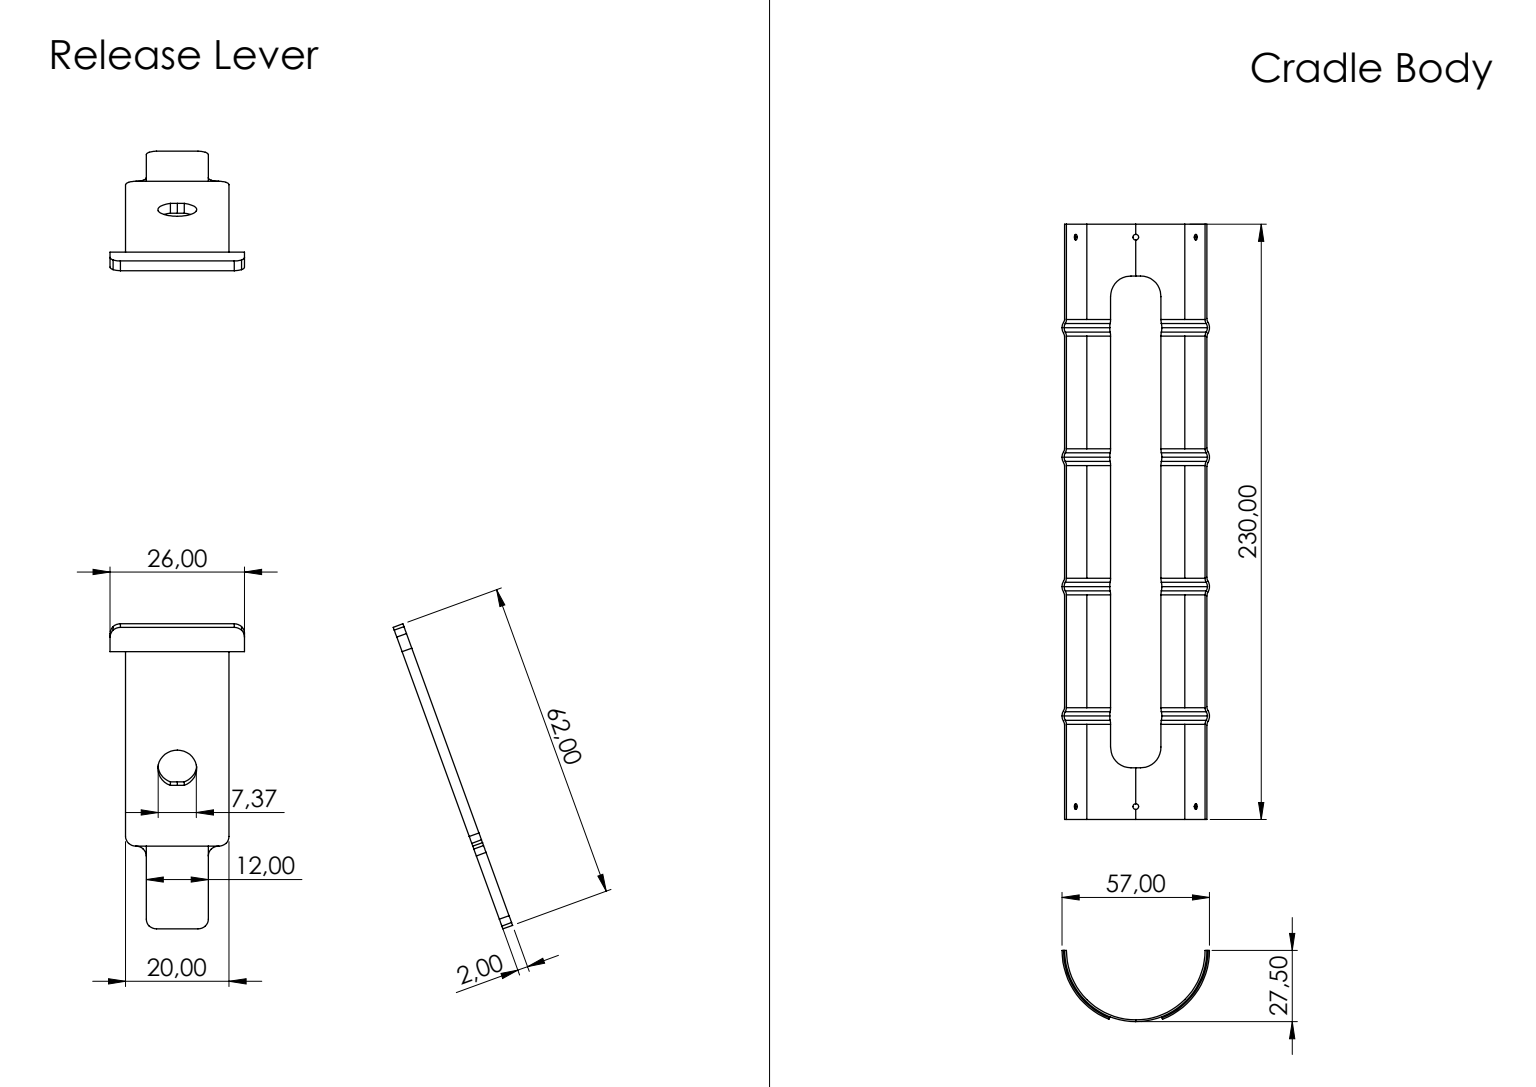
ISO-10303-21;
HEADER;
FILE_DESCRIPTION (('STEP AP214'),
    '1' );
FILE_NAME ('Cradle Body.step',
    '2026-10-06T09:00:30',
    ( '' ),
    ( '' ),
    'SwSTEP 2.0',
    'SolidWorks 2020',
    '' );
FILE_SCHEMA (( 'AUTOMOTIVE_DESIGN' ));
ENDSEC;

DATA;
#3=CARTESIAN_POINT ( 'NONE',  ( 27.50000000000000000, -6.735334946019999940E-15, 115.0000000000000000 ) ) ;
#7=B_SPLINE_CURVE_WITH_KNOTS ( 'NONE', 5,
 ( #8666, #18262, #27873, #6319, #23164, #13557 ),
 .UNSPECIFIED., .F., .F.,
 ( 6, 6 ),
 ( -2.319814965009999952, 0.000000000000000000 ),
 .UNSPECIFIED. ) ;
#21=ORIENTED_EDGE ( 'NONE', *, *, #30426, .T. ) ;
#35=AXIS2_PLACEMENT_3D ( 'NONE', #27512, #5959, #1254 ) ;
#45=ORIENTED_EDGE ( 'NONE', *, *, #3237, .T. ) ;
#75=CARTESIAN_POINT ( 'NONE',  ( 0.09701118263791908003, -27.50000000070000894, 6.100000000000011191 ) ) ;
#76=ORIENTED_EDGE ( 'NONE', *, *, #19659, .F. ) ;
#80=EDGE_CURVE ( 'NONE', #20682, #22430, #3324, .T. ) ;
#82=CARTESIAN_POINT ( 'NONE',  ( 7.105427357599999217E-15, 3.552713678799999608E-15, 43.21714158840000408 ) ) ;
#85=EDGE_LOOP ( 'NONE', ( #21526, #26943, #30310, #22481 ) ) ;
#87=CARTESIAN_POINT ( 'NONE',  ( 27.69999999930000101, -3.392159599989999961E-15, 90.00000000000000000 ) ) ;
#106=EDGE_CURVE ( 'NONE', #11838, #4649, #28678, .T. ) ;
#109=ORIENTED_EDGE ( 'NONE', *, *, #22749, .F. ) ;
#114=AXIS2_PLACEMENT_3D ( 'NONE', #11940, #28625, #12094 ) ;
#115=CARTESIAN_POINT ( 'NONE',  ( -3.552713678799999608E-15, 0.000000000000000000, 193.2171415880000040 ) ) ;
#128=DIRECTION ( 'NONE',  ( -0.000000000000000000, -0.000000000000000000, -1.000000000000000000 ) ) ;
#137=ORIENTED_EDGE ( 'NONE', *, *, #11511, .F. ) ;
#149=CARTESIAN_POINT ( 'NONE',  ( 0.4908581387334869928, -27.49541710664063032, 225.9948832293035537 ) ) ;
#160=ORIENTED_EDGE ( 'NONE', *, *, #26147, .F. ) ;
#162=FACE_BOUND ( 'NONE', #6310, .T. ) ;
#166=ORIENTED_EDGE ( 'NONE', *, *, #29617, .T. ) ;
#182=ORIENTED_EDGE ( 'NONE', *, *, #19559, .F. ) ;
#186=EDGE_CURVE ( 'NONE', #24695, #19740, #19204, .T. ) ;
#189=LINE ( 'NONE', #19380, #24692 ) ;
#190=CARTESIAN_POINT ( 'NONE',  ( 8.566424601805415762, -26.13212873426111216, 23.30748548239859019 ) ) ;
#192=AXIS2_PLACEMENT_3D ( 'NONE', #23801, #30571, #26003 ) ;
#202=EDGE_LOOP ( 'NONE', ( #3283, #15747, #28522, #14669, #12113 ) ) ;
#208=VECTOR ( 'NONE', #27934, 1000.000000000000114 ) ;
#210=CIRCLE ( 'NONE', #706, 27.69999999999999929 ) ;
#213=ORIENTED_EDGE ( 'NONE', *, *, #13656, .T. ) ;
#220=ADVANCED_FACE ( 'NONE', ( #19519 ), #21819, .T. ) ;
#224=EDGE_CURVE ( 'NONE', #17932, #4565, #12425, .T. ) ;
#228=CARTESIAN_POINT ( 'NONE',  ( 26.93395403039999891, -3.298349123909999533E-15, 87.75675929330000713 ) ) ;
#231=CARTESIAN_POINT ( 'NONE',  ( 22.70032920257776254, -14.24644155109503885, 5.491373161944450132 ) ) ;
#237=AXIS2_PLACEMENT_3D ( 'NONE', #28809, #7419, #7570 ) ;
#240=AXIS2_PLACEMENT_3D ( 'NONE', #28736, #7186, #4980 ) ;
#241=AXIS2_PLACEMENT_3D ( 'NONE', #12449, #26774, #973 ) ;
#243=AXIS2_PLACEMENT_3D ( 'NONE', #30286, #20689, #17993 ) ;
#255=EDGE_CURVE ( 'NONE', #7386, #15620, #13185, .T. ) ;
#264=DIRECTION ( 'NONE',  ( 0.000000000000000000, 0.000000000000000000, -1.000000000000000000 ) ) ;
#271=DIRECTION ( 'NONE',  ( 0.000000000000000000, 0.000000000000000000, 1.000000000000000000 ) ) ;
#276=CARTESIAN_POINT ( 'NONE',  ( 0.9565336475350260104, -27.48338672371320612, 4.451904520592202097 ) ) ;
#281=CARTESIAN_POINT ( 'NONE',  ( 8.903108651239925564, -22.82508830966962421, 140.0000000000000000 ) ) ;
#290=ORIENTED_EDGE ( 'NONE', *, *, #7961, .T. ) ;
#300=DIRECTION ( 'NONE',  ( -1.224606353819999829E-16, -1.000000000000000000, 0.000000000000000000 ) ) ;
#304=DIRECTION ( 'NONE',  ( 0.000000000000000000, 0.000000000000000000, 1.000000000000000000 ) ) ;
#312=CARTESIAN_POINT ( 'NONE',  ( 1.087768546295719840, -27.47890868157812605, 225.2179249496743978 ) ) ;
#314=CARTESIAN_POINT ( 'NONE',  ( 8.903108651239925564, -22.82508830966962421, 40.00000000000000000 ) ) ;
#317=DIRECTION ( 'NONE',  ( 0.9316362575375356503, 0.3633921898465274913, 0.000000000000000000 ) ) ;
#324=FACE_OUTER_BOUND ( 'NONE', #14055, .T. ) ;
#332=ORIENTED_EDGE ( 'NONE', *, *, #29953, .F. ) ;
#342=CARTESIAN_POINT ( 'NONE',  ( -23.20948082139999968, -13.40000000000000036, 6.099999999630000502 ) ) ;
#351=CARTESIAN_POINT ( 'NONE',  ( 8.414407093329970166, -26.18160851622837981, 23.09437632025412412 ) ) ;
#369=ORIENTED_EDGE ( 'NONE', *, *, #12352, .F. ) ;
#380=EDGE_CURVE ( 'NONE', #18294, #17040, #28347, .T. ) ;
#381=AXIS2_PLACEMENT_3D ( 'NONE', #29649, #27284, #22722 ) ;
#385=DIRECTION ( 'NONE',  ( 0.000000000000000000, 0.000000000000000000, 1.000000000000000000 ) ) ;
#387=CARTESIAN_POINT ( 'NONE',  ( 7.105427357599999217E-15, 3.552713678799999608E-15, 143.6055512749999821 ) ) ;
#390=CARTESIAN_POINT ( 'NONE',  ( 10.35667741062603397, -26.55163333981976592, 190.0000000000000000 ) ) ;
#399=DIRECTION ( 'NONE',  ( 0.000000000000000000, 0.000000000000000000, 1.000000000000000000 ) ) ;
#400=ORIENTED_EDGE ( 'NONE', *, *, #20390, .F. ) ;
#405=CIRCLE ( 'NONE', #17950, 27.23548387080000310 ) ;
#407=FACE_OUTER_BOUND ( 'NONE', #9123, .T. ) ;
#420=AXIS2_PLACEMENT_3D ( 'NONE', #11851, #7126, #19088 ) ;
#422=CARTESIAN_POINT ( 'NONE',  ( -27.92857142909999979, 3.420150602519999655E-15, 92.06031501479999690 ) ) ;
#427=CIRCLE ( 'NONE', #27022, 27.23548387080000310 ) ;
#428=DIRECTION ( 'NONE',  ( 0.3633921898465272138, -0.9316362575375356503, 0.000000000000000000 ) ) ;
#432=AXIS2_PLACEMENT_3D ( 'NONE', #11352, #25679, #6931 ) ;
#439=CARTESIAN_POINT ( 'NONE',  ( -24.33346004068414459, -12.81155130651161045, 5.286751411345756324 ) ) ;
#449=ORIENTED_EDGE ( 'NONE', *, *, #3492, .F. ) ;
#462=ORIENTED_EDGE ( 'NONE', *, *, #21169, .F. ) ;
#470=CARTESIAN_POINT ( 'NONE',  ( -3.907985046680000082E-14, -26.80000000000000071, 6.099999999630000502 ) ) ;
#471=DIRECTION ( 'NONE',  ( 1.000000000000000000, 0.000000000000000000, 0.000000000000000000 ) ) ;
#473=CARTESIAN_POINT ( 'NONE',  ( -27.50000000000000000, 3.367667473009999970E-15, 36.39444872359999295 ) ) ;
#474=CARTESIAN_POINT ( 'NONE',  ( 0.6479069288420113981, -26.79235980062891542, 224.0901877813894032 ) ) ;
#485=ORIENTED_EDGE ( 'NONE', *, *, #26372, .T. ) ;
#486=AXIS2_PLACEMENT_3D ( 'NONE', #21935, #385, #9970 ) ;
#489=ORIENTED_EDGE ( 'NONE', *, *, #26242, .T. ) ;
#498=DIRECTION ( 'NONE',  ( -0.7071067811865475727, -0.7071067811865475727, 0.000000000000000000 ) ) ;
#504=ADVANCED_FACE ( 'NONE', ( #24355, #2797 ), #16952, .T. ) ;
#505=CARTESIAN_POINT ( 'NONE',  ( 10.14902473058287491, -26.01926976374856082, 187.9396849849999853 ) ) ;
#513=ORIENTED_EDGE ( 'NONE', *, *, #26739, .T. ) ;
#515=CARTESIAN_POINT ( 'NONE',  ( -10.35667741062608371, -26.55163333981974816, 190.0000000000000000 ) ) ;
#521=DIRECTION ( 'NONE',  ( 1.000000000000000000, 0.000000000000000000, 0.000000000000000000 ) ) ;
#524=ORIENTED_EDGE ( 'NONE', *, *, #26123, .T. ) ;
#530=FACE_OUTER_BOUND ( 'NONE', #26990, .T. ) ;
#538=ORIENTED_EDGE ( 'NONE', *, *, #20624, .T. ) ;
#546=LINE ( 'NONE', #17194, #5634 ) ;
#547=DIRECTION ( 'NONE',  ( 0.000000000000000000, 0.000000000000000000, -1.000000000000000000 ) ) ;
#559=ORIENTED_EDGE ( 'NONE', *, *, #5058, .T. ) ;
#564=DIRECTION ( 'NONE',  ( 1.000000000000000000, 0.000000000000000000, 0.000000000000000000 ) ) ;
#568=DIRECTION ( 'NONE',  ( 1.000000000000000000, -1.224606353819999582E-16, 0.000000000000000000 ) ) ;
#569=AXIS2_PLACEMENT_3D ( 'NONE', #17547, #27158, #15193 ) ;
#570=CARTESIAN_POINT ( 'NONE',  ( -3.552713678799999608E-15, -26.80000000000000071, 0.000000000000000000 ) ) ;
#571=CARTESIAN_POINT ( 'NONE',  ( -23.92402432625451070, -13.56054118811422882, 3.912293197164086855 ) ) ;
#577=ORIENTED_EDGE ( 'NONE', *, *, #30008, .F. ) ;
#580=CARTESIAN_POINT ( 'NONE',  ( 24.49999999589999788, -3.000285566359999846E-15, 90.00000000000000000 ) ) ;
#583=CARTESIAN_POINT ( 'NONE',  ( 26.93395386830000149, -3.298349104060000254E-15, 142.2432411360000231 ) ) ;
#589=FACE_OUTER_BOUND ( 'NONE', #26163, .T. ) ;
#591=CARTESIAN_POINT ( 'NONE',  ( -22.29514036694591184, -14.89751301532327155, 93.21714158846667431 ) ) ;
#607=DIRECTION ( 'NONE',  ( 1.224606353819999829E-16, 1.000000000000000000, 0.000000000000000000 ) ) ;
#619=EDGE_CURVE ( 'NONE', #11656, #7142, #9529, .T. ) ;
#625=CARTESIAN_POINT ( 'NONE',  ( -26.84464183999999776, 3.287411896330000120E-15, 142.5624961750000068 ) ) ;
#637=ORIENTED_EDGE ( 'NONE', *, *, #4986, .T. ) ;
#640=ORIENTED_EDGE ( 'NONE', *, *, #8309, .F. ) ;
#660=CARTESIAN_POINT ( 'NONE',  ( 24.34663841809999951, -12.78636765230000094, 5.000000000000000000 ) ) ;
#667=DIRECTION ( 'NONE',  ( 0.3090169943750400994, -0.9510565162951234441, 0.000000000000000000 ) ) ;
#668=EDGE_CURVE ( 'NONE', #10071, #13694, #28108, .T. ) ;
#675=CARTESIAN_POINT ( 'NONE',  ( 27.50000000000000000, -1.044349611129999949E-13, 0.000000000000000000 ) ) ;
#677=EDGE_CURVE ( 'NONE', #10071, #14251, #16593, .T. ) ;
#679=DIRECTION ( 'NONE',  ( 0.9316362575375356503, 0.3633921898465274913, 0.000000000000000000 ) ) ;
#680=ORIENTED_EDGE ( 'NONE', *, *, #23014, .F. ) ;
#682=DIRECTION ( 'NONE',  ( 0.9316362575375356503, 0.3633921898465274913, 0.000000000000000000 ) ) ;
#684=CARTESIAN_POINT ( 'NONE',  ( 0.000000000000000000, 0.000000000000000000, 92.06031501460000754 ) ) ;
#685=CIRCLE ( 'NONE', #15728, 3.200000000000000178 ) ;
#688=MANIFOLD_SOLID_BREP ( 'Stock-MAS-156-1', #17562 ) ;
#691=TOROIDAL_SURFACE ( 'NONE', #8176, 29.80000000000000071, 3.000000000000000000 ) ;
#694=CARTESIAN_POINT ( 'NONE',  ( -0.2897532859572976571, -27.49881094958763939, 6.071390044457605661 ) ) ;
#695=CARTESIAN_POINT ( 'NONE',  ( 23.26185891380331583, -14.66761890373620503, 225.2867514118632357 ) ) ;
#706=AXIS2_PLACEMENT_3D ( 'NONE', #14476, #7537, #17129 ) ;
#708=CIRCLE ( 'NONE', #23295, 3.000000000000001332 ) ;
#709=CARTESIAN_POINT ( 'NONE',  ( 23.81569860410000317, -13.75000000000000000, 6.099999999630000502 ) ) ;
#717=LINE ( 'NONE', #17373, #10923 ) ;
#722=ORIENTED_EDGE ( 'NONE', *, *, #2189, .T. ) ;
#729=CIRCLE ( 'NONE', #20825, 27.50000000000000000 ) ;
#731=VECTOR ( 'NONE', #13088, 1000.000000000000114 ) ;
#733=CARTESIAN_POINT ( 'NONE',  ( 26.80000000069999899, -3.281945028320000125E-15, 142.8898184869999852 ) ) ;
#734=CARTESIAN_POINT ( 'NONE',  ( -5.851800771450323957, -26.15706768910720825, 208.9785434308453489 ) ) ;
#741=CARTESIAN_POINT ( 'NONE',  ( -7.833397470852288436, -25.63019328476619307, 22.68384840406914549 ) ) ;
#752=EDGE_CURVE ( 'NONE', #26248, #11846, #25282, .T. ) ;
#758=DIRECTION ( 'NONE',  ( 1.224606353819999829E-16, 1.000000000000000000, 0.000000000000000000 ) ) ;
#768=CARTESIAN_POINT ( 'NONE',  ( 20.19076655603537418, -17.71015691556361205, 86.78285841154168168 ) ) ;
#770=DIRECTION ( 'NONE',  ( 0.000000000000000000, 0.000000000000000000, 1.000000000000000000 ) ) ;
#774=CARTESIAN_POINT ( 'NONE',  ( 9.339631244007776445, -25.12005762863061165, 204.5931320852415354 ) ) ;
#783=DIRECTION ( 'NONE',  ( 0.7071067811865475727, 0.7071067811865475727, 0.000000000000000000 ) ) ;
#798=CYLINDRICAL_SURFACE ( 'NONE', #20779, 26.80000000000002203 ) ;
#799=CARTESIAN_POINT ( 'NONE',  ( -27.50000000000000000, 1.776356839399999804E-15, 43.60555127550000520 ) ) ;
#800=DIRECTION ( 'NONE',  ( 0.000000000000000000, 0.000000000000000000, 1.000000000000000000 ) ) ;
#807=CARTESIAN_POINT ( 'NONE',  ( 11.08346179031908640, -28.41490585489484033, 193.6055512750000105 ) ) ;
#813=CARTESIAN_POINT ( 'NONE',  ( -27.54391552379999908, 3.373045395949999841E-15, 92.95625301640001226 ) ) ;
#819=CARTESIAN_POINT ( 'NONE',  ( 0.000000000000000000, 0.000000000000000000, 90.00000000000000000 ) ) ;
#821=ORIENTED_EDGE ( 'NONE', *, *, #27749, .F. ) ;
#822=CARTESIAN_POINT ( 'NONE',  ( -0.8355101799141004815, -26.78702284090145014, 4.280685865825344827 ) ) ;
#839=CARTESIAN_POINT ( 'NONE',  ( 0.000000000000000000, -17.25771824150000100, 5.000000000000000000 ) ) ;
#840=EDGE_CURVE ( 'NONE', #23934, #21744, #20728, .T. ) ;
#842=CARTESIAN_POINT ( 'NONE',  ( 23.74292845531203966, -13.87604159492686939, 226.1000000000000512 ) ) ;
#846=EDGE_CURVE ( 'NONE', #15698, #27653, #3362, .T. ) ;
#859=SHAPE_REPRESENTATION_RELATIONSHIP ( 'NONE' , 'NONE' ,  #19621, #20057 ) ;
#863=ORIENTED_EDGE ( 'NONE', *, *, #7156, .T. ) ;
#871=ORIENTED_EDGE ( 'NONE', *, *, #27753, .F. ) ;
#873=CARTESIAN_POINT ( 'NONE',  ( 1.100000000000000089, -26.77741585740000119, 5.000000000000000000 ) ) ;
#875=ORIENTED_EDGE ( 'NONE', *, *, #15893, .F. ) ;
#876=CARTESIAN_POINT ( 'NONE',  ( 11.45957740435851235, -24.29669185712473478, 36.78285841129288514 ) ) ;
#885=CARTESIAN_POINT ( 'NONE',  ( 27.76135144349999706, -3.399672736829999707E-15, 142.3385858900000187 ) ) ;
#886=EDGE_CURVE ( 'NONE', #22309, #15300, #28972, .T. ) ;
#891=AXIS2_PLACEMENT_3D ( 'NONE', #15373, #6397, #3885 ) ;
#892=CARTESIAN_POINT ( 'NONE',  ( -19.36389667587701524, -18.53702679572193546, 93.21714158842225117 ) ) ;
#902=VERTEX_POINT ( 'NONE', #27140 ) ;
#903=CIRCLE ( 'NONE', #21011, 2.999999999999999556 ) ;
#906=ORIENTED_EDGE ( 'NONE', *, *, #846, .F. ) ;
#911=CIRCLE ( 'NONE', #3909, 4.000000000000001776 ) ;
#922=CARTESIAN_POINT ( 'NONE',  ( -27.92857142820000149, 1.776356839399999804E-15, 187.9396849849999853 ) ) ;
#927=CARTESIAN_POINT ( 'NONE',  ( 8.158046243928268382, -25.52871334855630536, 206.9076631228209635 ) ) ;
#930=CARTESIAN_POINT ( 'NONE',  ( 24.05715877135684622, -13.32261293554750914, 225.9948832293248415 ) ) ;
#942=ORIENTED_EDGE ( 'NONE', *, *, #4712, .F. ) ;
#947=EDGE_CURVE ( 'NONE', #18243, #19781, #29652, .T. ) ;
#958=VECTOR ( 'NONE', #5157, 1000.000000000000114 ) ;
#959=CARTESIAN_POINT ( 'NONE',  ( 0.000000000000000000, 0.000000000000000000, 115.0000000000000000 ) ) ;
#969=DIRECTION ( 'NONE',  ( 1.000000000000000000, 0.000000000000000000, 0.000000000000000000 ) ) ;
#970=LINE ( 'NONE', #17624, #2207 ) ;
#971=ORIENTED_EDGE ( 'NONE', *, *, #25154, .T. ) ;
#973=DIRECTION ( 'NONE',  ( -0.5000000000001898481, -0.8660254037843291286, 0.000000000000000000 ) ) ;
#975=CARTESIAN_POINT ( 'NONE',  ( -4.182178350032519809, -27.18131967880235322, 20.25455995680620447 ) ) ;
#976=ORIENTED_EDGE ( 'NONE', *, *, #14186, .T. ) ;
#981=EDGE_CURVE ( 'NONE', #18243, #12035, #20262, .T. ) ;
#988=CARTESIAN_POINT ( 'NONE',  ( -27.50000000000000000, 3.367667473009999970E-15, 186.3944487260000074 ) ) ;
#998=VECTOR ( 'NONE', #23561, 1000.000000000000000 ) ;
#999=AXIS2_PLACEMENT_3D ( 'NONE', #22838, #679, #10268 ) ;
#1000=CARTESIAN_POINT ( 'NONE',  ( 24.34660549313293032, -12.78643034496977116, 224.8543268302984188 ) ) ;
#1003=CARTESIAN_POINT ( 'NONE',  ( 23.76736455380283530, -13.83371703085023086, 223.8999999999988688 ) ) ;
#1004=ORIENTED_EDGE ( 'NONE', *, *, #677, .F. ) ;
#1025=CARTESIAN_POINT ( 'NONE',  ( 14.94562240850000023, -8.628859120750000500, 225.0000000000000000 ) ) ;
#1029=ORIENTED_EDGE ( 'NONE', *, *, #5957, .T. ) ;
#1031=CARTESIAN_POINT ( 'NONE',  ( -22.77466902118896996, -14.12660345815406338, 4.296357262948782285 ) ) ;
#1038=EDGE_LOOP ( 'NONE', ( #25052, #15396, #23007, #6576 ) ) ;
#1042=FACE_OUTER_BOUND ( 'NONE', #3125, .T. ) ;
#1048=ORIENTED_EDGE ( 'NONE', *, *, #17146, .F. ) ;
#1057=CARTESIAN_POINT ( 'NONE',  ( -23.73992238019999945, -12.43607998449999918, 225.0000000000000000 ) ) ;
#1067=CARTESIAN_POINT ( 'NONE',  ( 23.62133197435833409, -12.66014020633680914, 4.296357262547505940 ) ) ;
#1069=B_SPLINE_CURVE_WITH_KNOTS ( 'NONE', 3,
 ( #24794, #9698, #21667, #19302, #28895, #7344, #26539, #4979, #14590, #24178, #2618, #19455, #12210, #21822 ),
 .UNSPECIFIED., .F., .F.,
 ( 4, 2, 2, 2, 2, 2, 4 ),
 ( 0.000000000000000000, 0.2500000000000449640, 0.3750000000000674460, 0.4375000000000606182, 0.5000000000000538458, 0.7500000000000269784, 1.000000000000000000 ),
 .UNSPECIFIED. ) ;
#1070=CARTESIAN_POINT ( 'NONE',  ( -1.100000000000000089, -27.47799119300000115, 225.0000000000000000 ) ) ;
#1074=CARTESIAN_POINT ( 'NONE',  ( 7.662090775718879421, -25.68204763724676454, 207.5103208889252357 ) ) ;
#1077=CARTESIAN_POINT ( 'NONE',  ( 6.496986506900683800, -26.00150201275823392, 21.45239876629313258 ) ) ;
#1083=ORIENTED_EDGE ( 'NONE', *, *, #8304, .F. ) ;
#1088=EDGE_LOOP ( 'NONE', ( #13311, #8137, #3315, #26948, #18723, #26281, #19667, #6923, #6456, #7311, #3860, #7841, #18721, #26251, #1988, #26660, #13386, #29370, #11303, #12417, #30625, #13343, #13248, #22269, #29067, #21456, #29439, #26048, #28817, #4264, #9391, #19279, #17779, #17940, #28601, #166, #332, #23931, #19123, #1813, #6184, #27951, #18968, #5521 ) ) ;
#1092=CARTESIAN_POINT ( 'NONE',  ( -7.453090060300354480, -2.907137518772246576, 27.99999999999999645 ) ) ;
#1096=CARTESIAN_POINT ( 'NONE',  ( -7.453090060300356257, -2.907137518772246576, 20.00000000000000000 ) ) ;
#1110=CARTESIAN_POINT ( 'NONE',  ( 0.000000000000000000, 0.000000000000000000, 36.39444872359999295 ) ) ;
#1115=DIRECTION ( 'NONE',  ( 0.000000000000000000, 0.000000000000000000, 1.000000000000000000 ) ) ;
#1117=CARTESIAN_POINT ( 'NONE',  ( -22.63992238021892334, -14.34133587286723888, 224.9035646515725659 ) ) ;
#1119=ORIENTED_EDGE ( 'NONE', *, *, #21500, .T. ) ;
#1120=CARTESIAN_POINT ( 'NONE',  ( -0.1474957663552681764, -26.80000000000001492, 3.899999999999999911 ) ) ;
#1121=ORIENTED_EDGE ( 'NONE', *, *, #17384, .F. ) ;
#1131=CARTESIAN_POINT ( 'NONE',  ( 9.797681423453981964, -25.69548940455785413, 203.8387348960827694 ) ) ;
#1149=ORIENTED_EDGE ( 'NONE', *, *, #12119, .F. ) ;
#1158=CARTESIAN_POINT ( 'NONE',  ( 24.29812717139177636, -12.87956648213236832, 5.490554142100076085 ) ) ;
#1161=CARTESIAN_POINT ( 'NONE',  ( -8.903108651239966420, -22.82508830966961000, 140.0000000000000000 ) ) ;
#1163=EDGE_CURVE ( 'NONE', #16579, #13261, #16538, .T. ) ;
#1167=EDGE_CURVE ( 'NONE', #15899, #25472, #18720, .T. ) ;
#1168=B_SPLINE_CURVE_WITH_KNOTS ( 'NONE', 3,
 ( #26996, #12366, #24485, #2922, #12515, #29350, #5435, #3071, #734, #10325, #29505, #7942, #17542, #4831, #22437, #15497, #3534, #22594, #3375, #12981, #25101, #3227, #13445, #8397 ),
 .UNSPECIFIED., .F., .F.,
 ( 4, 2, 2, 2, 2, 2, 2, 2, 2, 2, 2, 4 ),
 ( 0.000000000000000000, 0.001577043753785914524, 0.002365565630678863329, 0.003154087507571812134, 0.004731131261357737934, 0.005519653138250699316, 0.006308175015143660698, 0.007885218768929582595, 0.009462262522715505358, 0.01025078439960847021, 0.01103930627650143333, 0.01261635003028735783 ),
 .UNSPECIFIED. ) ;
#1180=ORIENTED_EDGE ( 'NONE', *, *, #1838, .T. ) ;
#1182=CARTESIAN_POINT ( 'NONE',  ( -22.87891075612136760, -13.95728375031006685, 4.090187774257245223 ) ) ;
#1189=CARTESIAN_POINT ( 'NONE',  ( 22.63996212555145249, -14.34127312894895923, 224.8540320937674437 ) ) ;
#1206=EDGE_LOOP ( 'NONE', ( #7039, #213, #29911, #1121, #16764, #16573 ) ) ;
#1226=CARTESIAN_POINT ( 'NONE',  ( -9.993285220779425160, -25.61999708228226069, 136.3944487260000074 ) ) ;
#1231=CARTESIAN_POINT ( 'NONE',  ( 9.484767271962898150, -25.06561782275612771, 204.0863404859320553 ) ) ;
#1233=CARTESIAN_POINT ( 'NONE',  ( -24.90462872294775920, -9.900530325344874427, 43.21714158839293418 ) ) ;
#1234=AXIS2_PLACEMENT_3D ( 'NONE', #16237, #4129, #16086 ) ;
#1254=DIRECTION ( 'NONE',  ( 1.000000000000000000, -1.224606353819999829E-16, 0.000000000000000000 ) ) ;
#1264=DIRECTION ( 'NONE',  ( 0.3633921898465272138, -0.9316362575375356503, 1.850371707708593498E-14 ) ) ;
#1265=CARTESIAN_POINT ( 'NONE',  ( 3.552713678799999608E-15, -3.552713678799999608E-15, 136.7828584120000244 ) ) ;
#1276=CARTESIAN_POINT ( 'NONE',  ( -2.168672284410000206E-10, -27.14999999990000035, 0.000000000000000000 ) ) ;
#1278=DIRECTION ( 'NONE',  ( 1.000000000000000000, 0.000000000000000000, 0.000000000000000000 ) ) ;
#1279=CARTESIAN_POINT ( 'NONE',  ( -18.95046173579999760, -18.95046173579999760, -2.842170943039999687E-14 ) ) ;
#1282=ORIENTED_EDGE ( 'NONE', *, *, #21795, .F. ) ;
#1290=VERTEX_POINT ( 'NONE', #7385 ) ;
#1294=CARTESIAN_POINT ( 'NONE',  ( -23.26091398107482888, -13.42624119016083384, 0.000000000000000000 ) ) ;
#1296=DIRECTION ( 'NONE',  ( -1.000000000000000000, 1.224606353819999829E-16, 0.000000000000000000 ) ) ;
#1315=CARTESIAN_POINT ( 'NONE',  ( 26.80000000069999899, -3.281945028320000125E-15, 137.1101814800000227 ) ) ;
#1316=FACE_OUTER_BOUND ( 'NONE', #18611, .T. ) ;
#1318=DIRECTION ( 'NONE',  ( 0.000000000000000000, 0.000000000000000000, 1.000000000000000000 ) ) ;
#1324=CARTESIAN_POINT ( 'NONE',  ( 23.48807013373048491, -14.30280389787537842, 4.086914724217819206 ) ) ;
#1326=ADVANCED_FACE ( 'NONE', ( #162, #324 ), #9277, .F. ) ;
#1332=ADVANCED_FACE ( 'NONE', ( #18883 ), #6663, .T. ) ;
#1333=CYLINDRICAL_SURFACE ( 'NONE', #5437, 1.099999999999999867 ) ;
#1338=EDGE_LOOP ( 'NONE', ( #8212, #25635, #5309, #8348 ) ) ;
#1340=CARTESIAN_POINT ( 'NONE',  ( 18.95046173579999760, -18.95046173579999760, 115.0000000000000000 ) ) ;
#1343=CARTESIAN_POINT ( 'NONE',  ( 24.34663841809999951, -12.78636765230000094, 225.0000000000000000 ) ) ;
#1359=CARTESIAN_POINT ( 'NONE',  ( -18.95046173579999760, -18.95046173579999760, 115.0000000000000000 ) ) ;
#1374=EDGE_LOOP ( 'NONE', ( #18092, #3792, #29449, #21165 ) ) ;
#1375=CARTESIAN_POINT ( 'NONE',  ( 10.14902473071748368, -26.01926976409366077, 87.93968498540000667 ) ) ;
#1383=CIRCLE ( 'NONE', #7898, 27.50000000000000000 ) ;
#1389=CARTESIAN_POINT ( 'NONE',  ( 9.689803781819819051, -24.98716455116954549, 203.0573596598972017 ) ) ;
#1395=B_SPLINE_CURVE_WITH_KNOTS ( 'NONE', 5,
 ( #25094, #24937, #3063, #15177, #6041, #22267 ),
 .UNSPECIFIED., .F., .F.,
 ( 6, 6 ),
 ( -2.319814960280000005, 0.000000000000000000 ),
 .UNSPECIFIED. ) ;
#1402=AXIS2_PLACEMENT_3D ( 'NONE', #24745, #14997, #2153 ) ;
#1403=AXIS2_PLACEMENT_3D ( 'NONE', #15802, #3679, #8082 ) ;
#1405=ORIENTED_EDGE ( 'NONE', *, *, #3637, .F. ) ;
#1408=CARTESIAN_POINT ( 'NONE',  ( 7.105427357599999217E-15, 3.552713678799999608E-15, 93.60555127549999099 ) ) ;
#1411=CARTESIAN_POINT ( 'NONE',  ( -1.033595436889999888E-13, -27.50000000069999828, 3.899999999999999911 ) ) ;
#1416=EDGE_CURVE ( 'NONE', #27427, #6530, #20546, .T. ) ;
#1431=DIRECTION ( 'NONE',  ( 1.000000000000000000, -1.224606353820000075E-16, 0.000000000000000000 ) ) ;
#1433=CARTESIAN_POINT ( 'NONE',  ( -22.70120178296838986, -14.24511786445138206, 224.5052107108826647 ) ) ;
#1435=CARTESIAN_POINT ( 'NONE',  ( 0.8466631608419120658, -26.78674355063222734, 4.296357544259503669 ) ) ;
#1436=EDGE_LOOP ( 'NONE', ( #19200, #25509, #1669, #15010, #4840, #15096, #3053, #26439, #4768, #7960 ) ) ;
#1437=CARTESIAN_POINT ( 'NONE',  ( -9.738910687886987105, -24.96785170200594095, 143.2171415880000040 ) ) ;
#1441=ORIENTED_EDGE ( 'NONE', *, *, #10698, .F. ) ;
#1442=CARTESIAN_POINT ( 'NONE',  ( -3.552713678799999608E-15, -3.552713678799999608E-15, 141.6604601749999972 ) ) ;
#1452=ADVANCED_FACE ( 'NONE', ( #5755 ), #12994, .F. ) ;
#1453=CARTESIAN_POINT ( 'NONE',  ( 9.944225187684267553, -25.63929276476995156, 203.0591393848753512 ) ) ;
#1454=CARTESIAN_POINT ( 'NONE',  ( -21.30588112097817088, -16.35227051405537679, -0.000000000000000000 ) ) ;
#1459=CARTESIAN_POINT ( 'NONE',  ( -5.420768140797359358, -26.96154273974103077, 209.3135392056180706 ) ) ;
#1484=CARTESIAN_POINT ( 'NONE',  ( -23.25788685383076881, -13.43083806724688500, 186.7828584123333826 ) ) ;
#1486=ORIENTED_EDGE ( 'NONE', *, *, #27163, .T. ) ;
#1493=VERTEX_POINT ( 'NONE', #13937 ) ;
#1498=CARTESIAN_POINT ( 'NONE',  ( 25.43121960300669215, -8.635379644106567554, 136.7828584120000244 ) ) ;
#1502=CYLINDRICAL_SURFACE ( 'NONE', #243, 26.80000000000002203 ) ;
#1505=DIRECTION ( 'NONE',  ( 1.000000000000000000, 0.000000000000000000, 0.000000000000000000 ) ) ;
#1511=EDGE_CURVE ( 'NONE', #24890, #28814, #18024, .T. ) ;
#1520=DIRECTION ( 'NONE',  ( -0.000000000000000000, -0.000000000000000000, -1.000000000000000000 ) ) ;
#1526=VERTEX_POINT ( 'NONE', #5375 ) ;
#1529=CARTESIAN_POINT ( 'NONE',  ( -26.93395402219999824, 3.298349122909999612E-15, 187.7567592740000180 ) ) ;
#1540=DIRECTION ( 'NONE',  ( 0.000000000000000000, 0.000000000000000000, 1.000000000000000000 ) ) ;
#1544=CARTESIAN_POINT ( 'NONE',  ( -0.5569265645694643219, -27.49469370722579242, 225.9595466040883878 ) ) ;
#1548=CARTESIAN_POINT ( 'NONE',  ( -23.56630063302987921, -14.17280417044578655, 5.994883229690994852 ) ) ;
#1553=CARTESIAN_POINT ( 'NONE',  ( -1.100000000000000311, -27.47799119299999759, 224.9035402883650647 ) ) ;
#1563=EDGE_CURVE ( 'NONE', #7142, #20367, #26643, .T. ) ;
#1568=CIRCLE ( 'NONE', #4075, 27.49999999619999969 ) ;
#1569=DIRECTION ( 'NONE',  ( -0.3633921898465274913, 0.9316362575375356503, 0.000000000000000000 ) ) ;
#1571=DIRECTION ( 'NONE',  ( 0.000000000000000000, 0.000000000000000000, -1.000000000000000000 ) ) ;
#1579=CARTESIAN_POINT ( 'NONE',  ( -3.907985046680000082E-14, -26.80000000000000071, 6.099999999630000502 ) ) ;
#1586=EDGE_CURVE ( 'NONE', #22430, #26248, #13128, .T. ) ;
#1587=CARTESIAN_POINT ( 'NONE',  ( -27.92857142909999979, 3.420150602519999655E-15, 42.06031501480000401 ) ) ;
#1588=CIRCLE ( 'NONE', #28218, 27.50000000000000000 ) ;
#1596=EDGE_CURVE ( 'NONE', #6530, #7809, #10987, .T. ) ;
#1598=VERTEX_POINT ( 'NONE', #1437 ) ;
#1613=DIRECTION ( 'NONE',  ( 1.000000000000000000, 0.000000000000000000, 0.000000000000000000 ) ) ;
#1620=EDGE_CURVE ( 'NONE', #6179, #13261, #23694, .T. ) ;
#1633=EDGE_LOOP ( 'NONE', ( #13346, #45, #30897, #13735, #27902 ) ) ;
#1634=VERTEX_POINT ( 'NONE', #27695 ) ;
#1639=DIRECTION ( 'NONE',  ( 0.3633921898465273803, -0.9316362575375355393, -1.387778780781445044E-14 ) ) ;
#1643=CARTESIAN_POINT ( 'NONE',  ( -0.9560301558052189952, -26.78297054395609322, 224.4510318449164004 ) ) ;
#1648=FACE_OUTER_BOUND ( 'NONE', #26090, .T. ) ;
#1663=CARTESIAN_POINT ( 'NONE',  ( 9.993285220779439371, -25.61999708228226069, 27.99999999999999645 ) ) ;
#1669=ORIENTED_EDGE ( 'NONE', *, *, #31035, .T. ) ;
#1673=EDGE_LOOP ( 'NONE', ( #15667, #2741, #7837, #6105 ) ) ;
#1680=( LENGTH_UNIT ( ) NAMED_UNIT ( * ) SI_UNIT ( .MILLI., .METRE. ) );
#1706=ADVANCED_FACE ( 'NONE', ( #20781 ), #26066, .F. ) ;
#1708=AXIS2_PLACEMENT_3D ( 'NONE', #30537, #18565, #30994 ) ;
#1716=ORIENTED_EDGE ( 'NONE', *, *, #13633, .F. ) ;
#1718=DIRECTION ( 'NONE',  ( 0.000000000000000000, 0.000000000000000000, 1.000000000000000000 ) ) ;
#1721=DIRECTION ( 'NONE',  ( 0.000000000000000000, 0.000000000000000000, 1.000000000000000000 ) ) ;
#1730=CIRCLE ( 'NONE', #7253, 26.80000000000000071 ) ;
#1739=CARTESIAN_POINT ( 'NONE',  ( -2.947640775130000104E-14, -27.50000000000000000, 226.0999999999999943 ) ) ;
#1741=EDGE_CURVE ( 'NONE', #17533, #18378, #27065, .T. ) ;
#1742=EDGE_CURVE ( 'NONE', #10713, #24430, #2938, .T. ) ;
#1751=ORIENTED_EDGE ( 'NONE', *, *, #13656, .F. ) ;
#1756=CIRCLE ( 'NONE', #8768, 4.000000004070001225 ) ;
#1767=CARTESIAN_POINT ( 'NONE',  ( -26.80000000069999899, 3.281945028329999726E-15, 43.21714158909999526 ) ) ;
#1771=CARTESIAN_POINT ( 'NONE',  ( -8.566424601805399774, -26.13212873426111926, 206.6925145176014098 ) ) ;
#1780=CARTESIAN_POINT ( 'NONE',  ( -10.82908725742657019, -27.76276047461853835, 193.2171415880000040 ) ) ;
#1785=AXIS2_PLACEMENT_3D ( 'NONE', #27160, #27614, #10632 ) ;
#1793=ORIENTED_EDGE ( 'NONE', *, *, #25948, .F. ) ;
#1794=ORIENTED_EDGE ( 'NONE', *, *, #22467, .T. ) ;
#1802=B_SPLINE_CURVE_WITH_KNOTS ( 'NONE', 5,
 ( #3037, #26961, #3189, #22093, #5248, #3338 ),
 .UNSPECIFIED., .F., .F.,
 ( 6, 6 ),
 ( 0.000000000000000000, 2.319815199919999849 ),
 .UNSPECIFIED. ) ;
#1806=CARTESIAN_POINT ( 'NONE',  ( -23.73992238019999945, -12.43607998449999918, 5.000000000000000000 ) ) ;
#1808=CARTESIAN_POINT ( 'NONE',  ( -22.75759213010913484, -14.15424219528663130, 225.6766013745738348 ) ) ;
#1813=ORIENTED_EDGE ( 'NONE', *, *, #30225, .F. ) ;
#1814=CARTESIAN_POINT ( 'NONE',  ( -9.738910687886855655, -24.96785170200598714, 27.99999999999999645 ) ) ;
#1816=FACE_OUTER_BOUND ( 'NONE', #5552, .T. ) ;
#1824=DIRECTION ( 'NONE',  ( 0.9316362575375356503, 0.3633921898465274913, 0.000000000000000000 ) ) ;
#1827=CARTESIAN_POINT ( 'NONE',  ( -23.95771898018137236, -13.50170546705606789, 226.0719093208724075 ) ) ;
#1831=ORIENTED_EDGE ( 'NONE', *, *, #8892, .T. ) ;
#1832=DIRECTION ( 'NONE',  ( 0.9316362575375356503, 0.3633921898465274913, 0.000000000000000000 ) ) ;
#1838=EDGE_CURVE ( 'NONE', #4180, #4540, #6968, .T. ) ;
#1850=CARTESIAN_POINT ( 'NONE',  ( -0.2860395613546503069, -27.49884598709234496, 226.0719093208176673 ) ) ;
#1856=CARTESIAN_POINT ( 'NONE',  ( -24.34131725940281044, -12.79741914667978619, 224.7820750478432217 ) ) ;
#1857=ORIENTED_EDGE ( 'NONE', *, *, #6043, .F. ) ;
#1868=ORIENTED_EDGE ( 'NONE', *, *, #9506, .T. ) ;
#1870=CARTESIAN_POINT ( 'NONE',  ( -27.23548387100000312, 1.421085471519999843E-14, 91.66046017469999185 ) ) ;
#1883=CARTESIAN_POINT ( 'NONE',  ( -0.2196051096525505342, -26.79904497467719438, 6.087620938723986797 ) ) ;
#1902=ORIENTED_EDGE ( 'NONE', *, *, #16079, .T. ) ;
#1919=EDGE_CURVE ( 'NONE', #23553, #25078, #23536, .T. ) ;
#1924=LINE ( 'NONE', #30714, #27909 ) ;
#1929=DIRECTION ( 'NONE',  ( -0.9316362575375349842, 0.3633921898465292122, -0.000000000000000000 ) ) ;
#1945=EDGE_CURVE ( 'NONE', #24116, #11717, #903, .T. ) ;
#1947=ORIENTED_EDGE ( 'NONE', *, *, #186, .T. ) ;
#1950=CARTESIAN_POINT ( 'NONE',  ( 23.56630063294606714, -14.17280417058648467, 4.005116770382093350 ) ) ;
#1964=CARTESIAN_POINT ( 'NONE',  ( -9.738910687886981776, -24.96785170200593384, 193.2171415880000040 ) ) ;
#1974=CARTESIAN_POINT ( 'NONE',  ( 9.738910687886868089, -24.96785170200598358, 115.0000000000000000 ) ) ;
#1975=AXIS2_PLACEMENT_3D ( 'NONE', #17193, #24446, #16723 ) ;
#1982=EDGE_CURVE ( 'NONE', #27268, #21389, #15470, .T. ) ;
#1988=ORIENTED_EDGE ( 'NONE', *, *, #29277, .T. ) ;
#1991=ORIENTED_EDGE ( 'NONE', *, *, #13667, .F. ) ;
#2005=LINE ( 'NONE', #6708, #24844 ) ;
#2010=DIRECTION ( 'NONE',  ( -0.8090169943751909232, 0.5877852522921378498, 0.000000000000000000 ) ) ;
#2011=DIRECTION ( 'NONE',  ( 1.000000000000000000, 0.000000000000000000, 0.000000000000000000 ) ) ;
#2018=EDGE_CURVE ( 'NONE', #26248, #16461, #3994, .T. ) ;
#2019=CARTESIAN_POINT ( 'NONE',  ( -1.100000000000000089, -27.47799119300000115, 225.0000000000000000 ) ) ;
#2028=CARTESIAN_POINT ( 'NONE',  ( 0.000000000000000000, 0.000000000000000000, 190.0000000000000000 ) ) ;
#2031=CYLINDRICAL_SURFACE ( 'NONE', #9951, 26.80000000000002203 ) ;
#2061=TOROIDAL_SURFACE ( 'NONE', #7574, 29.80000000000000071, 3.000000000000000000 ) ;
#2074=EDGE_CURVE ( 'NONE', #13351, #2375, #5605, .T. ) ;
#2078=DIRECTION ( 'NONE',  ( 0.3633921898465272138, -0.9316362575375356503, 0.000000000000000000 ) ) ;
#2085=DIRECTION ( 'NONE',  ( 1.224606353819999829E-16, 1.000000000000000000, 0.000000000000000000 ) ) ;
#2098=VERTEX_POINT ( 'NONE', #27745 ) ;
#2112=CARTESIAN_POINT ( 'NONE',  ( -23.06578384684251048, -13.64653153747141801, 226.0721256962708878 ) ) ;
#2128=VECTOR ( 'NONE', #5783, 1000.000000000000000 ) ;
#2133=EDGE_CURVE ( 'NONE', #7727, #10044, #5912, .T. ) ;
#2138=CARTESIAN_POINT ( 'NONE',  ( 27.50000000000000000, -6.735334946019999940E-15, 36.39444872359999295 ) ) ;
#2153=DIRECTION ( 'NONE',  ( 0.3633921898465276024, -0.9316362575375355393, -3.469446951953614189E-14 ) ) ;
#2157=DIRECTION ( 'NONE',  ( 1.000000000000000000, 0.000000000000000000, 0.000000000000000000 ) ) ;
#2160=DIRECTION ( 'NONE',  ( 0.000000000000000000, 0.000000000000000000, -1.000000000000000000 ) ) ;
#2169=DIRECTION ( 'NONE',  ( 1.000000000000000000, 0.000000000000000000, 0.000000000000000000 ) ) ;
#2170=AXIS2_PLACEMENT_3D ( 'NONE', #11835, #13885, #19068 ) ;
#2172=DIRECTION ( 'NONE',  ( 0.000000000000000000, 0.000000000000000000, 1.000000000000000000 ) ) ;
#2189=EDGE_CURVE ( 'NONE', #8183, #12643, #7285, .T. ) ;
#2200=ADVANCED_FACE ( 'NONE', ( #19241 ), #16667, .T. ) ;
#2202=CARTESIAN_POINT ( 'NONE',  ( 27.92857142820000149, 1.776356839399999804E-15, 192.0603150150000147 ) ) ;
#2207=VECTOR ( 'NONE', #12915, 1000.000000000000114 ) ;
#2208=AXIS2_PLACEMENT_3D ( 'NONE', #25383, #5703, #20493 ) ;
#2217=EDGE_LOOP ( 'NONE', ( #23343, #25191, #17633, #24809, #15623, #4533 ) ) ;
#2230=AXIS2_PLACEMENT_3D ( 'NONE', #15972, #10626, #18001 ) ;
#2233=AXIS2_PLACEMENT_3D ( 'NONE', #21913, #12300, #29127 ) ;
#2235=B_SPLINE_CURVE_WITH_KNOTS ( 'NONE', 5,
 ( #16448, #30469, #21174, #11578, #18648, #2138 ),
 .UNSPECIFIED., .F., .F.,
 ( 6, 6 ),
 ( -2.300779731029999997, 0.000000000000000000 ),
 .UNSPECIFIED. ) ;
#2238=CIRCLE ( 'NONE', #19816, 27.50000000000000000 ) ;
#2249=VERTEX_POINT ( 'NONE', #14377 ) ;
#2251=CARTESIAN_POINT ( 'NONE',  ( 28.50000000000000000, -3.490128108379999702E-15, 190.0000000000000000 ) ) ;
#2260=AXIS2_PLACEMENT_3D ( 'NONE', #19061, #9302, #31021 ) ;
#2264=CARTESIAN_POINT ( 'NONE',  ( 26.80000000069999899, -3.281945028320000125E-15, 37.11018146769999504 ) ) ;
#2274=ORIENTED_EDGE ( 'NONE', *, *, #16284, .F. ) ;
#2290=FACE_OUTER_BOUND ( 'NONE', #6182, .T. ) ;
#2299=ORIENTED_EDGE ( 'NONE', *, *, #752, .F. ) ;
#2312=CARTESIAN_POINT ( 'NONE',  ( -2.813083154009999692E-14, -26.79999999949999889, 3.899999999999999911 ) ) ;
#2318=EDGE_CURVE ( 'NONE', #3529, #5952, #15658, .T. ) ;
#2339=EDGE_CURVE ( 'NONE', #17478, #24321, #19694, .T. ) ;
#2343=B_SPLINE_CURVE_WITH_KNOTS ( 'NONE', 3,
 ( #14729, #10007, #24323, #22271, #10320, #17080, #28888, #19605, #16923, #26680, #7338, #5286 ),
 .UNSPECIFIED., .F., .F.,
 ( 4, 2, 2, 2, 2, 4 ),
 ( 0.000000000000000000, 0.2499999999999773515, 0.3749999999999896749, 0.5000000000000019984, 0.7500000000000009992, 1.000000000000000000 ),
 .UNSPECIFIED. ) ;
#2349=ORIENTED_EDGE ( 'NONE', *, *, #1167, .T. ) ;
#2354=DIRECTION ( 'NONE',  ( -1.224606353819999829E-16, -1.000000000000000000, 0.000000000000000000 ) ) ;
#2355=ADVANCED_FACE ( 'NONE', ( #22224 ), #17490, .F. ) ;
#2372=ORIENTED_EDGE ( 'NONE', *, *, #6912, .F. ) ;
#2375=VERTEX_POINT ( 'NONE', #19713 ) ;
#2381=DIRECTION ( 'NONE',  ( 0.000000000000000000, 0.000000000000000000, -1.000000000000000000 ) ) ;
#2385=CARTESIAN_POINT ( 'NONE',  ( -27.23548386990000125, 3.335274659649999582E-15, 138.3395398259999922 ) ) ;
#2405=CARTESIAN_POINT ( 'NONE',  ( 18.95046173579999760, -18.95046173579999760, 43.21714158840000408 ) ) ;
#2407=ORIENTED_EDGE ( 'NONE', *, *, #7790, .F. ) ;
#2408=VERTEX_POINT ( 'NONE', #17181 ) ;
#2409=ORIENTED_EDGE ( 'NONE', *, *, #20417, .F. ) ;
#2411=FACE_OUTER_BOUND ( 'NONE', #12174, .T. ) ;
#2413=ADVANCED_FACE ( 'NONE', ( #530 ), #18170, .F. ) ;
#2418=AXIS2_PLACEMENT_3D ( 'NONE', #14565, #31084, #26819 ) ;
#2422=EDGE_LOOP ( 'NONE', ( #30105, #6247, #24854, #29914 ) ) ;
#2426=CARTESIAN_POINT ( 'NONE',  ( -27.76135144349999706, 3.399672736839999702E-15, 142.3385858900000187 ) ) ;
#2431=AXIS2_PLACEMENT_3D ( 'NONE', #27211, #9402, #20749 ) ;
#2454=AXIS2_PLACEMENT_3D ( 'NONE', #4821, #14417, #3027 ) ;
#2460=CIRCLE ( 'NONE', #29580, 26.80000000000000071 ) ;
#2462=ORIENTED_EDGE ( 'NONE', *, *, #1742, .T. ) ;
#2463=CARTESIAN_POINT ( 'NONE',  ( -26.84464183999999776, 3.287411896330000120E-15, 192.5624961750000068 ) ) ;
#2488=ORIENTED_EDGE ( 'NONE', *, *, #30930, .F. ) ;
#2491=ADVANCED_FACE ( 'NONE', ( #22681 ), #20621, .F. ) ;
#2504=AXIS2_PLACEMENT_3D ( 'NONE', #19203, #7396, #28789 ) ;
#2506=CARTESIAN_POINT ( 'NONE',  ( 0.000000000000000000, 0.000000000000000000, 20.00000000000000355 ) ) ;
#2507=DIRECTION ( 'NONE',  ( 0.000000000000000000, 1.000000000000000000, 0.000000000000000000 ) ) ;
#2509=EDGE_CURVE ( 'NONE', #5262, #15947, #26159, .T. ) ;
#2523=VERTEX_POINT ( 'NONE', #13824 ) ;
#2525=EDGE_LOOP ( 'NONE', ( #21481, #13778, #1991, #22145 ) ) ;
#2541=ADVANCED_FACE ( 'NONE', ( #3629 ), #4226, .F. ) ;
#2544=CARTESIAN_POINT ( 'NONE',  ( -23.30309534867867782, -14.60301215419051779, 225.4905541410415992 ) ) ;
#2545=CARTESIAN_POINT ( 'NONE',  ( 5.420768140797370016, -26.96154273974102367, 20.68646079438196139 ) ) ;
#2555=DIRECTION ( 'NONE',  ( 1.000000000000000000, 0.000000000000000000, 0.000000000000000000 ) ) ;
#2556=DIRECTION ( 'NONE',  ( 0.000000000000000000, 0.000000000000000000, -1.000000000000000000 ) ) ;
#2557=ORIENTED_EDGE ( 'NONE', *, *, #20470, .F. ) ;
#2565=ORIENTED_EDGE ( 'NONE', *, *, #25565, .T. ) ;
#2572=CARTESIAN_POINT ( 'NONE',  ( 9.738910687886868089, -24.96785170200598358, 115.0000000000000000 ) ) ;
#2578=CARTESIAN_POINT ( 'NONE',  ( 27.50000000000000000, -1.044349611129999949E-13, 0.000000000000000000 ) ) ;
#2582=ADVANCED_FACE ( 'NONE', ( #21995 ), #16795, .F. ) ;
#2584=CARTESIAN_POINT ( 'NONE',  ( -10.06596365874885812, -25.80632433378972124, 140.0000000000000000 ) ) ;
#2596=B_SPLINE_CURVE_WITH_KNOTS ( 'NONE', 3,
 ( #3576, #12711, #1389, #22320, #1231, #774, #29549, #7983, #13021, #17583, #927, #5630, #1074, #15230, #25303, #8290, #17885, #3267, #12874, #10518, #20418, #29705, #8133, #17730, #27489, #15536 ),
 .UNSPECIFIED., .F., .F.,
 ( 4, 2, 2, 2, 2, 2, 2, 2, 2, 2, 2, 2, 4 ),
 ( 0.000000000000000000, 0.001576840078853157653, 0.002365260118279736805, 0.003153680157706315306, 0.004730520236559471008, 0.005518940275986051677, 0.006307360315412630612, 0.007884200394265785880, 0.008672620433692339662, 0.009461040473118895178, 0.01024946051254545069, 0.01103788055197200621, 0.01261472063082510163 ),
 .UNSPECIFIED. ) ;
#2612=CIRCLE ( 'NONE', #19689, 28.50000000000000000 ) ;
#2618=CARTESIAN_POINT ( 'NONE',  ( -0.4946807615411580872, -26.79522487540722153, 225.9931951744256367 ) ) ;
#2624=DIRECTION ( 'NONE',  ( 1.000000000000000000, 0.000000000000000000, 0.000000000000000000 ) ) ;
#2625=EDGE_LOOP ( 'NONE', ( #31017, #27334, #3846, #5304 ) ) ;
#2627=CARTESIAN_POINT ( 'NONE',  ( 0.000000000000000000, 0.000000000000000000, 0.000000000000000000 ) ) ;
#2628=ORIENTED_EDGE ( 'NONE', *, *, #23222, .F. ) ;
#2629=B_SPLINE_CURVE_WITH_KNOTS ( 'NONE', 3,
 ( #24631, #876, #26678, #12663, #22270, #5582 ),
 .UNSPECIFIED., .F., .F.,
 ( 4, 2, 4 ),
 ( 0.4735259726301723759, 0.7367629863150860769, 1.000000000000000000 ),
 .UNSPECIFIED. ) ;
#2631=AXIS2_PLACEMENT_3D ( 'NONE', #7709, #14813, #14506 ) ;
#2650=CARTESIAN_POINT ( 'NONE',  ( 14.39562240800000126, -9.581487064249998298, 225.0000000000000000 ) ) ;
#2656=CARTESIAN_POINT ( 'NONE',  ( 18.95046173579999760, -18.95046173579999760, 115.0000000000000000 ) ) ;
#2660=EDGE_CURVE ( 'NONE', #24695, #14421, #12575, .T. ) ;
#2670=ORIENTED_EDGE ( 'NONE', *, *, #30110, .T. ) ;
#2683=CARTESIAN_POINT ( 'NONE',  ( -22.86188831003414634, -13.98516151716066069, 5.876648809228268711 ) ) ;
#2694=AXIS2_PLACEMENT_3D ( 'NONE', #3038, #4942, #9822 ) ;
#2710=EDGE_LOOP ( 'NONE', ( #24883, #16294, #14538, #25977, #13641, #20747 ) ) ;
#2731=FACE_OUTER_BOUND ( 'NONE', #20312, .T. ) ;
#2741=ORIENTED_EDGE ( 'NONE', *, *, #981, .F. ) ;
#2744=VECTOR ( 'NONE', #2556, 1000.000000000000000 ) ;
#2748=EDGE_LOOP ( 'NONE', ( #26366, #21675, #28485, #19199, #18414 ) ) ;
#2749=DIRECTION ( 'NONE',  ( 0.000000000000000000, 0.000000000000000000, -1.000000000000000000 ) ) ;
#2768=ORIENTED_EDGE ( 'NONE', *, *, #18659, .T. ) ;
#2778=DIRECTION ( 'NONE',  ( -0.8660254037843289066, -0.5000000000001899592, 0.000000000000000000 ) ) ;
#2779=CIRCLE ( 'NONE', #9807, 4.000000004070001225 ) ;
#2784=DIRECTION ( 'NONE',  ( 0.000000000000000000, 0.000000000000000000, -1.000000000000000000 ) ) ;
#2786=CARTESIAN_POINT ( 'NONE',  ( 27.69999999930000101, -3.392159599989999961E-15, 190.0000000000000000 ) ) ;
#2797=FACE_OUTER_BOUND ( 'NONE', #26703, .T. ) ;
#2809=FACE_OUTER_BOUND ( 'NONE', #6045, .T. ) ;
#2824=VERTEX_POINT ( 'NONE', #570 ) ;
#2825=ORIENTED_EDGE ( 'NONE', *, *, #24311, .F. ) ;
#2832=CYLINDRICAL_SURFACE ( 'NONE', #24536, 26.80000000000002203 ) ;
#2835=FACE_OUTER_BOUND ( 'NONE', #10954, .T. ) ;
#2840=B_SPLINE_CURVE_WITH_KNOTS ( 'NONE', 5,
 ( #7941, #733, #3225, #583, #12980, #12833 ),
 .UNSPECIFIED., .F., .F.,
 ( 6, 6 ),
 ( 0.000000000000000000, 2.319815200139999867 ),
 .UNSPECIFIED. ) ;
#2845=CARTESIAN_POINT ( 'NONE',  ( -23.34643930348659069, -14.53345043296637584, 225.6425104786826239 ) ) ;
#2846=CARTESIAN_POINT ( 'NONE',  ( 18.95046173579999760, -18.95046173579999760, 36.78285841159999592 ) ) ;
#2858=CARTESIAN_POINT ( 'NONE',  ( -10.14902473063359523, -26.01926976387844093, 142.0603150149999863 ) ) ;
#2875=ORIENTED_EDGE ( 'NONE', *, *, #24409, .T. ) ;
#2880=TOROIDAL_SURFACE ( 'NONE', #25505, 30.50000000000000000, 3.000000000000000000 ) ;
#2889=ORIENTED_EDGE ( 'NONE', *, *, #6189, .F. ) ;
#2900=ORIENTED_EDGE ( 'NONE', *, *, #23789, .F. ) ;
#2922=CARTESIAN_POINT ( 'NONE',  ( -3.664716979113584738, -26.54951320538905435, 209.8067551132096469 ) ) ;
#2934=EDGE_CURVE ( 'NONE', #4374, #6881, #14629, .T. ) ;
#2938=CIRCLE ( 'NONE', #13495, 4.000000000000001776 ) ;
#2941=ORIENTED_EDGE ( 'NONE', *, *, #26796, .T. ) ;
#2954=ORIENTED_EDGE ( 'NONE', *, *, #15780, .F. ) ;
#2968=CARTESIAN_POINT ( 'NONE',  ( 0.9003585010983619075, -26.78512143669438572, 224.3665129619594154 ) ) ;
#2977=ORIENTED_EDGE ( 'NONE', *, *, #13679, .F. ) ;
#2984=ORIENTED_EDGE ( 'NONE', *, *, #7926, .T. ) ;
#2985=B_SPLINE_CURVE_WITH_KNOTS ( 'NONE', 3,
 ( #8256, #15503, #17398, #3080, #29356, #19774, #22445, #17548, #8101, #22133, #27159, #741, #15355, #7801, #8844, #24953, #29671, #10333, #27004, #15195, #25109, #15052, #6491, #24799, #3385, #5442 ),
 .UNSPECIFIED., .F., .F.,
 ( 4, 2, 2, 2, 2, 2, 2, 2, 2, 2, 2, 2, 4 ),
 ( 0.000000000000000000, 0.001576840078853145944, 0.002365260118279718590, 0.003153680157706291454, 0.004730520236559437181, 0.005518940275986006574, 0.006307360315412575101, 0.007884200394265702613, 0.008672620433692270273, 0.009461040473118836197, 0.01024946051254540386, 0.01103788055197197152, 0.01261472063082510336 ),
 .UNSPECIFIED. ) ;
#2990=TOROIDAL_SURFACE ( 'NONE', #17049, 24.50000000000000000, 3.200000000000000178 ) ;
#2995=ORIENTED_EDGE ( 'NONE', *, *, #4104, .T. ) ;
#3001=CARTESIAN_POINT ( 'NONE',  ( -23.70578532293623653, -13.93854223005088677, 226.0877068035740365 ) ) ;
#3024=AXIS2_PLACEMENT_3D ( 'NONE', #24862, #17303, #22189 ) ;
#3027=DIRECTION ( 'NONE',  ( 0.3633921898465291567, 0.9316362575375349842, 0.000000000000000000 ) ) ;
#3028=EDGE_CURVE ( 'NONE', #21131, #24086, #21614, .T. ) ;
#3032=CARTESIAN_POINT ( 'NONE',  ( -0.9895645760634798060, -27.48220350681653557, 5.485672168196345844 ) ) ;
#3035=AXIS2_PLACEMENT_3D ( 'NONE', #2028, #23438, #23591 ) ;
#3037=CARTESIAN_POINT ( 'NONE',  ( 26.80000000000000071, -3.552713678799999608E-15, 193.2171415880000040 ) ) ;
#3038=CARTESIAN_POINT ( 'NONE',  ( -27.50000000000000000, 3.367667473009999970E-15, 0.000000000000000000 ) ) ;
#3049=CARTESIAN_POINT ( 'NONE',  ( 24.34131725955728598, -12.79741914641014411, 5.217924950592947475 ) ) ;
#3053=ORIENTED_EDGE ( 'NONE', *, *, #10857, .T. ) ;
#3057=DIRECTION ( 'NONE',  ( 0.000000000000000000, 0.000000000000000000, 1.000000000000000000 ) ) ;
#3063=CARTESIAN_POINT ( 'NONE',  ( -26.93395387809999875, 3.298349105260000080E-15, 42.24324102359999955 ) ) ;
#3064=CARTESIAN_POINT ( 'NONE',  ( 23.24663841809999809, -14.69162354060000020, 5.000000000000000000 ) ) ;
#3066=DIRECTION ( 'NONE',  ( -1.000000000000000000, 5.665498452320000818E-16, 0.000000000000000000 ) ) ;
#3071=CARTESIAN_POINT ( 'NONE',  ( -5.395560604220499101, -26.25584002662961680, 209.2195618656424756 ) ) ;
#3074=CARTESIAN_POINT ( 'NONE',  ( 1.100000000000000089, -27.47799119230000287, 5.000000000000000000 ) ) ;
#3080=CARTESIAN_POINT ( 'NONE',  ( -9.544994065185523624, -25.04267878452547080, 26.16927719407518538 ) ) ;
#3081=CARTESIAN_POINT ( 'NONE',  ( 26.80000000069999899, -3.281945028320000125E-15, 65.00000000000000000 ) ) ;
#3094=CARTESIAN_POINT ( 'NONE',  ( -23.70218820198384080, -12.50899637883967053, 225.4229804101834986 ) ) ;
#3095=DIRECTION ( 'NONE',  ( 1.000000000000000000, 0.000000000000000000, 0.000000000000000000 ) ) ;
#3101=VERTEX_POINT ( 'NONE', #16878 ) ;
#3109=CARTESIAN_POINT ( 'NONE',  ( 25.94284618478187809, -6.948772836044536660, 86.78285841113334698 ) ) ;
#3117=CARTESIAN_POINT ( 'NONE',  ( 9.738910687886866313, -24.96785170200598714, 27.46685764687258313 ) ) ;
#3122=LINE ( 'NONE', #13178, #24819 ) ;
#3125=EDGE_LOOP ( 'NONE', ( #20310, #17564, #15234, #8392 ) ) ;
#3133=CARTESIAN_POINT ( 'NONE',  ( -1.033595436889999888E-13, -27.50000000069999828, 3.899999999999999911 ) ) ;
#3135=EDGE_CURVE ( 'NONE', #25355, #10318, #12027, .T. ) ;
#3140=AXIS2_PLACEMENT_3D ( 'NONE', #14395, #21162, #18948 ) ;
#3141=CARTESIAN_POINT ( 'NONE',  ( -9.993285220779425160, -25.61999708228226069, 86.39444872359999295 ) ) ;
#3154=EDGE_LOOP ( 'NONE', ( #4420, #4293, #16099, #4034, #3458, #24419 ) ) ;
#3158=CARTESIAN_POINT ( 'NONE',  ( 3.466821295769682159E-14, -2.890242878314739659E-13, 27.99999999999999645 ) ) ;
#3159=FACE_OUTER_BOUND ( 'NONE', #2217, .T. ) ;
#3161=CARTESIAN_POINT ( 'NONE',  ( -9.944225187684255118, -25.63929276476996222, 26.94086061512460262 ) ) ;
#3167=DIRECTION ( 'NONE',  ( 1.000000000000000000, 0.000000000000000000, 0.000000000000000000 ) ) ;
#3168=CARTESIAN_POINT ( 'NONE',  ( -24.49999999470000134, 3.000285566209999917E-15, 89.99999999930000172 ) ) ;
#3174=ADVANCED_FACE ( 'NONE', ( #26638 ), #14686, .F. ) ;
#3175=CARTESIAN_POINT ( 'NONE',  ( 8.416763499243900881, -26.18199973230927924, 206.9245629863210354 ) ) ;
#3184=CARTESIAN_POINT ( 'NONE',  ( -0.5621952391521564119, -27.49459032466129926, 5.956950222287991537 ) ) ;
#3186=CARTESIAN_POINT ( 'NONE',  ( 23.53263993711012603, -14.22965940713208255, 225.9595466040883878 ) ) ;
#3189=CARTESIAN_POINT ( 'NONE',  ( 26.84464183999999776, -3.287411896319999731E-15, 192.5624961750000068 ) ) ;
#3203=CARTESIAN_POINT ( 'NONE',  ( 24.34663841808528417, -12.78636765232546146, 5.096459711759587563 ) ) ;
#3206=DIRECTION ( 'NONE',  ( -0.9316362575375349842, 0.3633921898465292122, -0.000000000000000000 ) ) ;
#3216=CARTESIAN_POINT ( 'NONE',  ( 0.9560301513573733478, -26.78297054411803302, 5.548968163149520905 ) ) ;
#3225=CARTESIAN_POINT ( 'NONE',  ( 26.84464183999999776, -3.287411896319999731E-15, 142.5624961750000068 ) ) ;
#3226=VECTOR ( 'NONE', #17718, 1000.000000000000114 ) ;
#3227=CARTESIAN_POINT ( 'NONE',  ( -9.689804814931735066, -24.98716964724290435, 203.0596100955893633 ) ) ;
#3233=CARTESIAN_POINT ( 'NONE',  ( -25.38111185550166127, -8.615767840674495304, 93.21714158837185948 ) ) ;
#3236=ORIENTED_EDGE ( 'NONE', *, *, #29708, .T. ) ;
#3237=EDGE_CURVE ( 'NONE', #24657, #12069, #7987, .T. ) ;
#3244=CIRCLE ( 'NONE', #8770, 27.92857142840000151 ) ;
#3251=CARTESIAN_POINT ( 'NONE',  ( -23.62009186240247161, -12.66256056379310202, 225.7119260798266396 ) ) ;
#3252=CARTESIAN_POINT ( 'NONE',  ( -24.08872333959828893, -11.87645233066225714, 143.2171415880000040 ) ) ;
#3255=AXIS2_PLACEMENT_3D ( 'NONE', #28296, #8786, #11777 ) ;
#3266=CARTESIAN_POINT ( 'NONE',  ( -23.73992238019999945, -12.43607998449999918, 5.000000000000000000 ) ) ;
#3267=CARTESIAN_POINT ( 'NONE',  ( 5.393907605749510559, -26.25263145716209578, 209.2056843174096628 ) ) ;
#3272=CARTESIAN_POINT ( 'NONE',  ( 6.706468900734747329, -25.94814536837671071, 21.60853380882830166 ) ) ;
#3283=ORIENTED_EDGE ( 'NONE', *, *, #7708, .F. ) ;
#3291=EDGE_CURVE ( 'NONE', #20382, #16822, #4991, .T. ) ;
#3294=DIRECTION ( 'NONE',  ( -1.000000000000000000, 5.665498452320000818E-16, 0.000000000000000000 ) ) ;
#3299=CARTESIAN_POINT ( 'NONE',  ( 23.20948082139999968, -13.40000000000000036, 6.099999999630000502 ) ) ;
#3300=CARTESIAN_POINT ( 'NONE',  ( 1.841797396446240631, -26.73663745407121795, 210.0000000000000284 ) ) ;
#3301=DIRECTION ( 'NONE',  ( 0.000000000000000000, 0.000000000000000000, 1.000000000000000000 ) ) ;
#3304=CARTESIAN_POINT ( 'NONE',  ( 22.88229166380642354, -13.95171381546676947, 225.9137588013241498 ) ) ;
#3305=DIRECTION ( 'NONE',  ( 0.000000000000000000, 0.000000000000000000, 1.000000000000000000 ) ) ;
#3315=ORIENTED_EDGE ( 'NONE', *, *, #7267, .T. ) ;
#3316=CARTESIAN_POINT ( 'NONE',  ( -0.9891024240349816088, -26.78175548724776434, 4.513394068097407619 ) ) ;
#3318=ADVANCED_FACE ( 'NONE', ( #25366 ), #8504, .F. ) ;
#3319=ORIENTED_EDGE ( 'NONE', *, *, #14351, .T. ) ;
#3320=ORIENTED_EDGE ( 'NONE', *, *, #26123, .F. ) ;
#3324=LINE ( 'NONE', #9445, #7067 ) ;
#3326=CARTESIAN_POINT ( 'NONE',  ( 0.000000000000000000, 0.000000000000000000, 187.9396849849999853 ) ) ;
#3327=CARTESIAN_POINT ( 'NONE',  ( 0.000000000000000000, 0.000000000000000000, 190.0000000000000000 ) ) ;
#3328=CARTESIAN_POINT ( 'NONE',  ( -10.14902473071754940, -26.01926976409365722, 37.93968498539999956 ) ) ;
#3336=CARTESIAN_POINT ( 'NONE',  ( 3.466821295769682159E-14, -2.890242878314739659E-13, 202.0000000000000000 ) ) ;
#3338=CARTESIAN_POINT ( 'NONE',  ( 27.23548386990000125, -3.335274659639999982E-15, 191.6604601740000078 ) ) ;
#3340=DIRECTION ( 'NONE',  ( 1.000000000000000000, 0.000000000000000000, 0.000000000000000000 ) ) ;
#3351=ORIENTED_EDGE ( 'NONE', *, *, #19785, .F. ) ;
#3353=FILL_AREA_STYLE_COLOUR ( '', #10763 ) ;
#3354=ORIENTED_EDGE ( 'NONE', *, *, #4559, .F. ) ;
#3358=DIRECTION ( 'NONE',  ( -1.000000000000000000, 1.224606353819999829E-16, 0.000000000000000000 ) ) ;
#3361=DIRECTION ( 'NONE',  ( -1.000000000000000000, 5.665498452320000818E-16, 0.000000000000000000 ) ) ;
#3362=CIRCLE ( 'NONE', #22472, 3.000000000000001332 ) ;
#3367=CARTESIAN_POINT ( 'NONE',  ( 0.8355090702542746772, -26.78702287552522066, 5.719315397085198427 ) ) ;
#3375=CARTESIAN_POINT ( 'NONE',  ( -9.335826947264916242, -25.12147279754469764, 204.6049336590874077 ) ) ;
#3379=CARTESIAN_POINT ( 'NONE',  ( 23.20948082139999968, -13.40000000000000036, 223.8999999999999773 ) ) ;
#3380=ORIENTED_EDGE ( 'NONE', *, *, #19127, .T. ) ;
#3384=TOROIDAL_SURFACE ( 'NONE', #5875, 30.50000000000000000, 3.000000000000000000 ) ;
#3385=CARTESIAN_POINT ( 'NONE',  ( -2.373622499810734698, -26.70000180411621216, 20.00000000000000711 ) ) ;
#3395=ORIENTED_EDGE ( 'NONE', *, *, #1563, .F. ) ;
#3405=CIRCLE ( 'NONE', #5921, 3.200000000000000178 ) ;
#3410=CARTESIAN_POINT ( 'NONE',  ( 27.76135143710000008, -3.399672736040000081E-15, 137.6614141009999912 ) ) ;
#3411=EDGE_CURVE ( 'NONE', #27268, #15558, #21084, .T. ) ;
#3413=CARTESIAN_POINT ( 'NONE',  ( 23.65805500388735183, -12.59178324494503265, 4.402070808934393398 ) ) ;
#3420=CARTESIAN_POINT ( 'NONE',  ( 0.000000000000000000, 0.000000000000000000, 90.00000000000000000 ) ) ;
#3436=CARTESIAN_POINT ( 'NONE',  ( -2.664535259099999568E-14, -26.80000000000000071, 115.0000000000000000 ) ) ;
#3438=VECTOR ( 'NONE', #1296, 1000.000000000000000 ) ;
#3458=ORIENTED_EDGE ( 'NONE', *, *, #18856, .T. ) ;
#3465=FACE_OUTER_BOUND ( 'NONE', #10035, .T. ) ;
#3467=CARTESIAN_POINT ( 'NONE',  ( -9.590600648852301902, -25.77356060526425097, 25.39622571667640472 ) ) ;
#3470=EDGE_CURVE ( 'NONE', #29399, #17667, #20609, .T. ) ;
#3474=AXIS2_PLACEMENT_3D ( 'NONE', #27872, #6153, #4112 ) ;
#3482=DIRECTION ( 'NONE',  ( 0.000000000000000000, 0.000000000000000000, -1.000000000000000000 ) ) ;
#3483=CARTESIAN_POINT ( 'NONE',  ( 26.84464185210000053, -3.287411897800000213E-15, 187.4375040470000044 ) ) ;
#3491=CARTESIAN_POINT ( 'NONE',  ( -23.24663841809999809, -14.69162354060000020, 225.0000000000000000 ) ) ;
#3492=EDGE_CURVE ( 'NONE', #11151, #13582, #23142, .T. ) ;
#3499=ORIENTED_EDGE ( 'NONE', *, *, #19706, .F. ) ;
#3511=DIRECTION ( 'NONE',  ( 0.3633921898465292122, 0.9316362575375348731, -6.938893903907226800E-15 ) ) ;
#3512=CARTESIAN_POINT ( 'NONE',  ( 3.552713678799999608E-15, -3.552713678799999608E-15, 186.7828584120000244 ) ) ;
#3517=EDGE_CURVE ( 'NONE', #11838, #3686, #5653, .T. ) ;
#3525=DIRECTION ( 'NONE',  ( 1.224606353819999829E-16, 1.000000000000000000, 0.000000000000000000 ) ) ;
#3527=ADVANCED_FACE ( 'NONE', ( #10081 ), #4040, .T. ) ;
#3529=VERTEX_POINT ( 'NONE', #29416 ) ;
#3531=DIRECTION ( 'NONE',  ( 0.3633921898465272138, -0.9316362575375356503, 2.312964634635741872E-15 ) ) ;
#3534=CARTESIAN_POINT ( 'NONE',  ( -8.964607010186835367, -25.25702356185616537, 205.5800510650676927 ) ) ;
#3543=CARTESIAN_POINT ( 'NONE',  ( -27.23548387180000319, 3.335274659879999868E-15, 88.33953982590000464 ) ) ;
#3559=CARTESIAN_POINT ( 'NONE',  ( -23.73992238018677980, -12.43607998452291774, 225.0964353478398436 ) ) ;
#3561=CARTESIAN_POINT ( 'NONE',  ( -26.80000000069999899, 3.281945028329999726E-15, 65.00000000000000000 ) ) ;
#3565=ORIENTED_EDGE ( 'NONE', *, *, #24311, .T. ) ;
#3572=CARTESIAN_POINT ( 'NONE',  ( -27.50000000000000000, 3.367667473009999970E-15, 186.7190980919999959 ) ) ;
#3576=CARTESIAN_POINT ( 'NONE',  ( 9.738910687886868089, -24.96785170200598358, 202.0000000000000000 ) ) ;
#3578=CARTESIAN_POINT ( 'NONE',  ( -26.11394584979203870, -6.088596733047853427, 43.21714158835001030 ) ) ;
#3582=VERTEX_POINT ( 'NONE', #24700 ) ;
#3595=CARTESIAN_POINT ( 'NONE',  ( -0.9007122707567293274, -27.48548889902986048, 4.367019785660003706 ) ) ;
#3598=DIRECTION ( 'NONE',  ( -0.3633921898465273803, 0.9316362575375355393, 0.000000000000000000 ) ) ;
#3608=AXIS2_PLACEMENT_3D ( 'NONE', #22628, #770, #24676 ) ;
#3618=ORIENTED_EDGE ( 'NONE', *, *, #30018, .T. ) ;
#3629=FACE_OUTER_BOUND ( 'NONE', #2710, .T. ) ;
#3637=EDGE_CURVE ( 'NONE', #10144, #15285, #6113, .T. ) ;
#3655=ORIENTED_EDGE ( 'NONE', *, *, #20172, .T. ) ;
#3660=CARTESIAN_POINT ( 'NONE',  ( 26.62724484483131349, -3.508068424019962883, 186.7828584120000244 ) ) ;
#3664=ORIENTED_EDGE ( 'NONE', *, *, #22554, .F. ) ;
#3665=CARTESIAN_POINT ( 'NONE',  ( -26.62724484483131704, -3.508068424019966880, 186.7828584128332920 ) ) ;
#3670=ADVANCED_FACE ( 'NONE', ( #25799 ), #27829, .T. ) ;
#3675=DIRECTION ( 'NONE',  ( -3.103340825716225161E-16, 1.008336558399225884E-16, 1.000000000000000000 ) ) ;
#3678=CARTESIAN_POINT ( 'NONE',  ( -23.62133197417733754, -12.66014020671418372, 5.703642737970564092 ) ) ;
#3679=DIRECTION ( 'NONE',  ( 0.000000000000000000, 0.000000000000000000, 1.000000000000000000 ) ) ;
#3683=CARTESIAN_POINT ( 'NONE',  ( 18.95046173579999760, -18.95046173579999760, 186.7828584120000244 ) ) ;
#3684=EDGE_CURVE ( 'NONE', #14251, #3529, #27152, .T. ) ;
#3686=VERTEX_POINT ( 'NONE', #30519 ) ;
#3688=CARTESIAN_POINT ( 'NONE',  ( -23.16094352436829240, -13.48406906362809998, 3.900000000003496670 ) ) ;
#3691=DIRECTION ( 'NONE',  ( 0.000000000000000000, 0.000000000000000000, 1.000000000000000000 ) ) ;
#3694=CARTESIAN_POINT ( 'NONE',  ( 23.13685276771313326, -13.52579547908016622, 223.9000000000000057 ) ) ;
#3704=EDGE_CURVE ( 'NONE', #18212, #13864, #19114, .T. ) ;
#3715=TOROIDAL_SURFACE ( 'NONE', #9237, 30.50000000000000000, 3.000000000000000000 ) ;
#3719=DIRECTION ( 'NONE',  ( 0.000000000000000000, 0.000000000000000000, 1.000000000000000000 ) ) ;
#3741=CARTESIAN_POINT ( 'NONE',  ( -1.421085471519999843E-14, -1.421085471519999843E-14, 86.39444872449999480 ) ) ;
#3745=AXIS2_PLACEMENT_3D ( 'NONE', #22899, #24788, #12978 ) ;
#3746=CARTESIAN_POINT ( 'NONE',  ( 9.335826947264928677, -25.12147279754469764, 25.39506634091258164 ) ) ;
#3758=VERTEX_POINT ( 'NONE', #9408 ) ;
#3759=ORIENTED_EDGE ( 'NONE', *, *, #16635, .F. ) ;
#3764=CARTESIAN_POINT ( 'NONE',  ( -0.2195863013093272698, -27.49906791309031462, 3.912356533825281257 ) ) ;
#3765=CARTESIAN_POINT ( 'NONE',  ( 27.63177371540000138, -3.383804565919999808E-15, 92.63947604839999883 ) ) ;
#3768=FACE_OUTER_BOUND ( 'NONE', #23895, .T. ) ;
#3769=AXIS2_PLACEMENT_3D ( 'NONE', #819, #7576, #10409 ) ;
#3770=ORIENTED_EDGE ( 'NONE', *, *, #17978, .F. ) ;
#3778=EDGE_CURVE ( 'NONE', #17932, #15300, #24638, .T. ) ;
#3788=ORIENTED_EDGE ( 'NONE', *, *, #4297, .T. ) ;
#3789=CARTESIAN_POINT ( 'NONE',  ( -22.64684861875350563, -14.33122899593499611, 224.7819332085316830 ) ) ;
#3792=ORIENTED_EDGE ( 'NONE', *, *, #25781, .F. ) ;
#3805=CARTESIAN_POINT ( 'NONE',  ( 9.506387914194320388, -25.80482363264563972, 204.8513626972847135 ) ) ;
#3807=CARTESIAN_POINT ( 'NONE',  ( 26.80000000069999899, -3.281945028320000125E-15, 186.7828584129999854 ) ) ;
#3825=CARTESIAN_POINT ( 'NONE',  ( -17.64448518804790567, -20.25643828355106990, 36.78285841153859081 ) ) ;
#3837=CARTESIAN_POINT ( 'NONE',  ( 0.000000000000000000, 0.000000000000000000, 190.0000000000000000 ) ) ;
#3842=B_SPLINE_CURVE_WITH_KNOTS ( 'NONE', 3,
 ( #14661, #14508, #12593, #2544, #2845, #24104, #26461, #3001, #12130, #31025 ),
 .UNSPECIFIED., .F., .F.,
 ( 4, 2, 2, 2, 4 ),
 ( 0.000000000000000000, 0.2500000000000000000, 0.5000000000000000000, 0.7500000000000000000, 1.000000000000000000 ),
 .UNSPECIFIED. ) ;
#3846=ORIENTED_EDGE ( 'NONE', *, *, #29825, .F. ) ;
#3852=CARTESIAN_POINT ( 'NONE',  ( -23.09885119212171389, -13.58970608817446823, 3.912379060515961626 ) ) ;
#3855=CARTESIAN_POINT ( 'NONE',  ( 9.993285220779439371, -25.61999708228226424, 27.46709065302605168 ) ) ;
#3860=ORIENTED_EDGE ( 'NONE', *, *, #14976, .T. ) ;
#3865=ADVANCED_FACE ( 'NONE', ( #5808 ), #15707, .T. ) ;
#3876=EDGE_LOOP ( 'NONE', ( #30607, #14615, #9443, #30664 ) ) ;
#3880=( NAMED_UNIT ( * ) PLANE_ANGLE_UNIT ( ) SI_UNIT ( $, .RADIAN. ) );
#3885=DIRECTION ( 'NONE',  ( -0.5000000000001894040, 0.8660254037843291286, 0.000000000000000000 ) ) ;
#3889=LINE ( 'NONE', #16003, #28859 ) ;
#3891=CIRCLE ( 'NONE', #17446, 2.999999999999999556 ) ;
#3895=CARTESIAN_POINT ( 'NONE',  ( 7.105427357599999217E-15, 3.552713678799999608E-15, 143.6055512749999821 ) ) ;
#3898=ADVANCED_FACE ( 'NONE', ( #5958 ), #15880, .F. ) ;
#3899=B_SPLINE_CURVE_WITH_KNOTS ( 'NONE', 3,
 ( #7160, #3203, #3049, #1158, #22252, #22569, #12641, #15019, #22715, #709 ),
 .UNSPECIFIED., .F., .F.,
 ( 4, 2, 2, 2, 4 ),
 ( 0.000000000000000000, 0.2500000000000000000, 0.5000000000000000000, 0.7500000000000000000, 1.000000000000000000 ),
 .UNSPECIFIED. ) ;
#3903=CARTESIAN_POINT ( 'NONE',  ( -24.29812717103635933, -12.87956648275837779, 224.5094458564340698 ) ) ;
#3909=AXIS2_PLACEMENT_3D ( 'NONE', #19589, #22105, #9834 ) ;
#3916=DIRECTION ( 'NONE',  ( 0.9316362575375356503, 0.3633921898465274913, 0.000000000000000000 ) ) ;
#3918=CARTESIAN_POINT ( 'NONE',  ( 0.000000000000000000, 0.000000000000000000, 115.0000000000000000 ) ) ;
#3919=CARTESIAN_POINT ( 'NONE',  ( -0.9877995808046760029, -27.48272658602412477, 4.509012502174277515 ) ) ;
#3921=FACE_OUTER_BOUND ( 'NONE', #27237, .T. ) ;
#3932=CARTESIAN_POINT ( 'NONE',  ( -0.8178280313492310993, -26.78758467680351174, 5.737227010353648460 ) ) ;
#3937=CARTESIAN_POINT ( 'NONE',  ( 23.09961856918545919, -13.58841269902310778, 226.0876905688013494 ) ) ;
#3941=CARTESIAN_POINT ( 'NONE',  ( -18.95046173579999760, -18.95046173579999760, 93.21714158839999698 ) ) ;
#3954=AXIS2_PLACEMENT_3D ( 'NONE', #3512, #17370, #564 ) ;
#3958=CIRCLE ( 'NONE', #17030, 2.999999999999999556 ) ;
#3960=CARTESIAN_POINT ( 'NONE',  ( 23.54244930488480136, -12.80639529643277008, 5.876648809236738380 ) ) ;
#3965=CARTESIAN_POINT ( 'NONE',  ( -9.739400760072916441, -25.71769950840797847, 204.0853438175687984 ) ) ;
#3974=CARTESIAN_POINT ( 'NONE',  ( 23.81569860410000317, -13.75000000000000000, 223.8999999999999773 ) ) ;
#3983=CARTESIAN_POINT ( 'NONE',  ( 0.000000000000000000, 0.000000000000000000, 192.0603150150000147 ) ) ;
#3987=EDGE_CURVE ( 'NONE', #5609, #30396, #9930, .T. ) ;
#3990=FACE_OUTER_BOUND ( 'NONE', #21797, .T. ) ;
#3993=DIRECTION ( 'NONE',  ( 0.000000000000000000, 0.000000000000000000, 1.000000000000000000 ) ) ;
#3994=LINE ( 'NONE', #20834, #11459 ) ;
#4000=CARTESIAN_POINT ( 'NONE',  ( -23.68794489818531446, -12.53584098786471479, 5.491373161348172438 ) ) ;
#4006=LINE ( 'NONE', #27922, #12813 ) ;
#4007=ORIENTED_EDGE ( 'NONE', *, *, #4030, .T. ) ;
#4010=DIRECTION ( 'NONE',  ( 0.9316362575375356503, 0.3633921898465274913, 0.000000000000000000 ) ) ;
#4030=EDGE_CURVE ( 'NONE', #19354, #4261, #24504, .T. ) ;
#4034=ORIENTED_EDGE ( 'NONE', *, *, #27403, .F. ) ;
#4036=CARTESIAN_POINT ( 'NONE',  ( -9.993285220779425160, -25.61999708228226069, 115.0000000000000000 ) ) ;
#4037=CARTESIAN_POINT ( 'NONE',  ( 9.738910687886932038, -24.96785170200595161, 143.2171415880000040 ) ) ;
#4040=TOROIDAL_SURFACE ( 'NONE', #11077, 29.80000000000000071, 3.000000000000000000 ) ;
#4052=CARTESIAN_POINT ( 'NONE',  ( -0.6750190883921094454, -27.49190635772141889, 225.8804910023025343 ) ) ;
#4056=ADVANCED_FACE ( 'NONE', ( #18544 ), #18336, .T. ) ;
#4075=AXIS2_PLACEMENT_3D ( 'NONE', #11971, #14183, #30865 ) ;
#4084=LINE ( 'NONE', #22971, #8706 ) ;
#4092=DIRECTION ( 'NONE',  ( 0.000000000000000000, 1.000000000000000000, 0.000000000000000000 ) ) ;
#4099=DIRECTION ( 'NONE',  ( 0.000000000000000000, 0.000000000000000000, 1.000000000000000000 ) ) ;
#4104=EDGE_CURVE ( 'NONE', #3529, #10318, #17323, .T. ) ;
#4112=DIRECTION ( 'NONE',  ( 0.7071067811865475727, 0.7071067811865475727, 0.000000000000000000 ) ) ;
#4114=CARTESIAN_POINT ( 'NONE',  ( 23.67274795607547233, -12.56353887348194220, 5.548968161597096937 ) ) ;
#4115=CARTESIAN_POINT ( 'NONE',  ( 27.50000000000000000, 1.776356839399999804E-15, 186.3944487249999895 ) ) ;
#4117=TOROIDAL_SURFACE ( 'NONE', #21709, 24.50000000000000000, 3.200000000000000178 ) ;
#4121=CARTESIAN_POINT ( 'NONE',  ( -9.944224317832761173, -25.63928765730900139, 203.0568480260882041 ) ) ;
#4123=CARTESIAN_POINT ( 'NONE',  ( -23.73992238019999945, -12.43607998449999918, 225.0000000000000000 ) ) ;
#4127=CARTESIAN_POINT ( 'NONE',  ( 23.88846875288458804, -13.62395840498221844, 223.8999999999999773 ) ) ;
#4129=DIRECTION ( 'NONE',  ( 0.000000000000000000, 0.000000000000000000, 1.000000000000000000 ) ) ;
#4130=ORIENTED_EDGE ( 'NONE', *, *, #2509, .F. ) ;
#4151=CARTESIAN_POINT ( 'NONE',  ( 23.30309534860585075, -14.60301215431637800, 4.509445859277517066 ) ) ;
#4159=VERTEX_POINT ( 'NONE', #29070 ) ;
#4160=CARTESIAN_POINT ( 'NONE',  ( -22.92720033282126124, -13.87810118031797835, 225.9606284813543482 ) ) ;
#4162=CARTESIAN_POINT ( 'NONE',  ( 26.80000000000001492, -1.754055898254314183, 136.7828584120000244 ) ) ;
#4174=ORIENTED_EDGE ( 'NONE', *, *, #17484, .T. ) ;
#4175=CARTESIAN_POINT ( 'NONE',  ( 10.82908725742652223, -27.76276047461856678, 136.7828584120000244 ) ) ;
#4178=DIRECTION ( 'NONE',  ( 0.3633921898465291567, 0.9316362575375349842, 0.000000000000000000 ) ) ;
#4179=CARTESIAN_POINT ( 'NONE',  ( -24.24391315703382688, -12.98049462792616815, 225.6749683491732981 ) ) ;
#4180=VERTEX_POINT ( 'NONE', #21851 ) ;
#4197=CARTESIAN_POINT ( 'NONE',  ( 0.6805609736260925802, -26.79155681409072898, 225.8766488246017730 ) ) ;
#4205=DIRECTION ( 'NONE',  ( 0.000000000000000000, 0.000000000000000000, 1.000000000000000000 ) ) ;
#4216=ORIENTED_EDGE ( 'NONE', *, *, #3684, .F. ) ;
#4217=EDGE_CURVE ( 'NONE', #18284, #12444, #22763, .T. ) ;
#4219=CIRCLE ( 'NONE', #24298, 3.199999983039998774 ) ;
#4226=PLANE ( 'NONE',  #16600 ) ;
#4232=DIRECTION ( 'NONE',  ( -0.9316362575375349842, 0.3633921898465292122, -0.000000000000000000 ) ) ;
#4238=CYLINDRICAL_SURFACE ( 'NONE', #4947, 26.80000000000002203 ) ;
#4245=AXIS2_PLACEMENT_3D ( 'NONE', #11752, #21359, #9381 ) ;
#4253=CARTESIAN_POINT ( 'NONE',  ( -23.20948082139999968, -13.40000000000000036, 3.900000000369999942 ) ) ;
#4261=VERTEX_POINT ( 'NONE', #25285 ) ;
#4264=ORIENTED_EDGE ( 'NONE', *, *, #15641, .F. ) ;
#4269=TOROIDAL_SURFACE ( 'NONE', #14319, 30.50000000000000000, 3.000000000000000000 ) ;
#4284=AXIS2_PLACEMENT_3D ( 'NONE', #12197, #4656, #22116 ) ;
#4286=CARTESIAN_POINT ( 'NONE',  ( -7.105427357599999217E-15, -7.105427357599999217E-15, 38.33953982530000104 ) ) ;
#4288=CARTESIAN_POINT ( 'NONE',  ( -10.82908725742658440, -27.76276047461855256, 136.7828584120000244 ) ) ;
#4293=ORIENTED_EDGE ( 'NONE', *, *, #2074, .T. ) ;
#4297=EDGE_CURVE ( 'NONE', #29399, #11656, #16336, .T. ) ;
#4300=EDGE_LOOP ( 'NONE', ( #4935, #20342, #20788, #6591, #30107, #25804, #13080, #30734, #5799, #21523, #21182, #27574, #2954, #27727, #26444, #5802, #15071, #20481, #871, #15393, #21291, #28606, #1793, #8776, #11064, #971, #19175, #3351, #16677, #29558, #4953, #18099, #3664, #2977, #19896, #27432, #27891, #13604, #5453, #27234, #22171, #8121, #5191, #15132 ) ) ;
#4302=DIRECTION ( 'NONE',  ( 1.000000000000000000, 0.000000000000000000, 0.000000000000000000 ) ) ;
#4304=ORIENTED_EDGE ( 'NONE', *, *, #25948, .T. ) ;
#4311=CARTESIAN_POINT ( 'NONE',  ( 23.76736455406628323, -13.83371703039393630, 3.899999999998877698 ) ) ;
#4322=DIRECTION ( 'NONE',  ( 0.3090169943750400994, -0.9510565162951234441, 0.000000000000000000 ) ) ;
#4325=CARTESIAN_POINT ( 'NONE',  ( 18.95046173579999760, -18.95046173579999760, 93.21714158839999698 ) ) ;
#4329=CARTESIAN_POINT ( 'NONE',  ( -23.74292845509082994, -13.87604159531000647, 3.900000000370010600 ) ) ;
#4344=EDGE_LOOP ( 'NONE', ( #19120, #1180, #8088, #14127 ) ) ;
#4349=CARTESIAN_POINT ( 'NONE',  ( -26.80000000069999899, 3.281945028329999726E-15, 187.1101814799999943 ) ) ;
#4350=DIRECTION ( 'NONE',  ( 1.000000000000000000, -1.224606353819998843E-16, 0.000000000000000000 ) ) ;
#4353=DIRECTION ( 'NONE',  ( 0.3633921898465272138, -0.9316362575375356503, -1.387778780781445044E-14 ) ) ;
#4366=LINE ( 'NONE', #23581, #16283 ) ;
#4374=VERTEX_POINT ( 'NONE', #4823 ) ;
#4379=ORIENTED_EDGE ( 'NONE', *, *, #18564, .F. ) ;
#4385=CIRCLE ( 'NONE', #23495, 26.80000000000000071 ) ;
#4395=CARTESIAN_POINT ( 'NONE',  ( -0.9242233315478671773, -26.78436826004146099, 5.597929193123646563 ) ) ;
#4415=ORIENTED_EDGE ( 'NONE', *, *, #22749, .T. ) ;
#4420=ORIENTED_EDGE ( 'NONE', *, *, #23196, .T. ) ;
#4422=DIRECTION ( 'NONE',  ( -0.3633921898465291012, -0.9316362575375348731, 0.000000000000000000 ) ) ;
#4435=CARTESIAN_POINT ( 'NONE',  ( 0.000000000000000000, 0.000000000000000000, 115.0000000000000000 ) ) ;
#4437=CARTESIAN_POINT ( 'NONE',  ( 23.72659769746557501, -12.46160974971369662, 225.2878164648903976 ) ) ;
#4445=FACE_OUTER_BOUND ( 'NONE', #85, .T. ) ;
#4457=EDGE_LOOP ( 'NONE', ( #13837, #3655, #13267, #11541, #22881 ) ) ;
#4464=EDGE_CURVE ( 'NONE', #24086, #7025, #12321, .T. ) ;
#4468=CARTESIAN_POINT ( 'NONE',  ( 2.168672284410000206E-10, -27.14999999990000035, 230.0000000000000000 ) ) ;
#4475=CARTESIAN_POINT ( 'NONE',  ( 23.25788685383077592, -13.43083806724684948, 136.7828584119999960 ) ) ;
#4484=AXIS2_PLACEMENT_3D ( 'NONE', #16654, #2354, #12092 ) ;
#4497=EDGE_CURVE ( 'NONE', #11846, #18237, #28383, .T. ) ;
#4498=B_SPLINE_CURVE_WITH_KNOTS ( 'NONE', 5,
 ( #28048, #12843, #10485, #20081, #12989, #3543 ),
 .UNSPECIFIED., .F., .F.,
 ( 6, 6 ),
 ( -2.319814892689999741, 0.000000000000000000 ),
 .UNSPECIFIED. ) ;
#4504=EDGE_CURVE ( 'NONE', #16579, #21098, #14196, .T. ) ;
#4507=DIRECTION ( 'NONE',  ( 0.000000000000000000, 0.000000000000000000, 1.000000000000000000 ) ) ;
#4524=CIRCLE ( 'NONE', #999, 3.200000000000000178 ) ;
#4533=ORIENTED_EDGE ( 'NONE', *, *, #16774, .F. ) ;
#4537=CARTESIAN_POINT ( 'NONE',  ( -24.49999999470000134, 3.000285566209999917E-15, 40.00000000070000539 ) ) ;
#4540=VERTEX_POINT ( 'NONE', #3683 ) ;
#4559=EDGE_CURVE ( 'NONE', #16212, #17178, #2779, .T. ) ;
#4565=VERTEX_POINT ( 'NONE', #8390 ) ;
#4570=DIRECTION ( 'NONE',  ( -0.3633921898465274913, 0.9316362575375356503, 0.000000000000000000 ) ) ;
#4578=CARTESIAN_POINT ( 'NONE',  ( -22.75778669576351732, -14.15360906368043281, 5.666076084815538927 ) ) ;
#4588=CIRCLE ( 'NONE', #8100, 27.69999999999999929 ) ;
#4593=EDGE_CURVE ( 'NONE', #17040, #12444, #1395, .T. ) ;
#4594=ORIENTED_EDGE ( 'NONE', *, *, #26202, .F. ) ;
#4614=AXIS2_PLACEMENT_3D ( 'NONE', #8039, #27246, #24896 ) ;
#4622=CARTESIAN_POINT ( 'NONE',  ( 1.100000000000000533, -27.47799119229999931, 5.097016884910053669 ) ) ;
#4623=ORIENTED_EDGE ( 'NONE', *, *, #619, .T. ) ;
#4639=EDGE_CURVE ( 'NONE', #8738, #27983, #15328, .T. ) ;
#4649=VERTEX_POINT ( 'NONE', #1964 ) ;
#4656=DIRECTION ( 'NONE',  ( 0.000000000000000000, 0.000000000000000000, 1.000000000000000000 ) ) ;
#4659=VERTEX_POINT ( 'NONE', #21153 ) ;
#4660=CARTESIAN_POINT ( 'NONE',  ( -2.107992564109736122, -27.41908764619381245, 210.0000000000000284 ) ) ;
#4661=CARTESIAN_POINT ( 'NONE',  ( 1.100000000000000089, -26.77741585740000119, 225.0000000000000000 ) ) ;
#4664=B_SPLINE_CURVE_WITH_KNOTS ( 'NONE', 5,
 ( #20883, #18971, #30483, #28578, #16302, #18657 ),
 .UNSPECIFIED., .F., .F.,
 ( 6, 6 ),
 ( -2.300779653589999807, 0.000000000000000000 ),
 .UNSPECIFIED. ) ;
#4671=EDGE_CURVE ( 'NONE', #28783, #13152, #4006, .T. ) ;
#4672=CARTESIAN_POINT ( 'NONE',  ( -24.34660549313268163, -12.78643034497024367, 5.145673169883069775 ) ) ;
#4678=EDGE_CURVE ( 'NONE', #2824, #10568, #30410, .T. ) ;
#4689=AXIS2_PLACEMENT_3D ( 'NONE', #387, #547, #5243 ) ;
#4690=CARTESIAN_POINT ( 'NONE',  ( -18.95046173579999760, -18.95046173579999760, 193.2171415880000040 ) ) ;
#4697=CIRCLE ( 'NONE', #12729, 27.69999999999999929 ) ;
#4699=VERTEX_POINT ( 'NONE', #30750 ) ;
#4712=EDGE_CURVE ( 'NONE', #22821, #15775, #7446, .T. ) ;
#4716=CARTESIAN_POINT ( 'NONE',  ( -26.95239803419980973, 3.927549058536718106E-14, 37.87317709539253485 ) ) ;
#4718=VECTOR ( 'NONE', #2749, 1000.000000000000000 ) ;
#4745=ADVANCED_FACE ( 'NONE', ( #9030 ), #23392, .F. ) ;
#4765=LINE ( 'NONE', #18761, #5275 ) ;
#4768=ORIENTED_EDGE ( 'NONE', *, *, #8887, .T. ) ;
#4769=CIRCLE ( 'NONE', #15317, 27.50000000000000000 ) ;
#4771=VERTEX_POINT ( 'NONE', #6668 ) ;
#4774=ORIENTED_EDGE ( 'NONE', *, *, #25154, .F. ) ;
#4775=CARTESIAN_POINT ( 'NONE',  ( 0.000000000000000000, 0.000000000000000000, 115.0000000000000000 ) ) ;
#4777=EDGE_CURVE ( 'NONE', #10568, #6141, #24662, .T. ) ;
#4782=CARTESIAN_POINT ( 'NONE',  ( -7.105427357599999217E-15, -7.105427357599999217E-15, 186.7828584120000244 ) ) ;
#4798=CARTESIAN_POINT ( 'NONE',  ( -1.100000000000000089, -17.25771824079999917, 5.000000000000000000 ) ) ;
#4803=CARTESIAN_POINT ( 'NONE',  ( 27.50000000000000000, -1.044349611129999949E-13, 0.000000000000000000 ) ) ;
#4805=FACE_OUTER_BOUND ( 'NONE', #5454, .T. ) ;
#4812=VERTEX_POINT ( 'NONE', #9338 ) ;
#4820=CARTESIAN_POINT ( 'NONE',  ( 0.8805184772471983390, -27.48609199509227352, 224.3250316508714661 ) ) ;
#4821=CARTESIAN_POINT ( 'NONE',  ( -11.08346179031913437, -28.41490585489481191, 193.6055512750000105 ) ) ;
#4823=CARTESIAN_POINT ( 'NONE',  ( -1.100000000000000089, -26.77741585740000119, 225.0000000000000000 ) ) ;
#4827=DIRECTION ( 'NONE',  ( 0.000000000000000000, 0.000000000000000000, 1.000000000000000000 ) ) ;
#4831=CARTESIAN_POINT ( 'NONE',  ( -7.838355892653579460, -25.63086664713629759, 207.3305258794510166 ) ) ;
#4840=ORIENTED_EDGE ( 'NONE', *, *, #28591, .F. ) ;
#4843=ORIENTED_EDGE ( 'NONE', *, *, #23886, .F. ) ;
#4857=CARTESIAN_POINT ( 'NONE',  ( -22.63992238019999803, -14.34133587289999845, 5.000000000000000000 ) ) ;
#4876=ORIENTED_EDGE ( 'NONE', *, *, #1982, .T. ) ;
#4880=EDGE_LOOP ( 'NONE', ( #13102, #7729, #5992, #20078, #15839, #24120 ) ) ;
#4883=ORIENTED_EDGE ( 'NONE', *, *, #20470, .T. ) ;
#4887=CARTESIAN_POINT ( 'NONE',  ( -8.903108651239966420, -22.82508830966961000, 190.0000000000000000 ) ) ;
#4900=FACE_OUTER_BOUND ( 'NONE', #29909, .T. ) ;
#4911=LINE ( 'NONE', #21747, #17809 ) ;
#4917=ORIENTED_EDGE ( 'NONE', *, *, #6056, .T. ) ;
#4923=ORIENTED_EDGE ( 'NONE', *, *, #5389, .T. ) ;
#4931=DIRECTION ( 'NONE',  ( 0.9316362575375356503, 0.3633921898465274913, 0.000000000000000000 ) ) ;
#4935=ORIENTED_EDGE ( 'NONE', *, *, #25863, .T. ) ;
#4942=DIRECTION ( 'NONE',  ( 1.224606353819999829E-16, 1.000000000000000000, 0.000000000000000000 ) ) ;
#4944=ORIENTED_EDGE ( 'NONE', *, *, #16041, .F. ) ;
#4947=AXIS2_PLACEMENT_3D ( 'NONE', #25805, #20922, #8627 ) ;
#4949=EDGE_LOOP ( 'NONE', ( #22413, #27085, #7136, #26059 ) ) ;
#4953=ORIENTED_EDGE ( 'NONE', *, *, #6593, .T. ) ;
#4954=DIRECTION ( 'NONE',  ( -0.8090169943751909232, 0.5877852522921378498, 0.000000000000000000 ) ) ;
#4967=AXIS2_PLACEMENT_3D ( 'NONE', #10051, #5470, #7526 ) ;
#4979=CARTESIAN_POINT ( 'NONE',  ( -0.8466629493849215926, -26.78674366432005982, 225.7036427418658775 ) ) ;
#4980=DIRECTION ( 'NONE',  ( -1.000000000000000000, 1.224606353819999829E-16, 0.000000000000000000 ) ) ;
#4985=CARTESIAN_POINT ( 'NONE',  ( 7.105427357599999217E-15, 8.881784196999999612E-15, 43.60555127550000520 ) ) ;
#4986=EDGE_CURVE ( 'NONE', #3686, #24086, #29401, .T. ) ;
#4991=CIRCLE ( 'NONE', #6497, 27.92857142840000151 ) ;
#5002=ADVANCED_FACE ( 'NONE', ( #22395 ), #29462, .F. ) ;
#5009=EDGE_CURVE ( 'NONE', #9711, #20581, #7798, .T. ) ;
#5012=CIRCLE ( 'NONE', #22110, 3.200000004570001888 ) ;
#5013=CARTESIAN_POINT ( 'NONE',  ( 0.2182390026759475909, -27.49908342132813033, 226.0877068033350099 ) ) ;
#5016=FACE_OUTER_BOUND ( 'NONE', #28886, .T. ) ;
#5019=CARTESIAN_POINT ( 'NONE',  ( 0.2196051099681128049, -26.79904497464113078, 223.9123790608769866 ) ) ;
#5032=ORIENTED_EDGE ( 'NONE', *, *, #1945, .F. ) ;
#5044=CARTESIAN_POINT ( 'NONE',  ( -22.63996098036293247, -14.34127493679862120, 5.145878552503609704 ) ) ;
#5057=CARTESIAN_POINT ( 'NONE',  ( 9.897162125334212135, -25.37356426560172906, 141.6604601749999972 ) ) ;
#5058=EDGE_CURVE ( 'NONE', #18447, #11838, #17898, .T. ) ;
#5081=ORIENTED_EDGE ( 'NONE', *, *, #19270, .F. ) ;
#5082=CIRCLE ( 'NONE', #15611, 27.50000000000000000 ) ;
#5085=CARTESIAN_POINT ( 'NONE',  ( 26.84464184930000030, -3.287411897459999980E-15, 87.43750406040000200 ) ) ;
#5088=CARTESIAN_POINT ( 'NONE',  ( 27.23548387180000319, -3.335274659869999873E-15, 91.66046017409999536 ) ) ;
#5098=EDGE_CURVE ( 'NONE', #26548, #28697, #26895, .T. ) ;
#5100=LINE ( 'NONE', #14712, #4718 ) ;
#5104=ORIENTED_EDGE ( 'NONE', *, *, #4986, .F. ) ;
#5112=CARTESIAN_POINT ( 'NONE',  ( -24.29812717100513098, -12.87956648280661831, 4.509445856313639922 ) ) ;
#5118=CARTESIAN_POINT ( 'NONE',  ( 7.105427357599999217E-15, 3.552713678799999608E-15, 41.66046017469999896 ) ) ;
#5122=AXIS2_PLACEMENT_3D ( 'NONE', #314, #29084, #17122 ) ;
#5128=CARTESIAN_POINT ( 'NONE',  ( -3.552713678799999608E-15, 0.000000000000000000, 43.21714158840000408 ) ) ;
#5138=ORIENTED_EDGE ( 'NONE', *, *, #30018, .F. ) ;
#5141=VERTEX_POINT ( 'NONE', #13879 ) ;
#5148=DIRECTION ( 'NONE',  ( 0.000000000000000000, 0.000000000000000000, 1.000000000000000000 ) ) ;
#5157=DIRECTION ( 'NONE',  ( 0.8660254037843289066, -0.5000000000001899592, 0.000000000000000000 ) ) ;
#5160=CARTESIAN_POINT ( 'NONE',  ( 0.000000000000000000, 0.000000000000000000, 42.06031501460000044 ) ) ;
#5164=CARTESIAN_POINT ( 'NONE',  ( 1.100000000000000533, -26.77741585740001184, 224.9029409945208613 ) ) ;
#5167=EDGE_CURVE ( 'NONE', #4565, #16141, #8885, .T. ) ;
#5179=ORIENTED_EDGE ( 'NONE', *, *, #5805, .T. ) ;
#5183=FACE_OUTER_BOUND ( 'NONE', #18417, .T. ) ;
#5191=ORIENTED_EDGE ( 'NONE', *, *, #22922, .F. ) ;
#5207=VERTEX_POINT ( 'NONE', #6631 ) ;
#5208=ADVANCED_FACE ( 'NONE', ( #16230 ), #20643, .F. ) ;
#5213=EDGE_CURVE ( 'NONE', #13677, #6141, #1924, .T. ) ;
#5218=ORIENTED_EDGE ( 'NONE', *, *, #19252, .F. ) ;
#5222=CARTESIAN_POINT ( 'NONE',  ( 27.23548387100000312, -3.552713678799999608E-15, 38.33953982530000104 ) ) ;
#5226=CIRCLE ( 'NONE', #9239, 4.000000000000000888 ) ;
#5229=B_SPLINE_CURVE_WITH_KNOTS ( 'NONE', 5,
 ( #23713, #26072, #29301, #21188, #24596, #7895 ),
 .UNSPECIFIED., .F., .F.,
 ( 6, 6 ),
 ( 0.000000000000000000, 2.319814960350000010 ),
 .UNSPECIFIED. ) ;
#5231=DIRECTION ( 'NONE',  ( 0.3633921898465272138, -0.9316362575375356503, -9.251858538542967489E-15 ) ) ;
#5242=CARTESIAN_POINT ( 'NONE',  ( 1.100000000000000089, -26.77741585740000119, 5.000000000000000000 ) ) ;
#5243=DIRECTION ( 'NONE',  ( 1.000000000000000000, 0.000000000000000000, 0.000000000000000000 ) ) ;
#5244=CARTESIAN_POINT ( 'NONE',  ( 27.92857142820000149, 1.776356839399999804E-15, 192.0603150150000147 ) ) ;
#5248=CARTESIAN_POINT ( 'NONE',  ( 27.06563794080000207, -3.314475219239999417E-15, 191.9402686260000053 ) ) ;
#5256=AXIS2_PLACEMENT_3D ( 'NONE', #15966, #4010, #13607 ) ;
#5258=B_SPLINE_CURVE_WITH_KNOTS ( 'NONE', 3,
 ( #30456, #9344, #11249, #30758, #8878, #28080, #25576, #28398, #30613, #16274, #23534, #6525 ),
 .UNSPECIFIED., .F., .F.,
 ( 4, 2, 2, 2, 2, 4 ),
 ( 0.000000000000000000, 0.2500000000000021094, 0.3750000000000024980, 0.5000000000000028866, 0.7500000000000014433, 1.000000000000000000 ),
 .UNSPECIFIED. ) ;
#5262=VERTEX_POINT ( 'NONE', #29118 ) ;
#5270=ADVANCED_FACE ( 'NONE', ( #4900 ), #6945, .F. ) ;
#5272=CARTESIAN_POINT ( 'NONE',  ( -24.05715877250037948, -13.32261293358842025, 4.005116771804169140 ) ) ;
#5275=VECTOR ( 'NONE', #28362, 1000.000000000000000 ) ;
#5279=EDGE_CURVE ( 'NONE', #21828, #21856, #23354, .T. ) ;
#5286=CARTESIAN_POINT ( 'NONE',  ( 23.20948082139999968, -13.40000000000000036, 223.8999999999999773 ) ) ;
#5304=ORIENTED_EDGE ( 'NONE', *, *, #14737, .T. ) ;
#5307=VERTEX_POINT ( 'NONE', #14657 ) ;
#5309=ORIENTED_EDGE ( 'NONE', *, *, #2339, .T. ) ;
#5312=FACE_OUTER_BOUND ( 'NONE', #1633, .T. ) ;
#5323=CARTESIAN_POINT ( 'NONE',  ( -27.76135143710000008, 3.399672736049999681E-15, 187.6614141010000196 ) ) ;
#5327=CARTESIAN_POINT ( 'NONE',  ( -27.06563794070000029, 3.314475219249999806E-15, 141.9402686260000053 ) ) ;
#5330=EDGE_CURVE ( 'NONE', #3101, #27268, #28858, .T. ) ;
#5335=CARTESIAN_POINT ( 'NONE',  ( 23.95771898011812340, -13.50170546717094311, 3.928090679509207206 ) ) ;
#5337=ORIENTED_EDGE ( 'NONE', *, *, #22251, .F. ) ;
#5338=ADVANCED_FACE ( 'NONE', ( #26300 ), #21268, .F. ) ;
#5342=B_SPLINE_CURVE_WITH_KNOTS ( 'NONE', 3,
 ( #4661, #28267, #21661, #9217, #18977, #23415, #23875, #4197, #28585, #11743, #11595, #9691 ),
 .UNSPECIFIED., .F., .F.,
 ( 4, 2, 2, 2, 2, 4 ),
 ( 0.000000000000000000, 0.2500000000000334177, 0.3750000000000278666, 0.5000000000000223155, 0.7500000000000111022, 1.000000000000000000 ),
 .UNSPECIFIED. ) ;
#5352=CARTESIAN_POINT ( 'NONE',  ( 28.50000000000000000, -3.490128108379999702E-15, 40.00000000000000000 ) ) ;
#5367=ORIENTED_EDGE ( 'NONE', *, *, #3492, .T. ) ;
#5375=CARTESIAN_POINT ( 'NONE',  ( 9.738910687886868089, -24.96785170200598358, 36.78285841123148003 ) ) ;
#5376=ORIENTED_EDGE ( 'NONE', *, *, #14126, .F. ) ;
#5389=EDGE_CURVE ( 'NONE', #22997, #6732, #15815, .T. ) ;
#5401=ORIENTED_EDGE ( 'NONE', *, *, #23222, .T. ) ;
#5410=( LENGTH_UNIT ( ) NAMED_UNIT ( * ) SI_UNIT ( .MILLI., .METRE. ) );
#5411=AXIS2_PLACEMENT_3D ( 'NONE', #28568, #25750, #23077 ) ;
#5414=AXIS2_PLACEMENT_3D ( 'NONE', #9819, #16892, #9975 ) ;
#5416=ORIENTED_EDGE ( 'NONE', *, *, #26922, .T. ) ;
#5421=CARTESIAN_POINT ( 'NONE',  ( -24.34663841808528062, -12.78636765232546324, 4.903540287127751363 ) ) ;
#5435=CARTESIAN_POINT ( 'NONE',  ( -4.671347416476984371, -26.39088508839784453, 209.5126867146601910 ) ) ;
#5437=AXIS2_PLACEMENT_3D ( 'NONE', #1025, #5880, #15636 ) ;
#5439=CARTESIAN_POINT ( 'NONE',  ( 1.071537507505435638, -27.47917025549320513, 4.713010325135398304 ) ) ;
#5442=CARTESIAN_POINT ( 'NONE',  ( -1.841797396446221979, -26.73663745407121795, 20.00000000000000355 ) ) ;
#5453=ORIENTED_EDGE ( 'NONE', *, *, #22848, .F. ) ;
#5454=EDGE_LOOP ( 'NONE', ( #19933, #23219, #15745, #8653, #11798, #2557, #27583, #5376, #7972, #12452 ) ) ;
#5470=DIRECTION ( 'NONE',  ( 0.000000000000000000, 0.000000000000000000, 1.000000000000000000 ) ) ;
#5475=CARTESIAN_POINT ( 'NONE',  ( 11.08346179031909529, -28.41490585489483678, 136.3944487250000179 ) ) ;
#5495=CARTESIAN_POINT ( 'NONE',  ( 0.000000000000000000, 0.000000000000000000, 115.0000000000000000 ) ) ;
#5521=ORIENTED_EDGE ( 'NONE', *, *, #28501, .T. ) ;
#5523=DIRECTION ( 'NONE',  ( 0.000000000000000000, 0.000000000000000000, 1.000000000000000000 ) ) ;
#5527=ORIENTED_EDGE ( 'NONE', *, *, #26629, .F. ) ;
#5535=AXIS2_PLACEMENT_3D ( 'NONE', #10541, #19676, #8154 ) ;
#5538=DIRECTION ( 'NONE',  ( 1.000000000000000000, 0.000000000000000000, 0.000000000000000000 ) ) ;
#5552=EDGE_LOOP ( 'NONE', ( #22733, #20786, #28170, #15062 ) ) ;
#5577=UNCERTAINTY_MEASURE_WITH_UNIT (LENGTH_MEASURE( 1.000000000000000082E-05 ), #22570, 'distance_accuracy_value', 'NONE');
#5582=CARTESIAN_POINT ( 'NONE',  ( 18.95046173579999760, -18.95046173579999760, 36.78285841159999592 ) ) ;
#5584=DIRECTION ( 'NONE',  ( 0.000000000000000000, 0.000000000000000000, 1.000000000000000000 ) ) ;
#5594=CARTESIAN_POINT ( 'NONE',  ( -24.31247271682646272, -11.33627354958356825, 93.21714158842222275 ) ) ;
#5596=ORIENTED_EDGE ( 'NONE', *, *, #21169, .T. ) ;
#5603=ORIENTED_EDGE ( 'NONE', *, *, #1163, .F. ) ;
#5604=PRODUCT_DEFINITION ( 'UNKNOWN', '', #11850, #7480 ) ;
#5605=B_SPLINE_CURVE_WITH_KNOTS ( 'NONE', 3,
 ( #25718, #15792, #18616, #4151, #13745, #1324, #1950, #11228, #4311, #23360 ),
 .UNSPECIFIED., .F., .F.,
 ( 4, 2, 2, 2, 4 ),
 ( 0.000000000000000000, 0.2500000000000000000, 0.5000000000000000000, 0.7500000000000000000, 1.000000000000000000 ),
 .UNSPECIFIED. ) ;
#5609=VERTEX_POINT ( 'NONE', #28889 ) ;
#5611=CARTESIAN_POINT ( 'NONE',  ( -23.25782843603512617, -13.31625947502723939, 226.1000000000011880 ) ) ;
#5612=CIRCLE ( 'NONE', #114, 26.80000000000000071 ) ;
#5625=CARTESIAN_POINT ( 'NONE',  ( 18.95046173579999760, -18.95046173579999760, 86.78285841159998881 ) ) ;
#5630=CARTESIAN_POINT ( 'NONE',  ( 7.833397470852297317, -25.63019328476620018, 207.3161515959309895 ) ) ;
#5633=CARTESIAN_POINT ( 'NONE',  ( -24.76259292740831697, -10.24958551592169265, 43.21714158839987618 ) ) ;
#5634=VECTOR ( 'NONE', #24138, 1000.000000000000114 ) ;
#5635=CARTESIAN_POINT ( 'NONE',  ( 24.34663841809999951, -12.78636765230000094, 225.0000000000000000 ) ) ;
#5643=ORIENTED_EDGE ( 'NONE', *, *, #24613, .T. ) ;
#5652=DIRECTION ( 'NONE',  ( 0.000000000000000000, 0.000000000000000000, 1.000000000000000000 ) ) ;
#5653=LINE ( 'NONE', #27369, #13591 ) ;
#5662=ADVANCED_FACE ( 'NONE', ( #19915 ), #20375, .F. ) ;
#5669=LINE ( 'NONE', #22365, #7715 ) ;
#5682=VERTEX_POINT ( 'NONE', #17540 ) ;
#5687=ADVANCED_FACE ( 'NONE', ( #8091 ), #28370, .F. ) ;
#5701=DIRECTION ( 'NONE',  ( 1.224606353819999829E-16, 1.000000000000000000, 0.000000000000000000 ) ) ;
#5703=DIRECTION ( 'NONE',  ( 0.000000000000000000, 0.000000000000000000, 1.000000000000000000 ) ) ;
#5704=CARTESIAN_POINT ( 'NONE',  ( -24.49999999589999788, 3.000285566369999841E-15, 190.0000000000000000 ) ) ;
#5730=DIRECTION ( 'NONE',  ( 0.3633921898465272138, -0.9316362575375356503, -2.312964634635741872E-15 ) ) ;
#5735=CARTESIAN_POINT ( 'NONE',  ( -26.80000000069999899, 3.281945028329999726E-15, 92.88981852279999885 ) ) ;
#5750=CARTESIAN_POINT ( 'NONE',  ( -18.95046173579999760, -18.95046173579999760, 93.21714158839999698 ) ) ;
#5755=FACE_OUTER_BOUND ( 'NONE', #30389, .T. ) ;
#5756=DIRECTION ( 'NONE',  ( 0.000000000000000000, 0.000000000000000000, 1.000000000000000000 ) ) ;
#5764=ORIENTED_EDGE ( 'NONE', *, *, #27686, .T. ) ;
#5766=CARTESIAN_POINT ( 'NONE',  ( -23.68723484211243147, -12.53725850803311914, 225.4947892886579552 ) ) ;
#5780=CARTESIAN_POINT ( 'NONE',  ( -27.23548386990000125, 3.335274659649999582E-15, 188.3395398260000206 ) ) ;
#5782=AXIS2_PLACEMENT_3D ( 'NONE', #13214, #20305, #1278 ) ;
#5783=DIRECTION ( 'NONE',  ( 0.000000000000000000, 0.000000000000000000, -1.000000000000000000 ) ) ;
#5789=DIRECTION ( 'NONE',  ( 0.9316362575375356503, 0.3633921898465274913, 0.000000000000000000 ) ) ;
#5791=CARTESIAN_POINT ( 'NONE',  ( -24.76914019444431858, -10.23375669952357470, 43.21714158839954933 ) ) ;
#5792=CARTESIAN_POINT ( 'NONE',  ( 9.543143524407904366, -25.04338540923419743, 26.16054379342799052 ) ) ;
#5793=ORIENTED_EDGE ( 'NONE', *, *, #106, .T. ) ;
#5795=ADVANCED_FACE ( 'NONE', ( #9184, #1816 ), #11246, .F. ) ;
#5799=ORIENTED_EDGE ( 'NONE', *, *, #12141, .F. ) ;
#5802=ORIENTED_EDGE ( 'NONE', *, *, #13633, .T. ) ;
#5805=EDGE_CURVE ( 'NONE', #3582, #14877, #27871, .T. ) ;
#5808=FACE_OUTER_BOUND ( 'NONE', #3876, .T. ) ;
#5827=CARTESIAN_POINT ( 'NONE',  ( 0.000000000000000000, 0.000000000000000000, 40.00000000000000000 ) ) ;
#5833=CARTESIAN_POINT ( 'NONE',  ( -0.6805621215738131280, -26.79155678488164938, 4.123352033172330344 ) ) ;
#5837=EDGE_LOOP ( 'NONE', ( #13417, #29365, #182, #23435 ) ) ;
#5838=CARTESIAN_POINT ( 'NONE',  ( 9.897162125403639266, -25.37356426577971646, 41.66046017469999896 ) ) ;
#5840=DIRECTION ( 'NONE',  ( 1.000000000000000000, -1.224606353819999582E-16, 0.000000000000000000 ) ) ;
#5850=CARTESIAN_POINT ( 'NONE',  ( -0.1477568774490881365, -27.50000000000000711, 6.100000000000010303 ) ) ;
#5857=ORIENTED_EDGE ( 'NONE', *, *, #21179, .F. ) ;
#5859=CARTESIAN_POINT ( 'NONE',  ( -9.738910687886855655, -24.96785170200598714, 36.78285841123146582 ) ) ;
#5871=DIRECTION ( 'NONE',  ( 0.3633921898465291567, 0.9316362575375349842, 0.000000000000000000 ) ) ;
#5875=AXIS2_PLACEMENT_3D ( 'NONE', #8947, #18546, #15710 ) ;
#5880=DIRECTION ( 'NONE',  ( -0.8660254037843290176, 0.5000000000001899592, -1.018673689593249976E-32 ) ) ;
#5901=CARTESIAN_POINT ( 'NONE',  ( -22.81399828927099449, -14.09994392937125518, 93.21714158846111786 ) ) ;
#5912=CIRCLE ( 'NONE', #420, 4.000000000000000888 ) ;
#5917=CARTESIAN_POINT ( 'NONE',  ( -23.31771987846477145, -13.21065015015469868, 226.0876905690154786 ) ) ;
#5918=CARTESIAN_POINT ( 'NONE',  ( -23.25788685383075460, -13.43083806724684770, 143.2171415880000040 ) ) ;
#5921=AXIS2_PLACEMENT_3D ( 'NONE', #14394, #14699, #28846 ) ;
#5922=CARTESIAN_POINT ( 'NONE',  ( -24.49999999589999788, 3.000285566369999841E-15, 90.00000000000000000 ) ) ;
#5945=EDGE_CURVE ( 'NONE', #28212, #16979, #16737, .T. ) ;
#5949=EDGE_CURVE ( 'NONE', #24427, #1634, #21992, .T. ) ;
#5952=VERTEX_POINT ( 'NONE', #12791 ) ;
#5957=EDGE_CURVE ( 'NONE', #19471, #4565, #29772, .T. ) ;
#5958=FACE_OUTER_BOUND ( 'NONE', #26778, .T. ) ;
#5959=DIRECTION ( 'NONE',  ( 1.224606353819999829E-16, 1.000000000000000000, 0.000000000000000000 ) ) ;
#5969=DIRECTION ( 'NONE',  ( -1.000000000000000000, 1.224606353819999829E-16, 0.000000000000000000 ) ) ;
#5972=CARTESIAN_POINT ( 'NONE',  ( -9.738910687886855655, -24.96785170200598714, 202.0000000000000000 ) ) ;
#5976=CARTESIAN_POINT ( 'NONE',  ( -27.76135144259999876, 3.399672736729999754E-15, 92.33858589269999584 ) ) ;
#5979=EDGE_CURVE ( 'NONE', #9833, #25397, #28002, .T. ) ;
#5980=AXIS2_PLACEMENT_3D ( 'NONE', #20850, #23681, #4322 ) ;
#5982=DIRECTION ( 'NONE',  ( -0.5000000000001898481, -0.8660254037843291286, 0.000000000000000000 ) ) ;
#5985=CARTESIAN_POINT ( 'NONE',  ( 0.000000000000000000, 0.000000000000000000, 20.00000000000000355 ) ) ;
#5986=ORIENTED_EDGE ( 'NONE', *, *, #24795, .T. ) ;
#5988=CARTESIAN_POINT ( 'NONE',  ( -7.365079183348027136, -26.49619795852260040, 21.94317657039426805 ) ) ;
#5992=ORIENTED_EDGE ( 'NONE', *, *, #1511, .F. ) ;
#6000=CARTESIAN_POINT ( 'NONE',  ( 4.182178350032534908, -27.18131967880234257, 209.7454400431937813 ) ) ;
#6013=AXIS2_PLACEMENT_3D ( 'NONE', #4887, #12114, #14492 ) ;
#6026=ORIENTED_EDGE ( 'NONE', *, *, #16439, .F. ) ;
#6034=VECTOR ( 'NONE', #10154, 1000.000000000000114 ) ;
#6037=CARTESIAN_POINT ( 'NONE',  ( -23.25801811775868799, -13.31593093575191666, 6.100000000003494627 ) ) ;
#6041=CARTESIAN_POINT ( 'NONE',  ( -26.80000000069999899, 3.281945028329999726E-15, 42.88981852279999885 ) ) ;
#6043=EDGE_CURVE ( 'NONE', #14251, #28953, #22326, .T. ) ;
#6045=EDGE_LOOP ( 'NONE', ( #25766, #10380, #17849, #10213 ) ) ;
#6048=LINE ( 'NONE', #1340, #23357 ) ;
#6055=CARTESIAN_POINT ( 'NONE',  ( -14.39562240800000126, -9.581487064249998298, 5.000000000000000000 ) ) ;
#6056=EDGE_CURVE ( 'NONE', #7318, #6778, #15151, .T. ) ;
#6061=B_SPLINE_CURVE_WITH_KNOTS ( 'NONE', 3,
 ( #18556, #20604, #18400, #6290, #20925, #4395, #11328, #23453, #3932, #11482, #16044, #1883, #9261, #1579 ),
 .UNSPECIFIED., .F., .F.,
 ( 4, 2, 2, 2, 2, 2, 4 ),
 ( 0.000000000000000000, 0.2499999999999984457, 0.3749999999999976130, 0.4374999999999976130, 0.4999999999999976685, 0.7499999999999988898, 1.000000000000000000 ),
 .UNSPECIFIED. ) ;
#6065=AXIS2_PLACEMENT_3D ( 'NONE', #11875, #6682, #25899 ) ;
#6082=CARTESIAN_POINT ( 'NONE',  ( -27.23548387060000309, 7.105427357599999217E-15, 141.6604601749999972 ) ) ;
#6086=DIRECTION ( 'NONE',  ( 0.000000000000000000, 0.000000000000000000, 1.000000000000000000 ) ) ;
#6090=DIRECTION ( 'NONE',  ( 0.000000000000000000, 0.000000000000000000, 1.000000000000000000 ) ) ;
#6105=ORIENTED_EDGE ( 'NONE', *, *, #27878, .F. ) ;
#6113=B_SPLINE_CURVE_WITH_KNOTS ( 'NONE', 3,
 ( #6587, #20437, #10684, #6280, #3919, #20280, #3595, #25322, #8623, #15709, #25163, #3764, #18391, #1411 ),
 .UNSPECIFIED., .F., .F.,
 ( 4, 2, 2, 2, 2, 2, 4 ),
 ( 0.000000000000000000, 0.2500000000000006106, 0.3750000000000009992, 0.4375000000000012768, 0.5000000000000015543, 0.7500000000000006661, 1.000000000000000000 ),
 .UNSPECIFIED. ) ;
#6124=EDGE_CURVE ( 'NONE', #2408, #22757, #13883, .T. ) ;
#6127=CARTESIAN_POINT ( 'NONE',  ( 23.81569860410000317, -13.75000000000000000, 6.099999999630000502 ) ) ;
#6137=VERTEX_POINT ( 'NONE', #30718 ) ;
#6141=VERTEX_POINT ( 'NONE', #30415 ) ;
#6142=CARTESIAN_POINT ( 'NONE',  ( -2.639108104135487576, -27.37825522961219704, 20.00000000000000355 ) ) ;
#6153=DIRECTION ( 'NONE',  ( 0.000000000000000000, 0.000000000000000000, 1.000000000000000000 ) ) ;
#6154=CARTESIAN_POINT ( 'NONE',  ( 2.639108104135504007, -27.37825522961219704, 210.0000000000000853 ) ) ;
#6156=CARTESIAN_POINT ( 'NONE',  ( 27.23548387060000309, -1.776356839399999804E-15, 188.3395398250000028 ) ) ;
#6160=CARTESIAN_POINT ( 'NONE',  ( -4.696583076644003540, -27.09716880376585380, 209.5942911595222995 ) ) ;
#6167=EDGE_CURVE ( 'NONE', #20581, #11717, #12720, .T. ) ;
#6174=CIRCLE ( 'NONE', #6692, 3.199999983039998774 ) ;
#6179=VERTEX_POINT ( 'NONE', #15926 ) ;
#6181=CARTESIAN_POINT ( 'NONE',  ( 23.25788685383077592, -13.43083806724684948, 186.7828584119999391 ) ) ;
#6182=EDGE_LOOP ( 'NONE', ( #18605, #369, #6813, #14908, #20275 ) ) ;
#6184=ORIENTED_EDGE ( 'NONE', *, *, #10047, .T. ) ;
#6189=EDGE_CURVE ( 'NONE', #12912, #13582, #23794, .T. ) ;
#6202=CARTESIAN_POINT ( 'NONE',  ( 25.94128158184369681, -6.955966684932006316, 0.000000000000000000 ) ) ;
#6204=ORIENTED_EDGE ( 'NONE', *, *, #3704, .F. ) ;
#6206=CARTESIAN_POINT ( 'NONE',  ( -22.70032920229352769, -14.24644155152564373, 4.508626839105193795 ) ) ;
#6209=PLANE ( 'NONE',  #17535 ) ;
#6212=CARTESIAN_POINT ( 'NONE',  ( 27.69999999930000101, -3.392159599989999961E-15, 140.0000000000000000 ) ) ;
#6218=CIRCLE ( 'NONE', #17262, 27.23548387100000312 ) ;
#6220=DIRECTION ( 'NONE',  ( 0.000000000000000000, 0.000000000000000000, -1.000000000000000000 ) ) ;
#6221=CARTESIAN_POINT ( 'NONE',  ( -24.33346004068009449, -12.81155130651987406, 225.2867514112106733 ) ) ;
#6230=EDGE_CURVE ( 'NONE', #13263, #20656, #685, .T. ) ;
#6233=ORIENTED_EDGE ( 'NONE', *, *, #12323, .F. ) ;
#6241=CIRCLE ( 'NONE', #16793, 3.000000000000001332 ) ;
#6242=B_SPLINE_CURVE_WITH_KNOTS ( 'NONE', 3,
 ( #24673, #7977, #15379, #22626, #24977, #3413, #13015, #1067, #10657, #20248, #23251, #15529, #16006, #6405 ),
 .UNSPECIFIED., .F., .F.,
 ( 4, 2, 2, 2, 2, 2, 4 ),
 ( 0.000000000000000000, 0.2500000000000003331, 0.3750000000000004996, 0.4375000000000000000, 0.4999999999999995559, 0.7499999999999997780, 1.000000000000000000 ),
 .UNSPECIFIED. ) ;
#6247=ORIENTED_EDGE ( 'NONE', *, *, #10579, .F. ) ;
#6263=AXIS2_PLACEMENT_3D ( 'NONE', #20529, #5584, #12832 ) ;
#6264=CARTESIAN_POINT ( 'NONE',  ( -24.13062658854171971, -13.18986347145018634, 224.0869147258247835 ) ) ;
#6274=AXIS2_PLACEMENT_3D ( 'NONE', #16492, #4232, #27987 ) ;
#6278=FACE_OUTER_BOUND ( 'NONE', #9523, .T. ) ;
#6280=CARTESIAN_POINT ( 'NONE',  ( -1.019043872447617405, -27.48159911132789901, 4.579737331571473113 ) ) ;
#6285=CIRCLE ( 'NONE', #8724, 26.80000000000000071 ) ;
#6290=CARTESIAN_POINT ( 'NONE',  ( -1.018916986544576408, -26.78112380547544547, 5.420582067115832459 ) ) ;
#6298=AXIS2_PLACEMENT_3D ( 'NONE', #29767, #10583, #19724 ) ;
#6301=EDGE_CURVE ( 'NONE', #5952, #19818, #27798, .T. ) ;
#6306=CARTESIAN_POINT ( 'NONE',  ( -18.95046173579999760, -18.95046173579999760, 115.0000000000000000 ) ) ;
#6308=CARTESIAN_POINT ( 'NONE',  ( -6.756062549273579521, -26.65810324902504291, 21.45434275270897118 ) ) ;
#6309=VERTEX_POINT ( 'NONE', #25963 ) ;
#6310=EDGE_LOOP ( 'NONE', ( #22793, #6814, #18130, #25347 ) ) ;
#6319=CARTESIAN_POINT ( 'NONE',  ( -26.93395402219999824, 3.298349122909999612E-15, 137.7567592739999895 ) ) ;
#6320=CARTESIAN_POINT ( 'NONE',  ( 23.63627835225026530, -12.63201688062175698, 5.666076084815439451 ) ) ;
#6322=CARTESIAN_POINT ( 'NONE',  ( 27.06563796010000189, -3.314475221599999482E-15, 188.0597313979999967 ) ) ;
#6326=CARTESIAN_POINT ( 'NONE',  ( -3.163284386374744628, -27.32243547426060815, 209.9517032567745503 ) ) ;
#6331=DIRECTION ( 'NONE',  ( -0.9316362575375349842, 0.3633921898465292122, -0.000000000000000000 ) ) ;
#6341=ORIENTED_EDGE ( 'NONE', *, *, #2339, .F. ) ;
#6347=CARTESIAN_POINT ( 'NONE',  ( 24.28117756997326637, -12.91036561242075997, 4.443835645643864574 ) ) ;
#6366=ORIENTED_EDGE ( 'NONE', *, *, #24765, .F. ) ;
#6370=CARTESIAN_POINT ( 'NONE',  ( 15.49562240950000103, -7.676231176589999983, 225.0000000000000000 ) ) ;
#6373=EDGE_CURVE ( 'NONE', #14204, #24890, #8637, .T. ) ;
#6378=DIRECTION ( 'NONE',  ( 0.9316362575375356503, 0.3633921898465274913, 0.000000000000000000 ) ) ;
#6381=CIRCLE ( 'NONE', #31004, 3.200000004570001888 ) ;
#6394=CARTESIAN_POINT ( 'NONE',  ( 27.50000000000000000, -6.735334946019999940E-15, 36.39444872359999295 ) ) ;
#6397=DIRECTION ( 'NONE',  ( 0.8660254037843290176, 0.5000000000001899592, 0.000000000000000000 ) ) ;
#6405=CARTESIAN_POINT ( 'NONE',  ( 23.20948082139999968, -13.40000000000000036, 3.900000000369999942 ) ) ;
#6417=CARTESIAN_POINT ( 'NONE',  ( -0.4908581392059040982, -27.49541710664062677, 224.0051167709335402 ) ) ;
#6426=AXIS2_PLACEMENT_3D ( 'NONE', #9446, #19049, #28648 ) ;
#6429=DIRECTION ( 'NONE',  ( 1.000000000000000000, 0.000000000000000000, 0.000000000000000000 ) ) ;
#6447=CARTESIAN_POINT ( 'NONE',  ( 0.000000000000000000, 0.000000000000000000, 115.0000000000000000 ) ) ;
#6450=CARTESIAN_POINT ( 'NONE',  ( 27.63177356790000161, -3.383804547859999682E-15, 187.3605236429999934 ) ) ;
#6456=ORIENTED_EDGE ( 'NONE', *, *, #3237, .F. ) ;
#6459=ORIENTED_EDGE ( 'NONE', *, *, #3637, .T. ) ;
#6467=DIRECTION ( 'NONE',  ( -1.000000000000000000, 1.224606353819999829E-16, 0.000000000000000000 ) ) ;
#6470=DIRECTION ( 'NONE',  ( 0.9316362575375356503, 0.3633921898465274913, 0.000000000000000000 ) ) ;
#6477=CARTESIAN_POINT ( 'NONE',  ( -7.919194817802633679, -26.33574556704115466, 207.5082310198851019 ) ) ;
#6482=AXIS2_PLACEMENT_3D ( 'NONE', #23568, #11592, #16308 ) ;
#6483=CARTESIAN_POINT ( 'NONE',  ( 10.06596365874881194, -25.80632433378973900, 140.0000000000000000 ) ) ;
#6485=CARTESIAN_POINT ( 'NONE',  ( 0.000000000000000000, 0.000000000000000000, 91.66046017469999185 ) ) ;
#6491=CARTESIAN_POINT ( 'NONE',  ( -3.674376064820711107, -26.54820124389934577, 20.19531595841323579 ) ) ;
#6493=CIRCLE ( 'NONE', #26113, 27.23548387100000312 ) ;
#6497=AXIS2_PLACEMENT_3D ( 'NONE', #3326, #29297, #7889 ) ;
#6511=CARTESIAN_POINT ( 'NONE',  ( -23.52681767331053919, -12.83507605119044293, 5.909812226101280430 ) ) ;
#6515=STYLED_ITEM ( 'NONE', ( #23239 ), #688 ) ;
#6522=CARTESIAN_POINT ( 'NONE',  ( 7.105427357599999217E-15, 3.552713678799999608E-15, 43.21714158840000408 ) ) ;
#6524=CARTESIAN_POINT ( 'NONE',  ( 9.799563951679273188, -25.69477015992459101, 26.17015415056619432 ) ) ;
#6525=CARTESIAN_POINT ( 'NONE',  ( 23.20948082139999968, -13.40000000000000036, 3.900000000369999942 ) ) ;
#6530=VERTEX_POINT ( 'NONE', #22077 ) ;
#6544=ORIENTED_EDGE ( 'NONE', *, *, #13679, .T. ) ;
#6549=EDGE_CURVE ( 'NONE', #10339, #22309, #3244, .T. ) ;
#6553=ORIENTED_EDGE ( 'NONE', *, *, #23556, .F. ) ;
#6560=CARTESIAN_POINT ( 'NONE',  ( 10.35667741062603397, -26.55163333981976592, 140.0000000000000000 ) ) ;
#6576=ORIENTED_EDGE ( 'NONE', *, *, #3135, .T. ) ;
#6587=CARTESIAN_POINT ( 'NONE',  ( -1.100000000000000089, -27.47799119230000287, 5.000000000000000000 ) ) ;
#6588=CARTESIAN_POINT ( 'NONE',  ( 27.50000000000000000, -3.367667472999999580E-15, 93.28090191849999258 ) ) ;
#6591=ORIENTED_EDGE ( 'NONE', *, *, #16433, .F. ) ;
#6593=EDGE_CURVE ( 'NONE', #6773, #12147, #11301, .T. ) ;
#6603=DIRECTION ( 'NONE',  ( 0.000000000000000000, 0.000000000000000000, 1.000000000000000000 ) ) ;
#6608=CARTESIAN_POINT ( 'NONE',  ( -2.813083154009999692E-14, -26.79999999949999889, 3.899999999999999911 ) ) ;
#6613=ORIENTED_EDGE ( 'NONE', *, *, #21500, .F. ) ;
#6625=CARTESIAN_POINT ( 'NONE',  ( -26.80000000110000613, -1.759504892044711388, -0.000000000000000000 ) ) ;
#6628=AXIS2_PLACEMENT_3D ( 'NONE', #9584, #2507, #16507 ) ;
#6631=CARTESIAN_POINT ( 'NONE',  ( 27.92857142860000152, -3.116236426490000064E-16, 42.06031501460000044 ) ) ;
#6636=CARTESIAN_POINT ( 'NONE',  ( -8.903108651239966420, -22.82508830966961000, 90.00000000000000000 ) ) ;
#6656=FACE_OUTER_BOUND ( 'NONE', #29148, .T. ) ;
#6663=TOROIDAL_SURFACE ( 'NONE', #24253, 29.80000000000000071, 3.000000000000000000 ) ;
#6668=CARTESIAN_POINT ( 'NONE',  ( -9.897162125403683675, -25.37356426577969870, 41.66046017469999896 ) ) ;
#6670=AXIS2_PLACEMENT_3D ( 'NONE', #17509, #24605, #24290 ) ;
#6675=CARTESIAN_POINT ( 'NONE',  ( 7.919194817802646114, -26.33574556704115111, 22.49176898011488035 ) ) ;
#6682=DIRECTION ( 'NONE',  ( 0.000000000000000000, 0.000000000000000000, 1.000000000000000000 ) ) ;
#6689=B_SPLINE_CURVE_WITH_KNOTS ( 'NONE', 3,
 ( #4123, #30715, #21431, #9144, #13880, #13719, #18745, #23330, #28502, #16541 ),
 .UNSPECIFIED., .F., .F.,
 ( 4, 2, 2, 2, 4 ),
 ( 0.000000000000000000, 0.2500000000000000000, 0.5000000000000000000, 0.7500000000000000000, 1.000000000000000000 ),
 .UNSPECIFIED. ) ;
#6692=AXIS2_PLACEMENT_3D ( 'NONE', #28664, #2085, #26311 ) ;
#6700=CARTESIAN_POINT ( 'NONE',  ( -27.50000000000000000, 3.367667473009999970E-15, 115.0000000010000036 ) ) ;
#6701=CARTESIAN_POINT ( 'NONE',  ( -9.738910687886855655, -24.96785170200598714, 36.78285841123146582 ) ) ;
#6705=EDGE_CURVE ( 'NONE', #21828, #8486, #4524, .T. ) ;
#6708=CARTESIAN_POINT ( 'NONE',  ( 9.993285220779439371, -25.61999708228226069, 115.0000000000000000 ) ) ;
#6713=TOROIDAL_SURFACE ( 'NONE', #11748, 29.80000000000000071, 3.000000000000000000 ) ;
#6722=CARTESIAN_POINT ( 'NONE',  ( -23.92402432643254073, -13.56054118780705231, 223.9122931972334811 ) ) ;
#6732=VERTEX_POINT ( 'NONE', #20471 ) ;
#6758=AXIS2_PLACEMENT_3D ( 'NONE', #21733, #23641, #2078 ) ;
#6761=CARTESIAN_POINT ( 'NONE',  ( -24.34663841809999951, -12.78636765230000094, 225.0000000000000000 ) ) ;
#6773=VERTEX_POINT ( 'NONE', #18730 ) ;
#6778=VERTEX_POINT ( 'NONE', #13708 ) ;
#6806=CARTESIAN_POINT ( 'NONE',  ( 0.000000000000000000, 0.000000000000000000, 190.0000000000000000 ) ) ;
#6811=CARTESIAN_POINT ( 'NONE',  ( -2.664535259099999568E-14, -26.80000000000000071, 115.0000000000000000 ) ) ;
#6813=ORIENTED_EDGE ( 'NONE', *, *, #20390, .T. ) ;
#6814=ORIENTED_EDGE ( 'NONE', *, *, #14790, .T. ) ;
#6827=DIRECTION ( 'NONE',  ( 0.000000000000000000, 0.000000000000000000, 1.000000000000000000 ) ) ;
#6832=DIRECTION ( 'NONE',  ( 0.000000000000000000, 0.000000000000000000, 1.000000000000000000 ) ) ;
#6849=ORIENTED_EDGE ( 'NONE', *, *, #8074, .F. ) ;
#6850=CARTESIAN_POINT ( 'NONE',  ( 11.08346179031907930, -28.41490585489482257, 186.3944487249999895 ) ) ;
#6855=DIRECTION ( 'NONE',  ( 0.000000000000000000, 0.000000000000000000, -1.000000000000000000 ) ) ;
#6862=ADVANCED_FACE ( 'NONE', ( #5183 ), #19047, .T. ) ;
#6881=VERTEX_POINT ( 'NONE', #31009 ) ;
#6888=CIRCLE ( 'NONE', #27484, 4.000000000000000888 ) ;
#6890=DIRECTION ( 'NONE',  ( 1.000000000000000000, 0.000000000000000000, 0.000000000000000000 ) ) ;
#6901=B_SPLINE_CURVE_WITH_KNOTS ( 'NONE', 5,
 ( #22935, #3410, #8280, #20246, #29846, #25614 ),
 .UNSPECIFIED., .F., .F.,
 ( 6, 6 ),
 ( -2.300779717370000199, 0.000000000000000000 ),
 .UNSPECIFIED. ) ;
#6912=EDGE_CURVE ( 'NONE', #25637, #10339, #18062, .T. ) ;
#6923=ORIENTED_EDGE ( 'NONE', *, *, #18957, .T. ) ;
#6926=ORIENTED_EDGE ( 'NONE', *, *, #29953, .T. ) ;
#6931=DIRECTION ( 'NONE',  ( 1.000000000000000000, -1.224606353819999829E-16, 0.000000000000000000 ) ) ;
#6933=CIRCLE ( 'NONE', #2431, 27.92857142840000151 ) ;
#6939=CARTESIAN_POINT ( 'NONE',  ( -22.63992238019999803, -14.34133587289999845, 5.000000000000000000 ) ) ;
#6941=ORIENTED_EDGE ( 'NONE', *, *, #16694, .T. ) ;
#6942=TOROIDAL_SURFACE ( 'NONE', #26051, 24.50000000000000000, 3.200000000000000178 ) ;
#6945=CYLINDRICAL_SURFACE ( 'NONE', #14293, 26.80000000000002203 ) ;
#6957=ORIENTED_EDGE ( 'NONE', *, *, #29494, .F. ) ;
#6964=EDGE_CURVE ( 'NONE', #24321, #11773, #5012, .T. ) ;
#6965=CARTESIAN_POINT ( 'NONE',  ( 23.24663841809999809, -14.69162354060000020, 5.000000000000000000 ) ) ;
#6968=CIRCLE ( 'NONE', #3954, 26.80000000000000071 ) ;
#6981=EDGE_CURVE ( 'NONE', #18020, #18294, #26135, .T. ) ;
#6998=AXIS2_PLACEMENT_3D ( 'NONE', #14893, #15045, #17393 ) ;
#7001=EDGE_LOOP ( 'NONE', ( #8950, #13032, #29758, #637, #9992, #4843, #28422, #15870, #863, #20586 ) ) ;
#7012=ORIENTED_EDGE ( 'NONE', *, *, #24795, .F. ) ;
#7018=DIRECTION ( 'NONE',  ( 0.000000000000000000, 0.000000000000000000, 1.000000000000000000 ) ) ;
#7025=VERTEX_POINT ( 'NONE', #15102 ) ;
#7039=ORIENTED_EDGE ( 'NONE', *, *, #16041, .T. ) ;
#7059=DIRECTION ( 'NONE',  ( 1.000000000000000000, 0.000000000000000000, 0.000000000000000000 ) ) ;
#7064=CARTESIAN_POINT ( 'NONE',  ( -1.027511273769999933E-13, -27.50000000000000000, 230.0000000000000000 ) ) ;
#7067=VECTOR ( 'NONE', #4422, 1000.000000000000000 ) ;
#7074=CARTESIAN_POINT ( 'NONE',  ( -27.23548387100000312, 3.552713678799999608E-15, 38.33953982530000104 ) ) ;
#7080=CARTESIAN_POINT ( 'NONE',  ( -18.95046173579999760, -18.95046173579999760, 186.7828584120000244 ) ) ;
#7105=CARTESIAN_POINT ( 'NONE',  ( 23.48238834476582326, -12.91648733588402820, 225.9606284813543482 ) ) ;
#7110=CARTESIAN_POINT ( 'NONE',  ( 1.100000000000000089, -27.47799119230000287, 5.000000000000000000 ) ) ;
#7116=ORIENTED_EDGE ( 'NONE', *, *, #26922, .F. ) ;
#7117=CARTESIAN_POINT ( 'NONE',  ( 23.32129337752340348, -14.57293380313067388, 5.556164354324400811 ) ) ;
#7124=VERTEX_POINT ( 'NONE', #31090 ) ;
#7126=DIRECTION ( 'NONE',  ( -0.9316362575375349842, 0.3633921898465292122, -0.000000000000000000 ) ) ;
#7136=ORIENTED_EDGE ( 'NONE', *, *, #27076, .T. ) ;
#7141=CARTESIAN_POINT ( 'NONE',  ( 0.8184510536726904428, -27.48788286177519780, 5.736540937228021164 ) ) ;
#7142=VERTEX_POINT ( 'NONE', #9208 ) ;
#7156=EDGE_CURVE ( 'NONE', #24307, #10785, #14074, .T. ) ;
#7160=CARTESIAN_POINT ( 'NONE',  ( 24.34663841809999951, -12.78636765230000094, 5.000000000000000000 ) ) ;
#7161=ORIENTED_EDGE ( 'NONE', *, *, #5979, .T. ) ;
#7170=DIRECTION ( 'NONE',  ( -0.000000000000000000, -0.000000000000000000, -1.000000000000000000 ) ) ;
#7171=VECTOR ( 'NONE', #9309, 1000.000000000000000 ) ;
#7176=ORIENTED_EDGE ( 'NONE', *, *, #15461, .T. ) ;
#7186=DIRECTION ( 'NONE',  ( 0.000000000000000000, 0.000000000000000000, 1.000000000000000000 ) ) ;
#7194=EDGE_CURVE ( 'NONE', #25472, #27663, #29627, .T. ) ;
#7198=ADVANCED_FACE ( 'NONE', ( #26065 ), #2990, .F. ) ;
#7206=AXIS2_PLACEMENT_3D ( 'NONE', #10700, #10400, #25178 ) ;
#7214=VECTOR ( 'NONE', #19836, 1000.000000000000000 ) ;
#7222=CYLINDRICAL_SURFACE ( 'NONE', #6628, 1.100000000000000089 ) ;
#7225=CARTESIAN_POINT ( 'NONE',  ( 1.087555935787781758, -26.77834284438278090, 224.7819484277976869 ) ) ;
#7227=CIRCLE ( 'NONE', #3769, 27.69999999999999929 ) ;
#7237=CARTESIAN_POINT ( 'NONE',  ( 24.14619884838972297, -13.16136950037729569, 4.119508997699939279 ) ) ;
#7244=DIRECTION ( 'NONE',  ( 0.000000000000000000, 0.000000000000000000, -1.000000000000000000 ) ) ;
#7253=AXIS2_PLACEMENT_3D ( 'NONE', #18486, #21164, #30760 ) ;
#7267=EDGE_CURVE ( 'NONE', #3758, #21856, #28106, .T. ) ;
#7277=ORIENTED_EDGE ( 'NONE', *, *, #5957, .F. ) ;
#7278=CIRCLE ( 'NONE', #12800, 27.50000000000000000 ) ;
#7285=LINE ( 'NONE', #18928, #8932 ) ;
#7287=EDGE_LOOP ( 'NONE', ( #28482, #19702, #16950, #137, #25671 ) ) ;
#7289=DIRECTION ( 'NONE',  ( 0.8660254037843290176, 0.5000000000001899592, 0.000000000000000000 ) ) ;
#7291=AXIS2_PLACEMENT_3D ( 'NONE', #27755, #13755, #20999 ) ;
#7296=CARTESIAN_POINT ( 'NONE',  ( 0.000000000000000000, 0.000000000000000000, 115.0000000000000000 ) ) ;
#7299=DIRECTION ( 'NONE',  ( 0.000000000000000000, 0.000000000000000000, -1.000000000000000000 ) ) ;
#7303=VECTOR ( 'NONE', #12759, 1000.000000000000114 ) ;
#7311=ORIENTED_EDGE ( 'NONE', *, *, #8643, .T. ) ;
#7318=VERTEX_POINT ( 'NONE', #19438 ) ;
#7338=CARTESIAN_POINT ( 'NONE',  ( 23.25782843551338885, -13.31625947593092896, 223.8999999999988404 ) ) ;
#7344=CARTESIAN_POINT ( 'NONE',  ( -0.9242233308569890449, -26.78436826007333238, 225.5979291942194891 ) ) ;
#7351=VERTEX_POINT ( 'NONE', #24474 ) ;
#7358=ORIENTED_EDGE ( 'NONE', *, *, #15081, .T. ) ;
#7371=EDGE_CURVE ( 'NONE', #19781, #20878, #13424, .T. ) ;
#7385=CARTESIAN_POINT ( 'NONE',  ( 9.993285220779503319, -25.61999708228222872, 93.60555127639999284 ) ) ;
#7386=VERTEX_POINT ( 'NONE', #28878 ) ;
#7389=ORIENTED_EDGE ( 'NONE', *, *, #9901, .T. ) ;
#7396=DIRECTION ( 'NONE',  ( 0.000000000000000000, 0.000000000000000000, 1.000000000000000000 ) ) ;
#7401=DIRECTION ( 'NONE',  ( 0.3633921898465292122, 0.9316362575375348731, 0.000000000000000000 ) ) ;
#7405=EDGE_CURVE ( 'NONE', #15775, #24427, #29333, .T. ) ;
#7409=EDGE_CURVE ( 'NONE', #13409, #4540, #15031, .T. ) ;
#7413=CARTESIAN_POINT ( 'NONE',  ( 8.090238276950916685, -26.28358643434115649, 22.68593013736110109 ) ) ;
#7419=DIRECTION ( 'NONE',  ( -0.9316362575375349842, 0.3633921898465292122, -0.000000000000000000 ) ) ;
#7423=ORIENTED_EDGE ( 'NONE', *, *, #5009, .T. ) ;
#7432=DIRECTION ( 'NONE',  ( -0.7071067811865475727, 0.7071067811865475727, 0.000000000000000000 ) ) ;
#7445=FACE_BOUND ( 'NONE', #16309, .T. ) ;
#7446=B_SPLINE_CURVE_WITH_KNOTS ( 'NONE', 3,
 ( #8869, #15961, #25569, #4475, #18474, #1498, #8552, #11400, #4162, #28072 ),
 .UNSPECIFIED., .F., .F.,
 ( 4, 2, 2, 2, 4 ),
 ( 0.000000000000000000, 0.2499999999999998890, 0.4999999999999997780, 0.7499999999999998890, 1.000000000000000000 ),
 .UNSPECIFIED. ) ;
#7449=CARTESIAN_POINT ( 'NONE',  ( 0.8471243414734038746, -27.48706736360548319, 5.703083847462546707 ) ) ;
#7480=PRODUCT_DEFINITION_CONTEXT ( 'detailed design', #15825, 'design' ) ;
#7496=TOROIDAL_SURFACE ( 'NONE', #6482, 24.50000000000000000, 4.000000000000000000 ) ;
#7500=ORIENTED_EDGE ( 'NONE', *, *, #5167, .T. ) ;
#7505=AXIS2_PLACEMENT_3D ( 'NONE', #24274, #7289, #21929 ) ;
#7512=ORIENTED_EDGE ( 'NONE', *, *, #29999, .T. ) ;
#7526=DIRECTION ( 'NONE',  ( -1.000000000000000000, 5.665498452320000818E-16, 0.000000000000000000 ) ) ;
#7529=CARTESIAN_POINT ( 'NONE',  ( 8.903108651239925564, -22.82508830966962421, 90.00000000000000000 ) ) ;
#7532=ADVANCED_FACE ( 'NONE', ( #8705 ), #20574, .F. ) ;
#7537=DIRECTION ( 'NONE',  ( 0.000000000000000000, 0.000000000000000000, 1.000000000000000000 ) ) ;
#7538=EDGE_LOOP ( 'NONE', ( #26363, #5179, #12042, #19040 ) ) ;
#7547=ADVANCED_FACE ( 'NONE', ( #25410 ), #10284, .F. ) ;
#7563=CYLINDRICAL_SURFACE ( 'NONE', #2631, 1.099999999999998979 ) ;
#7565=CARTESIAN_POINT ( 'NONE',  ( 5.654928157491471374, -26.91331636611315403, 20.79580928853452093 ) ) ;
#7570=DIRECTION ( 'NONE',  ( 0.3633921898465292122, 0.9316362575375348731, -5.204170427930420494E-15 ) ) ;
#7574=AXIS2_PLACEMENT_3D ( 'NONE', #10170, #10484, #8254 ) ;
#7576=DIRECTION ( 'NONE',  ( 0.000000000000000000, 0.000000000000000000, 1.000000000000000000 ) ) ;
#7580=DIRECTION ( 'NONE',  ( 1.000000000000000000, -1.224606353819999582E-16, 0.000000000000000000 ) ) ;
#7582=ORIENTED_EDGE ( 'NONE', *, *, #2074, .F. ) ;
#7590=VERTEX_POINT ( 'NONE', #21459 ) ;
#7600=CARTESIAN_POINT ( 'NONE',  ( 27.23548387100000312, -1.776356839399999804E-15, 88.33953982530000815 ) ) ;
#7603=CARTESIAN_POINT ( 'NONE',  ( 27.06563795990000187, -3.314475221579999886E-15, 91.94026860140000679 ) ) ;
#7617=CARTESIAN_POINT ( 'NONE',  ( -1.421085471519999843E-14, -3.552713678799999608E-15, 186.3944487249999895 ) ) ;
#7626=CARTESIAN_POINT ( 'NONE',  ( -27.50000000000000000, 3.552713678799999608E-15, 193.6055512750000105 ) ) ;
#7633=DIRECTION ( 'NONE',  ( 1.000000000000000000, 0.000000000000000000, 0.000000000000000000 ) ) ;
#7636=TOROIDAL_SURFACE ( 'NONE', #19717, 24.50000000000000000, 3.200000000000000178 ) ;
#7643=DIRECTION ( 'NONE',  ( -1.000000000000000000, 5.665498452320000818E-16, 0.000000000000000000 ) ) ;
#7645=CARTESIAN_POINT ( 'NONE',  ( -23.81569860410000317, -13.75000000000000000, 6.099999999630000502 ) ) ;
#7649=DIRECTION ( 'NONE',  ( 1.000000000000000000, 0.000000000000000000, 0.000000000000000000 ) ) ;
#7651=ORIENTED_EDGE ( 'NONE', *, *, #1919, .F. ) ;
#7655=ORIENTED_EDGE ( 'NONE', *, *, #6549, .F. ) ;
#7658=CARTESIAN_POINT ( 'NONE',  ( 23.20948082139999968, -13.40000000000000036, 223.8999999999999773 ) ) ;
#7669=CARTESIAN_POINT ( 'NONE',  ( -2.947640775130000104E-14, -27.50000000000000000, 226.0999999999999943 ) ) ;
#7672=CARTESIAN_POINT ( 'NONE',  ( -9.897162125297919388, -25.37356426550854138, 191.6604601750000256 ) ) ;
#7675=DIRECTION ( 'NONE',  ( 0.000000000000000000, 0.000000000000000000, 1.000000000000000000 ) ) ;
#7691=AXIS2_PLACEMENT_3D ( 'NONE', #12605, #27236, #29284 ) ;
#7708=EDGE_CURVE ( 'NONE', #9708, #12147, #6493, .T. ) ;
#7709=CARTESIAN_POINT ( 'NONE',  ( -14.94562240850000023, -8.628859120750000500, 225.0000000000000000 ) ) ;
#7715=VECTOR ( 'NONE', #3305, 1000.000000000000000 ) ;
#7727=VERTEX_POINT ( 'NONE', #12157 ) ;
#7729=ORIENTED_EDGE ( 'NONE', *, *, #20770, .T. ) ;
#7732=DIRECTION ( 'NONE',  ( 0.000000000000000000, -1.000000000000000000, 0.000000000000000000 ) ) ;
#7737=VECTOR ( 'NONE', #21598, 1000.000000000000000 ) ;
#7748=CARTESIAN_POINT ( 'NONE',  ( -26.80000000069999899, 3.281945028329999726E-15, 143.2171415869999862 ) ) ;
#7754=ADVANCED_FACE ( 'NONE', ( #15752 ), #12529, .T. ) ;
#7757=DIRECTION ( 'NONE',  ( -1.224606353819999829E-16, -1.000000000000000000, 0.000000000000000000 ) ) ;
#7758=AXIS2_PLACEMENT_3D ( 'NONE', #6485, #25698, #14364 ) ;
#7777=CARTESIAN_POINT ( 'NONE',  ( 26.80000000069999899, -3.281945028320000125E-15, 115.0000000010000036 ) ) ;
#7779=CARTESIAN_POINT ( 'NONE',  ( -2.947640775130000104E-14, -27.50000000000000000, 223.8999999999999773 ) ) ;
#7790=EDGE_CURVE ( 'NONE', #14877, #25546, #24604, .T. ) ;
#7796=CARTESIAN_POINT ( 'NONE',  ( 0.2897533057796581324, -27.49881094941897786, 3.928609959452268097 ) ) ;
#7798=CIRCLE ( 'NONE', #9303, 3.200000000000002398 ) ;
#7801=CARTESIAN_POINT ( 'NONE',  ( -7.121574564636396154, -25.83919502053029404, 21.93648921904840776 ) ) ;
#7804=CARTESIAN_POINT ( 'NONE',  ( 24.50000001620000134, -3.000285568839999855E-15, 139.9999999960000139 ) ) ;
#7809=VERTEX_POINT ( 'NONE', #988 ) ;
#7810=CARTESIAN_POINT ( 'NONE',  ( -11.08346179031913437, -28.41490585489481191, 93.60555127549999099 ) ) ;
#7817=CARTESIAN_POINT ( 'NONE',  ( -21.30888436558564081, -16.34772642260385211, 143.2171415880000040 ) ) ;
#7833=CARTESIAN_POINT ( 'NONE',  ( -24.79654435811118063, -10.16723671460306910, 43.21714158839818509 ) ) ;
#7837=ORIENTED_EDGE ( 'NONE', *, *, #29448, .T. ) ;
#7841=ORIENTED_EDGE ( 'NONE', *, *, #20220, .F. ) ;
#7848=EDGE_CURVE ( 'NONE', #2098, #18252, #17261, .T. ) ;
#7850=DIRECTION ( 'NONE',  ( 0.000000000000000000, 0.000000000000000000, -1.000000000000000000 ) ) ;
#7872=CARTESIAN_POINT ( 'NONE',  ( 27.23548386990000125, -3.335274659639999982E-15, 141.6604601740000078 ) ) ;
#7878=ORIENTED_EDGE ( 'NONE', *, *, #380, .F. ) ;
#7883=EDGE_CURVE ( 'NONE', #8486, #902, #8006, .T. ) ;
#7884=DIRECTION ( 'NONE',  ( 1.224606353819999829E-16, 1.000000000000000000, 0.000000000000000000 ) ) ;
#7889=DIRECTION ( 'NONE',  ( 1.000000000000000000, 0.000000000000000000, 0.000000000000000000 ) ) ;
#7894=AXIS2_PLACEMENT_3D ( 'NONE', #19632, #24661, #3095 ) ;
#7895=CARTESIAN_POINT ( 'NONE',  ( 27.23548387180000319, -3.335274659869999873E-15, 41.66046017409999536 ) ) ;
#7898=AXIS2_PLACEMENT_3D ( 'NONE', #18699, #1571, #28298 ) ;
#7903=CARTESIAN_POINT ( 'NONE',  ( -23.53263993751885153, -14.22965940645031324, 224.0404533955600073 ) ) ;
#7907=CARTESIAN_POINT ( 'NONE',  ( 23.24663841809999809, -14.69162354060000020, 225.0000000000000000 ) ) ;
#7908=ORIENTED_EDGE ( 'NONE', *, *, #2133, .F. ) ;
#7918=EDGE_LOOP ( 'NONE', ( #9437, #4379, #17329, #12179 ) ) ;
#7926=EDGE_CURVE ( 'NONE', #7386, #20468, #7, .T. ) ;
#7928=CARTESIAN_POINT ( 'NONE',  ( -24.34663841809999951, -12.78636765230000094, 5.000000000000000000 ) ) ;
#7929=DIRECTION ( 'NONE',  ( 0.9316362575375356503, 0.3633921898465274913, 0.000000000000000000 ) ) ;
#7933=ORIENTED_EDGE ( 'NONE', *, *, #22913, .F. ) ;
#7941=CARTESIAN_POINT ( 'NONE',  ( 26.80000000000000071, -1.776356839399999804E-15, 143.2171415880000040 ) ) ;
#7942=CARTESIAN_POINT ( 'NONE',  ( -7.107063564515523346, -25.84129680694969267, 208.0588908682941565 ) ) ;
#7946=CARTESIAN_POINT ( 'NONE',  ( 0.9895645837522295540, -27.48220350653630817, 4.514327848603801208 ) ) ;
#7948=CYLINDRICAL_SURFACE ( 'NONE', #569, 27.50000000000000000 ) ;
#7949=CARTESIAN_POINT ( 'NONE',  ( -24.76171951330574927, -10.25169584067251094, 93.21714158839991171 ) ) ;
#7960=ORIENTED_EDGE ( 'NONE', *, *, #22021, .T. ) ;
#7961=EDGE_CURVE ( 'NONE', #12226, #7590, #6888, .T. ) ;
#7967=CARTESIAN_POINT ( 'NONE',  ( -23.45048833551293654, -12.97319122232136479, 225.9951937281581706 ) ) ;
#7970=CARTESIAN_POINT ( 'NONE',  ( -24.49999999589999788, 3.000285566369999841E-15, 140.0000000000000000 ) ) ;
#7972=ORIENTED_EDGE ( 'NONE', *, *, #840, .T. ) ;
#7977=CARTESIAN_POINT ( 'NONE',  ( 23.73992238018677270, -12.43607998452291064, 4.902940994718408163 ) ) ;
#7978=DIRECTION ( 'NONE',  ( -0.9316362575375349842, 0.3633921898465292122, -0.000000000000000000 ) ) ;
#7982=CARTESIAN_POINT ( 'NONE',  ( 0.000000000000000000, 0.000000000000000000, 40.00000000000000000 ) ) ;
#7983=CARTESIAN_POINT ( 'NONE',  ( 8.966526567020551397, -25.25634759429104292, 205.5763919674312206 ) ) ;
#7987=CIRCLE ( 'NONE', #30635, 3.000000000000001332 ) ;
#7994=DIRECTION ( 'NONE',  ( 0.000000000000000000, 0.000000000000000000, 1.000000000000000000 ) ) ;
#8006=CIRCLE ( 'NONE', #10516, 3.200000000000000178 ) ;
#8022=ADVANCED_FACE ( 'NONE', ( #3921 ), #2880, .F. ) ;
#8034=CARTESIAN_POINT ( 'NONE',  ( -0.2892551163132154324, -26.79878419087592789, 3.928509618683601712 ) ) ;
#8036=ORIENTED_EDGE ( 'NONE', *, *, #27582, .F. ) ;
#8039=CARTESIAN_POINT ( 'NONE',  ( -1.065814103639999922E-14, 1.421085471519999843E-14, 186.3944487249999895 ) ) ;
#8053=CARTESIAN_POINT ( 'NONE',  ( -0.8790545793981902056, -27.48597397712025980, 5.665333839370780389 ) ) ;
#8059=CARTESIAN_POINT ( 'NONE',  ( 23.56630063259553864, -14.17280417119362035, 224.0051167707288755 ) ) ;
#8062=CARTESIAN_POINT ( 'NONE',  ( 9.738910687886932038, -24.96785170200595161, 193.2171415880000040 ) ) ;
#8074=EDGE_CURVE ( 'NONE', #9436, #30789, #4385, .T. ) ;
#8077=ADVANCED_FACE ( 'NONE', ( #22965 ), #3384, .F. ) ;
#8078=AXIS2_PLACEMENT_3D ( 'NONE', #24490, #15353, #7643 ) ;
#8082=DIRECTION ( 'NONE',  ( -0.8090169943751909232, 0.5877852522921378498, 0.000000000000000000 ) ) ;
#8085=EDGE_CURVE ( 'NONE', #27430, #30479, #27023, .T. ) ;
#8086=CARTESIAN_POINT ( 'NONE',  ( 0.8784916548508220346, -26.78562594433358868, 5.666076087045988530 ) ) ;
#8088=ORIENTED_EDGE ( 'NONE', *, *, #7409, .F. ) ;
#8090=CARTESIAN_POINT ( 'NONE',  ( -22.78981481891096550, -14.10205219198089388, 4.262772992854607423 ) ) ;
#8091=FACE_OUTER_BOUND ( 'NONE', #15434, .T. ) ;
#8093=CARTESIAN_POINT ( 'NONE',  ( -23.32129337776675015, -14.57293380274186134, 4.443835645165135517 ) ) ;
#8095=EDGE_CURVE ( 'NONE', #8882, #6309, #1383, .T. ) ;
#8098=ORIENTED_EDGE ( 'NONE', *, *, #27878, .T. ) ;
#8100=AXIS2_PLACEMENT_3D ( 'NONE', #28036, #28504, #9146 ) ;
#8101=CARTESIAN_POINT ( 'NONE',  ( -8.730899654840367674, -25.33966640892204580, 23.96123044120707846 ) ) ;
#8119=CYLINDRICAL_SURFACE ( 'NONE', #891, 1.099999999999999867 ) ;
#8121=ORIENTED_EDGE ( 'NONE', *, *, #19217, .F. ) ;
#8132=EDGE_CURVE ( 'NONE', #18237, #18212, #28507, .T. ) ;
#8133=CARTESIAN_POINT ( 'NONE',  ( 3.674376064820728427, -26.54820124389934577, 209.8046840415867109 ) ) ;
#8137=ORIENTED_EDGE ( 'NONE', *, *, #21170, .T. ) ;
#8141=DIRECTION ( 'NONE',  ( 0.000000000000000000, 0.000000000000000000, 1.000000000000000000 ) ) ;
#8154=DIRECTION ( 'NONE',  ( 1.000000000000000000, 0.000000000000000000, 0.000000000000000000 ) ) ;
#8156=DIRECTION ( 'NONE',  ( 0.000000000000000000, 0.000000000000000000, 1.000000000000000000 ) ) ;
#8171=ADVANCED_FACE ( 'NONE', ( #9882 ), #20991, .T. ) ;
#8176=AXIS2_PLACEMENT_3D ( 'NONE', #15127, #24578, #667 ) ;
#8180=CIRCLE ( 'NONE', #22775, 27.69999999999999929 ) ;
#8182=CARTESIAN_POINT ( 'NONE',  ( -8.095177325567840754, -26.28419651245281585, 22.67157132346132187 ) ) ;
#8183=VERTEX_POINT ( 'NONE', #14612 ) ;
#8192=CARTESIAN_POINT ( 'NONE',  ( 3.928578988383309323, -27.21916582938554541, 209.8062029264887656 ) ) ;
#8194=VERTEX_POINT ( 'NONE', #4857 ) ;
#8195=AXIS2_PLACEMENT_3D ( 'NONE', #27683, #20610, #12910 ) ;
#8196=ADVANCED_FACE ( 'NONE', ( #12393 ), #12940, .T. ) ;
#8204=DIRECTION ( 'NONE',  ( 0.000000000000000000, 0.000000000000000000, -1.000000000000000000 ) ) ;
#8210=CARTESIAN_POINT ( 'NONE',  ( -14.94562240850000023, -8.628859120750000500, 5.000000000000000000 ) ) ;
#8212=ORIENTED_EDGE ( 'NONE', *, *, #5009, .F. ) ;
#8222=AXIS2_PLACEMENT_3D ( 'NONE', #4537, #23124, #9244 ) ;
#8233=ORIENTED_EDGE ( 'NONE', *, *, #12057, .T. ) ;
#8237=ORIENTED_EDGE ( 'NONE', *, *, #25937, .T. ) ;
#8250=CARTESIAN_POINT ( 'NONE',  ( 22.71519155913117061, -14.22192772740461209, 224.4424652943675937 ) ) ;
#8254=DIRECTION ( 'NONE',  ( 0.8090169943751909232, 0.5877852522921378498, 0.000000000000000000 ) ) ;
#8256=CARTESIAN_POINT ( 'NONE',  ( -9.738910687886855655, -24.96785170200598714, 27.99999999999999645 ) ) ;
#8259=EDGE_CURVE ( 'NONE', #5262, #23982, #9022, .T. ) ;
#8262=CARTESIAN_POINT ( 'NONE',  ( 0.000000000000000000, 0.000000000000000000, 190.0000000000000000 ) ) ;
#8265=EDGE_LOOP ( 'NONE', ( #27781, #1029, #20308, #22611, #2372, #30065, #20942, #31050, #8817, #12537, #9946, #14384, #9980, #27622, #11726, #7908, #8973, #14684, #4174, #22832, #16867, #1119, #2299, #9055, #23858, #1441, #18349, #976, #17784, #14023, #15652, #7423, #27351, #5032, #1868, #2889, #17705, #21604, #24021, #24579, #27495, #21069, #24534, #14403 ) ) ;
#8273=CARTESIAN_POINT ( 'NONE',  ( -25.94284618478185322, -6.948772836044507351, 143.2171415880000040 ) ) ;
#8280=CARTESIAN_POINT ( 'NONE',  ( 27.63177356800000339, -3.383804547859999682E-15, 137.3605236429999934 ) ) ;
#8284=DIRECTION ( 'NONE',  ( -1.000000000000000000, 5.665498452320000818E-16, 0.000000000000000000 ) ) ;
#8286=CARTESIAN_POINT ( 'NONE',  ( 0.000000000000000000, 0.000000000000000000, 140.0000000000000000 ) ) ;
#8290=CARTESIAN_POINT ( 'NONE',  ( 6.076762841307634666, -26.10292173851731690, 208.8288339172677013 ) ) ;
#8292=CARTESIAN_POINT ( 'NONE',  ( -26.79999999999997939, -1.754055898257046664, 43.21714158836666542 ) ) ;
#8304=EDGE_CURVE ( 'NONE', #17178, #13324, #14455, .T. ) ;
#8309=EDGE_CURVE ( 'NONE', #16475, #17862, #21485, .T. ) ;
#8310=DIRECTION ( 'NONE',  ( -0.9316362575375356503, -0.3633921898465275468, 0.000000000000000000 ) ) ;
#8323=CARTESIAN_POINT ( 'NONE',  ( 22.77614505612612206, -14.12431931114201866, 225.7119260791445186 ) ) ;
#8325=DIRECTION ( 'NONE',  ( 1.000000000000000000, 0.000000000000000000, 0.000000000000000000 ) ) ;
#8326=ORIENTED_EDGE ( 'NONE', *, *, #4777, .T. ) ;
#8330=B_SPLINE_CURVE_WITH_KNOTS ( 'NONE', 5,
 ( #20253, #3572, #24524, #24675, #5323, #922 ),
 .UNSPECIFIED., .F., .F.,
 ( 6, 6 ),
 ( 0.000000000000000000, 2.300779717520000212 ),
 .UNSPECIFIED. ) ;
#8335=CARTESIAN_POINT ( 'NONE',  ( -6.965151789112635328, -26.60412671351617320, 21.61051234482303585 ) ) ;
#8348=ORIENTED_EDGE ( 'NONE', *, *, #29638, .T. ) ;
#8349=ADVANCED_FACE ( 'NONE', ( #12860 ), #15521, .F. ) ;
#8350=CARTESIAN_POINT ( 'NONE',  ( -3.552713678799999608E-15, 0.000000000000000000, 193.2171415880000040 ) ) ;
#8361=CARTESIAN_POINT ( 'NONE',  ( 24.08956650215635165, -13.26503430039987919, 224.0404533956383659 ) ) ;
#8363=CARTESIAN_POINT ( 'NONE',  ( 23.34643930356318720, -14.53345043283277782, 224.3574895212763636 ) ) ;
#8364=VERTEX_POINT ( 'NONE', #22764 ) ;
#8371=CARTESIAN_POINT ( 'NONE',  ( 25.94284618478187809, -6.948772836044536660, 186.7828584120000244 ) ) ;
#8372=ORIENTED_EDGE ( 'NONE', *, *, #23999, .F. ) ;
#8377=SURFACE_SIDE_STYLE ('',( #25235 ) ) ;
#8390=CARTESIAN_POINT ( 'NONE',  ( -9.993285220779425160, -25.61999708228226069, 202.0000000000000000 ) ) ;
#8392=ORIENTED_EDGE ( 'NONE', *, *, #7409, .T. ) ;
#8397=CARTESIAN_POINT ( 'NONE',  ( -9.738910687886855655, -24.96785170200598714, 202.0000000000000000 ) ) ;
#8399=AXIS2_PLACEMENT_3D ( 'NONE', #1092, #1569, #8310 ) ;
#8402=ORIENTED_EDGE ( 'NONE', *, *, #752, .T. ) ;
#8403=ADVANCED_FACE ( 'NONE', ( #27025 ), #8119, .F. ) ;
#8404=CARTESIAN_POINT ( 'NONE',  ( 0.000000000000000000, 0.000000000000000000, 93.60555127639999284 ) ) ;
#8411=CARTESIAN_POINT ( 'NONE',  ( -23.88846875309505080, -13.62395840461769225, 226.1000000000000227 ) ) ;
#8414=CARTESIAN_POINT ( 'NONE',  ( 0.000000000000000000, 0.000000000000000000, 141.6604601749999972 ) ) ;
#8420=ORIENTED_EDGE ( 'NONE', *, *, #3470, .T. ) ;
#8421=ADVANCED_FACE ( 'NONE', ( #23092 ), #21983, .F. ) ;
#8427=TOROIDAL_SURFACE ( 'NONE', #24513, 29.80000000000000071, 3.000000000000000000 ) ;
#8428=CARTESIAN_POINT ( 'NONE',  ( 10.06596365874881194, -25.80632433378973900, 190.0000000000000000 ) ) ;
#8432=DIRECTION ( 'NONE',  ( 1.000000000000000000, -1.224606353819998843E-16, 0.000000000000000000 ) ) ;
#8445=CARTESIAN_POINT ( 'NONE',  ( -23.82266443414332002, -12.31939917416737096, 43.21714158843889919 ) ) ;
#8449=CARTESIAN_POINT ( 'NONE',  ( 23.81569860410000317, -13.75000000000000000, 226.0999999999999943 ) ) ;
#8461=DIRECTION ( 'NONE',  ( 0.000000000000000000, 0.000000000000000000, -1.000000000000000000 ) ) ;
#8462=DIRECTION ( 'NONE',  ( 0.000000000000000000, 0.000000000000000000, 1.000000000000000000 ) ) ;
#8465=DIRECTION ( 'NONE',  ( 1.000000000000000000, 0.000000000000000000, 0.000000000000000000 ) ) ;
#8486=VERTEX_POINT ( 'NONE', #8428 ) ;
#8488=CYLINDRICAL_SURFACE ( 'NONE', #26329, 1.099999999999998979 ) ;
#8492=ORIENTED_EDGE ( 'NONE', *, *, #3778, .F. ) ;
#8504=CYLINDRICAL_SURFACE ( 'NONE', #3474, 26.80000000000002203 ) ;
#8508=VERTEX_POINT ( 'NONE', #18973 ) ;
#8537=ORIENTED_EDGE ( 'NONE', *, *, #12640, .F. ) ;
#8538=CARTESIAN_POINT ( 'NONE',  ( 24.34663841809999951, -12.78636765230000094, 5.000000000000000000 ) ) ;
#8546=CARTESIAN_POINT ( 'NONE',  ( -0.8355090854489903851, -26.78702287505212709, 224.2806846201137887 ) ) ;
#8552=CARTESIAN_POINT ( 'NONE',  ( 25.94284618478187809, -6.948772836044536660, 136.7828584120000244 ) ) ;
#8564=CARTESIAN_POINT ( 'NONE',  ( 27.54391552369999729, -3.373045395939999845E-15, 142.9562530130000084 ) ) ;
#8567=CARTESIAN_POINT ( 'NONE',  ( 10.82908725742651512, -27.76276047461856322, 93.21714158839999698 ) ) ;
#8570=CARTESIAN_POINT ( 'NONE',  ( -24.14619884830422336, -13.16136950053335752, 225.8804910025767185 ) ) ;
#8574=CARTESIAN_POINT ( 'NONE',  ( 27.50000000000000000, -1.776356839399999804E-15, 136.3944487250000179 ) ) ;
#8591=CARTESIAN_POINT ( 'NONE',  ( -1.027511273769999933E-13, -27.50000000000000000, 115.0000000000000000 ) ) ;
#8592=CARTESIAN_POINT ( 'NONE',  ( -24.49999999589999788, 3.000285566369999841E-15, 140.0000000000000000 ) ) ;
#8596=CIRCLE ( 'NONE', #26710, 27.23548387060000309 ) ;
#8623=CARTESIAN_POINT ( 'NONE',  ( -0.8184510532230938606, -27.48788286177401474, 4.263459062314771231 ) ) ;
#8627=DIRECTION ( 'NONE',  ( 0.7071067811865475727, 0.7071067811865475727, 0.000000000000000000 ) ) ;
#8628=EDGE_CURVE ( 'NONE', #2523, #12147, #5229, .T. ) ;
#8632=VECTOR ( 'NONE', #20526, 1000.000000000000000 ) ;
#8637=LINE ( 'NONE', #16198, #20771 ) ;
#8638=CARTESIAN_POINT ( 'NONE',  ( 22.68420274108862245, -14.27219891852400302, 225.4229804109004931 ) ) ;
#8643=EDGE_CURVE ( 'NONE', #24657, #17664, #14970, .T. ) ;
#8647=CARTESIAN_POINT ( 'NONE',  ( -23.16113320663907160, -13.48374052519065813, 223.9000000000012562 ) ) ;
#8649=CARTESIAN_POINT ( 'NONE',  ( 0.09707315090956633585, -26.79999999950001310, 3.899999999999991473 ) ) ;
#8653=ORIENTED_EDGE ( 'NONE', *, *, #27360, .F. ) ;
#8656=ORIENTED_EDGE ( 'NONE', *, *, #29853, .T. ) ;
#8657=CARTESIAN_POINT ( 'NONE',  ( -23.24663841809999809, -14.69162354060000020, 225.0000000000000000 ) ) ;
#8666=CARTESIAN_POINT ( 'NONE',  ( -26.80000000000000071, 6.217248937899999413E-15, 136.7828584120000244 ) ) ;
#8667=CARTESIAN_POINT ( 'NONE',  ( 23.48532359031332462, -12.91116100182251714, 5.957452580039663381 ) ) ;
#8672=CARTESIAN_POINT ( 'NONE',  ( -9.799563951679274965, -25.69477015992461233, 203.8298458494338661 ) ) ;
#8688=DIRECTION ( 'NONE',  ( 0.3633921898465274913, -0.9316362575375355393, 0.000000000000000000 ) ) ;
#8693=CARTESIAN_POINT ( 'NONE',  ( 24.34660549313368705, -12.78643034496831277, 4.854326830101610923 ) ) ;
#8705=FACE_OUTER_BOUND ( 'NONE', #17782, .T. ) ;
#8706=VECTOR ( 'NONE', #11011, 1000.000000000000000 ) ;
#8717=CARTESIAN_POINT ( 'NONE',  ( -22.64694720645078263, -14.33102249094126890, 4.781948427652641165 ) ) ;
#8718=DIRECTION ( 'NONE',  ( 0.7071067811865475727, -0.7071067811865475727, 0.000000000000000000 ) ) ;
#8724=AXIS2_PLACEMENT_3D ( 'NONE', #30888, #24117, #2555 ) ;
#8725=EDGE_LOOP ( 'NONE', ( #19863, #11853, #30126, #7655 ) ) ;
#8730=TOROIDAL_SURFACE ( 'NONE', #30843, 24.50000000000000000, 4.000000000000000000 ) ;
#8734=CARTESIAN_POINT ( 'NONE',  ( -24.34660549313262834, -12.78643034497033781, 225.1456731698328895 ) ) ;
#8738=VERTEX_POINT ( 'NONE', #9234 ) ;
#8748=VECTOR ( 'NONE', #8204, 1000.000000000000000 ) ;
#8762=CARTESIAN_POINT ( 'NONE',  ( -1.071601127040515022, -27.47917021046086106, 225.2867514115019674 ) ) ;
#8768=AXIS2_PLACEMENT_3D ( 'NONE', #5704, #17655, #20337 ) ;
#8770=AXIS2_PLACEMENT_3D ( 'NONE', #9488, #21455, #12005 ) ;
#8776=ORIENTED_EDGE ( 'NONE', *, *, #14020, .F. ) ;
#8786=DIRECTION ( 'NONE',  ( 0.000000000000000000, 0.000000000000000000, 1.000000000000000000 ) ) ;
#8790=CARTESIAN_POINT ( 'NONE',  ( 0.000000000000000000, 0.000000000000000000, 90.00000000000000000 ) ) ;
#8796=B_SPLINE_CURVE_WITH_KNOTS ( 'NONE', 3,
 ( #2019, #1553, #18377, #11609, #21206, #27973, #6417, #9233, #18841, #13657 ),
 .UNSPECIFIED., .F., .F.,
 ( 4, 2, 2, 2, 4 ),
 ( 0.000000000000000000, 0.2500000000000000000, 0.5000000000000000000, 0.7500000000000000000, 1.000000000000000000 ),
 .UNSPECIFIED. ) ;
#8806=EDGE_CURVE ( 'NONE', #2098, #29682, #20486, .T. ) ;
#8811=CARTESIAN_POINT ( 'NONE',  ( 0.9876146829922234360, -26.78228247995595979, 4.508624923504668480 ) ) ;
#8812=VERTEX_POINT ( 'NONE', #19156 ) ;
#8816=EDGE_LOOP ( 'NONE', ( #26893, #29941, #17028, #29591 ) ) ;
#8817=ORIENTED_EDGE ( 'NONE', *, *, #27081, .T. ) ;
#8844=CARTESIAN_POINT ( 'NONE',  ( -6.726015838937419389, -25.94607852067422016, 21.60652066236992752 ) ) ;
#8857=ORIENTED_EDGE ( 'NONE', *, *, #8304, .T. ) ;
#8862=CARTESIAN_POINT ( 'NONE',  ( -1.100000000000000089, -26.77741585740000119, 225.0000000000000000 ) ) ;
#8869=CARTESIAN_POINT ( 'NONE',  ( 18.95046173579999760, -18.95046173579999760, 136.7828584120000244 ) ) ;
#8870=ADVANCED_FACE ( 'NONE', ( #24805 ), #13966, .T. ) ;
#8878=CARTESIAN_POINT ( 'NONE',  ( 22.71671780426621723, -14.21943167003267838, 4.451031837088323506 ) ) ;
#8882=VERTEX_POINT ( 'NONE', #8574 ) ;
#8885=B_SPLINE_CURVE_WITH_KNOTS ( 'NONE', 3,
 ( #10894, #20803, #4121, #8672, #3965, #28032, #25529, #18271, #11361, #1771, #20485, #28346, #6477, #27714, #27881, #18592, #13400, #13563, #1459, #8992, #6160, #18112, #25374, #6326, #16078, #28188 ),
 .UNSPECIFIED., .F., .F.,
 ( 4, 2, 2, 2, 2, 2, 2, 2, 2, 2, 2, 2, 4 ),
 ( 0.000000000000000000, 0.001576069497370726673, 0.002364104246056131318, 0.003152138994741535746, 0.004728208492112424832, 0.005516243240797868291, 0.006304277989483312618, 0.007880347486854262853, 0.008668382235539714986, 0.009456416984225165384, 0.01024445173291061752, 0.01103248648159606791, 0.01260855597896695483 ),
 .UNSPECIFIED. ) ;
#8887=EDGE_CURVE ( 'NONE', #31042, #17004, #15508, .T. ) ;
#8892=EDGE_CURVE ( 'NONE', #24657, #25641, #405, .T. ) ;
#8899=DIRECTION ( 'NONE',  ( 1.224606353819999829E-16, 1.000000000000000000, 0.000000000000000000 ) ) ;
#8904=CARTESIAN_POINT ( 'NONE',  ( -26.80000000000000071, 9.769962616700000205E-15, 186.7828584120000244 ) ) ;
#8913=CARTESIAN_POINT ( 'NONE',  ( 10.82908725742652933, -27.76276047461856322, 36.78285841159999592 ) ) ;
#8917=CARTESIAN_POINT ( 'NONE',  ( 9.738910687886868089, -24.96785170200598358, 115.0000000000000000 ) ) ;
#8932=VECTOR ( 'NONE', #16872, 1000.000000000000000 ) ;
#8939=ORIENTED_EDGE ( 'NONE', *, *, #16011, .T. ) ;
#8941=ORIENTED_EDGE ( 'NONE', *, *, #6964, .F. ) ;
#8943=CARTESIAN_POINT ( 'NONE',  ( -9.993285220779425160, -25.61999708228226069, 36.39444872359999295 ) ) ;
#8946=CARTESIAN_POINT ( 'NONE',  ( 3.466821295769682159E-14, -2.890242878314739659E-13, 277.5163816122566800 ) ) ;
#8947=CARTESIAN_POINT ( 'NONE',  ( -7.105427357599999217E-15, 7.105427357599999217E-15, 86.39444872449999480 ) ) ;
#8950=ORIENTED_EDGE ( 'NONE', *, *, #29279, .F. ) ;
#8960=DIRECTION ( 'NONE',  ( -0.9316362575375349842, 0.3633921898465292122, -0.000000000000000000 ) ) ;
#8968=LINE ( 'NONE', #30059, #15835 ) ;
#8972=DIRECTION ( 'NONE',  ( 0.9316362575375356503, 0.3633921898465274913, 0.000000000000000000 ) ) ;
#8973=ORIENTED_EDGE ( 'NONE', *, *, #26458, .T. ) ;
#8986=CARTESIAN_POINT ( 'NONE',  ( 23.35305511532094869, -13.14889042229386895, 6.071490516007937543 ) ) ;
#8992=CARTESIAN_POINT ( 'NONE',  ( -4.941595660341803864, -27.05346828916500712, 209.5085898789650116 ) ) ;
#8997=EDGE_CURVE ( 'NONE', #17381, #17245, #22001, .T. ) ;
#9008=EDGE_LOOP ( 'NONE', ( #577, #18886, #10497, #15515 ) ) ;
#9010=PLANE ( 'NONE',  #13789 ) ;
#9018=EDGE_CURVE ( 'NONE', #12383, #23813, #30772, .T. ) ;
#9022=B_SPLINE_CURVE_WITH_KNOTS ( 'NONE', 5,
 ( #21385, #16958, #19172, #26712, #14761, #19013 ),
 .UNSPECIFIED., .F., .F.,
 ( 6, 6 ),
 ( -2.300779731039999998, 0.000000000000000000 ),
 .UNSPECIFIED. ) ;
#9030=FACE_OUTER_BOUND ( 'NONE', #23593, .T. ) ;
#9041=CARTESIAN_POINT ( 'NONE',  ( -27.50000000000000000, 3.367667473009999970E-15, 230.0000000000000000 ) ) ;
#9055=ORIENTED_EDGE ( 'NONE', *, *, #2018, .T. ) ;
#9061=CARTESIAN_POINT ( 'NONE',  ( -26.84464185210000053, 3.287411897809999814E-15, 187.4375040470000044 ) ) ;
#9065=EDGE_CURVE ( 'NONE', #17448, #12078, #2235, .T. ) ;
#9069=DIRECTION ( 'NONE',  ( 0.000000000000000000, 0.000000000000000000, 1.000000000000000000 ) ) ;
#9073=CARTESIAN_POINT ( 'NONE',  ( -4.130757957910000097E-10, -1.288485762530000039E-09, 230.0000000000000000 ) ) ;
#9079=EDGE_CURVE ( 'NONE', #16428, #21606, #16597, .T. ) ;
#9084=CARTESIAN_POINT ( 'NONE',  ( -24.34663841808528062, -12.78636765232545969, 224.9035402871930387 ) ) ;
#9120=CARTESIAN_POINT ( 'NONE',  ( 0.9003580991302461145, -26.78512134311359105, 4.366512425711518652 ) ) ;
#9122=DIRECTION ( 'NONE',  ( 0.000000000000000000, 0.000000000000000000, 1.000000000000000000 ) ) ;
#9123=EDGE_LOOP ( 'NONE', ( #21845, #28690, #5857, #28016 ) ) ;
#9144=CARTESIAN_POINT ( 'NONE',  ( -23.67414648238567665, -12.56096907814344732, 224.4424652941504235 ) ) ;
#9146=DIRECTION ( 'NONE',  ( 1.000000000000000000, 0.000000000000000000, 0.000000000000000000 ) ) ;
#9157=ORIENTED_EDGE ( 'NONE', *, *, #3684, .T. ) ;
#9161=ORIENTED_EDGE ( 'NONE', *, *, #29031, .T. ) ;
#9171=B_SPLINE_CURVE_WITH_KNOTS ( 'NONE', 5,
 ( #24866, #15256, #27064, #10084, #28961, #799 ),
 .UNSPECIFIED., .F., .F.,
 ( 6, 6 ),
 ( 0.000000000000000000, 2.300779653749999820 ),
 .UNSPECIFIED. ) ;
#9178=CARTESIAN_POINT ( 'NONE',  ( 18.95046173579999760, -18.95046173579999760, -2.842170943039999687E-14 ) ) ;
#9180=CIRCLE ( 'NONE', #16219, 4.000000000000000888 ) ;
#9184=FACE_BOUND ( 'NONE', #21498, .T. ) ;
#9185=CARTESIAN_POINT ( 'NONE',  ( 9.221751571650358414, -25.90851042236079849, 24.42522152380284339 ) ) ;
#9186=B_SPLINE_CURVE_WITH_KNOTS ( 'NONE', 3,
 ( #20530, #3855, #13444, #6524, #16122, #30756, #12131, #9185, #21160, #190, #351, #7413, #6675, #9780, #11406, #9934, #24105, #7565, #2545, #26612, #16273, #19538, #21905, #19381, #14662, #29121 ),
 .UNSPECIFIED., .F., .F.,
 ( 4, 2, 2, 2, 2, 2, 2, 2, 2, 2, 2, 2, 4 ),
 ( 0.000000000000000000, 0.001576069497370868920, 0.002364104246056298285, 0.003152138994741727866, 0.004728208492112593968, 0.005516243240798030488, 0.006304277989483467008, 0.007880347486854335712, 0.008668382235539772232, 0.009456416984225208752, 0.01024445173291064354, 0.01103248648159608006, 0.01260855597896695136 ),
 .UNSPECIFIED. ) ;
#9191=ORIENTED_EDGE ( 'NONE', *, *, #668, .T. ) ;
#9192=DIRECTION ( 'NONE',  ( -1.000000000000000000, 0.000000000000000000, 0.000000000000000000 ) ) ;
#9199=EDGE_LOOP ( 'NONE', ( #15875, #13895, #8402, #21682, #24076, #10186, #26136, #1405, #26354, #20300 ) ) ;
#9204=EDGE_CURVE ( 'NONE', #5609, #15947, #911, .T. ) ;
#9208=CARTESIAN_POINT ( 'NONE',  ( 27.23548387100000312, -1.776356839399999804E-15, 88.33953982530000815 ) ) ;
#9209=SURFACE_SIDE_STYLE ('',( #18656 ) ) ;
#9215=DIRECTION ( 'NONE',  ( -1.000000000000000000, 5.665498452320000818E-16, 0.000000000000000000 ) ) ;
#9217=CARTESIAN_POINT ( 'NONE',  ( 0.9891023284355177081, -26.78175549087869101, 225.4866061618205606 ) ) ;
#9218=TOROIDAL_SURFACE ( 'NONE', #13770, 24.50000000000000000, 3.200000000000000178 ) ;
#9221=ADVANCED_FACE ( 'NONE', ( #407 ), #23037, .F. ) ;
#9230=DIRECTION ( 'NONE',  ( -1.000000000000000000, 1.224606353819999829E-16, 0.000000000000000000 ) ) ;
#9233=CARTESIAN_POINT ( 'NONE',  ( -0.2182390032459076146, -27.49908342132812322, 223.9122931967829970 ) ) ;
#9234=CARTESIAN_POINT ( 'NONE',  ( 9.738910687886932038, -24.96785170200595161, 93.21714158839999698 ) ) ;
#9235=EDGE_CURVE ( 'NONE', #12069, #13409, #11946, .T. ) ;
#9237=AXIS2_PLACEMENT_3D ( 'NONE', #3895, #4205, #2010 ) ;
#9239=AXIS2_PLACEMENT_3D ( 'NONE', #30727, #11531, #21132 ) ;
#9240=AXIS2_PLACEMENT_3D ( 'NONE', #6522, #23378, #18478 ) ;
#9242=DIRECTION ( 'NONE',  ( 0.000000000000000000, 0.000000000000000000, -1.000000000000000000 ) ) ;
#9243=ORIENTED_EDGE ( 'NONE', *, *, #20954, .T. ) ;
#9244=DIRECTION ( 'NONE',  ( 1.000000000000000000, -1.224606353819999582E-16, 0.000000000000000000 ) ) ;
#9250=CARTESIAN_POINT ( 'NONE',  ( -3.552713678799999608E-15, 0.000000000000000000, 36.39444872449999480 ) ) ;
#9260=AXIS2_PLACEMENT_3D ( 'NONE', #26616, #24109, #14668 ) ;
#9261=CARTESIAN_POINT ( 'NONE',  ( -0.09707459578013553914, -26.79999999950000955, 6.099999999999997868 ) ) ;
#9269=FACE_OUTER_BOUND ( 'NONE', #1206, .T. ) ;
#9277=CYLINDRICAL_SURFACE ( 'NONE', #13697, 26.80000000000002203 ) ;
#9282=ORIENTED_EDGE ( 'NONE', *, *, #1741, .T. ) ;
#9283=EDGE_CURVE ( 'NONE', #28570, #24922, #26533, .T. ) ;
#9286=CARTESIAN_POINT ( 'NONE',  ( -1.421085471519999843E-14, -1.421085471519999843E-14, 87.93968498540000667 ) ) ;
#9302=DIRECTION ( 'NONE',  ( -0.8660254037843290176, 0.5000000000001899592, -1.018673689593249976E-32 ) ) ;
#9303=AXIS2_PLACEMENT_3D ( 'NONE', #12624, #22086, #15303 ) ;
#9309=DIRECTION ( 'NONE',  ( 0.000000000000000000, 0.000000000000000000, -1.000000000000000000 ) ) ;
#9338=CARTESIAN_POINT ( 'NONE',  ( 2.107992564109750333, -27.41908764619381245, 20.00000000000000355 ) ) ;
#9344=CARTESIAN_POINT ( 'NONE',  ( 22.63996098036280458, -14.34127493679882903, 4.854121447380539855 ) ) ;
#9357=CARTESIAN_POINT ( 'NONE',  ( 9.993285220779439371, -25.61999708228226069, 115.0000000000000000 ) ) ;
#9359=ORIENTED_EDGE ( 'NONE', *, *, #24049, .F. ) ;
#9375=EDGE_CURVE ( 'NONE', #20468, #12912, #427, .T. ) ;
#9376=CARTESIAN_POINT ( 'NONE',  ( -9.897162125400486232, -25.37356426577148127, 38.33953982530000104 ) ) ;
#9381=DIRECTION ( 'NONE',  ( 0.3633921898465291567, 0.9316362575375349842, 0.000000000000000000 ) ) ;
#9385=CIRCLE ( 'NONE', #27986, 3.200000000000000178 ) ;
#9388=CARTESIAN_POINT ( 'NONE',  ( 0.000000000000000000, 0.000000000000000000, 136.3944487260000074 ) ) ;
#9389=B_SPLINE_CURVE_WITH_KNOTS ( 'NONE', 3,
 ( #6965, #11535, #19080, #7117, #26470, #26623, #26164, #17023, #21602, #21442 ),
 .UNSPECIFIED., .F., .F.,
 ( 4, 2, 2, 2, 4 ),
 ( 0.000000000000000000, 0.2500000000000000000, 0.5000000000000000000, 0.7500000000000000000, 1.000000000000000000 ),
 .UNSPECIFIED. ) ;
#9391=ORIENTED_EDGE ( 'NONE', *, *, #11633, .T. ) ;
#9397=VERTEX_POINT ( 'NONE', #25237 ) ;
#9401=DIRECTION ( 'NONE',  ( -1.000000000000000000, 1.224606353819999829E-16, 0.000000000000000000 ) ) ;
#9402=DIRECTION ( 'NONE',  ( 0.000000000000000000, 0.000000000000000000, -1.000000000000000000 ) ) ;
#9408=CARTESIAN_POINT ( 'NONE',  ( 9.738910687886868089, -24.96785170200598358, 202.0000000000000000 ) ) ;
#9409=CARTESIAN_POINT ( 'NONE',  ( 0.000000000000000000, 0.000000000000000000, 40.00000000000000000 ) ) ;
#9418=CARTESIAN_POINT ( 'NONE',  ( 27.50000000000000000, -3.367667472999999580E-15, 193.6055512739999926 ) ) ;
#9421=B_SPLINE_CURVE_WITH_KNOTS ( 'NONE', 3,
 ( #29551, #8292, #10520, #3578, #17585, #17887, #22782, #27346, #29857, #1233, #10834, #7833, #12713, #5791, #27195, #5633, #20420, #30012, #8445, #29707, #17435, #24986, #13023, #18045, #10366, #22633 ),
 .UNSPECIFIED., .F., .F.,
 ( 4, 2, 2, 2, 1, 1, 1, 1, 1, 1, 2, 2, 2, 2, 2, 4 ),
 ( 0.000000000000000000, 0.2499999999999553690, 0.3749999999999330536, 0.4374999999999219513, 0.4687499999999163447, 0.4843749999999137912, 0.4921874999999124034, 0.4960937499999118483, 0.4980468749999114042, 0.4990234374999112377, 0.4995117187499112932, 0.4999999999999112932, 0.6249999999999333866, 0.7499999999999554801, 0.8749999999999776845, 1.000000000000000000 ),
 .UNSPECIFIED. ) ;
#9423=CARTESIAN_POINT ( 'NONE',  ( -23.61599683758278800, -12.66993935690586959, 4.280684604083014655 ) ) ;
#9427=VECTOR ( 'NONE', #1520, 1000.000000000000000 ) ;
#9432=ORIENTED_EDGE ( 'NONE', *, *, #16742, .T. ) ;
#9434=CARTESIAN_POINT ( 'NONE',  ( -25.94284618478186744, -6.948772836044545542, 186.7828584126666840 ) ) ;
#9435=DIRECTION ( 'NONE',  ( 1.000000000000000000, 0.000000000000000000, 0.000000000000000000 ) ) ;
#9436=VERTEX_POINT ( 'NONE', #10918 ) ;
#9437=ORIENTED_EDGE ( 'NONE', *, *, #8997, .F. ) ;
#9441=FACE_OUTER_BOUND ( 'NONE', #1374, .T. ) ;
#9443=ORIENTED_EDGE ( 'NONE', *, *, #28292, .F. ) ;
#9445=CARTESIAN_POINT ( 'NONE',  ( 7.453090060300409547, -2.907137518772282991, 20.00000000000000000 ) ) ;
#9446=CARTESIAN_POINT ( 'NONE',  ( 24.49999999589999788, -3.000285566359999846E-15, 140.0000000000000000 ) ) ;
#9458=VECTOR ( 'NONE', #17610, 1000.000000000000000 ) ;
#9459=ADVANCED_FACE ( 'NONE', ( #6656 ), #6942, .F. ) ;
#9460=CARTESIAN_POINT ( 'NONE',  ( 23.63672937736964030, -12.63153181622180554, 225.6766013745815940 ) ) ;
#9469=CARTESIAN_POINT ( 'NONE',  ( -9.993285220779545952, -25.61999708228220740, 93.60555127549999099 ) ) ;
#9485=CARTESIAN_POINT ( 'NONE',  ( 26.84464184930000030, -3.287411897459999980E-15, 37.43750406050000379 ) ) ;
#9488=CARTESIAN_POINT ( 'NONE',  ( 0.000000000000000000, 0.000000000000000000, 192.0603150150000147 ) ) ;
#9501=CARTESIAN_POINT ( 'NONE',  ( 0.9007122719980839021, -27.48548889903062431, 5.632980212606629955 ) ) ;
#9503=DIRECTION ( 'NONE',  ( -0.9316362575375349842, 0.3633921898465292122, -0.000000000000000000 ) ) ;
#9505=CARTESIAN_POINT ( 'NONE',  ( 26.80000000000000071, -3.552713678799999608E-15, 93.21714158839999698 ) ) ;
#9506=EDGE_CURVE ( 'NONE', #24116, #13582, #20674, .T. ) ;
#9511=DIRECTION ( 'NONE',  ( 0.000000000000000000, 0.000000000000000000, 1.000000000000000000 ) ) ;
#9523=EDGE_LOOP ( 'NONE', ( #22714, #27501, #6366, #6233 ) ) ;
#9524=DIRECTION ( 'NONE',  ( 0.000000000000000000, 0.000000000000000000, 1.000000000000000000 ) ) ;
#9526=VERTEX_POINT ( 'NONE', #19240 ) ;
#9529=CIRCLE ( 'NONE', #20085, 27.23548387100000312 ) ;
#9531=B_SPLINE_CURVE_WITH_KNOTS ( 'NONE', 3,
 ( #8538, #8693, #18301, #6347, #21714, #7237, #12105, #5335, #26588, #22174 ),
 .UNSPECIFIED., .F., .F.,
 ( 4, 2, 2, 2, 4 ),
 ( 0.000000000000000000, 0.2500000000000000000, 0.5000000000000000000, 0.7500000000000000000, 1.000000000000000000 ),
 .UNSPECIFIED. ) ;
#9551=CARTESIAN_POINT ( 'NONE',  ( -26.79999999999999361, -1.754055898257055324, 93.21714158836665831 ) ) ;
#9552=LINE ( 'NONE', #21673, #21863 ) ;
#9555=CARTESIAN_POINT ( 'NONE',  ( -1.100000000000000089, -27.47799119300000115, 225.0000000000000000 ) ) ;
#9563=ORIENTED_EDGE ( 'NONE', *, *, #24459, .T. ) ;
#9568=ADVANCED_FACE ( 'NONE', ( #2411 ), #14681, .F. ) ;
#9569=DIRECTION ( 'NONE',  ( 1.000000000000000000, -1.224606353819999582E-16, 0.000000000000000000 ) ) ;
#9579=AXIS2_PLACEMENT_3D ( 'NONE', #14605, #28914, #12227 ) ;
#9584=CARTESIAN_POINT ( 'NONE',  ( 0.000000000000000000, -17.25771824150000100, 225.0000000000000000 ) ) ;
#9590=CARTESIAN_POINT ( 'NONE',  ( -26.79999999999999361, 3.901323708532900174E-14, 37.32841481368520675 ) ) ;
#9591=ORIENTED_EDGE ( 'NONE', *, *, #10857, .F. ) ;
#9598=ORIENTED_EDGE ( 'NONE', *, *, #1596, .T. ) ;
#9600=AXIS2_PLACEMENT_3D ( 'NONE', #5128, #16623, #2011 ) ;
#9606=EDGE_CURVE ( 'NONE', #4699, #4261, #18327, .T. ) ;
#9613=ORIENTED_EDGE ( 'NONE', *, *, #6230, .F. ) ;
#9622=DIRECTION ( 'NONE',  ( 0.000000000000000000, 0.000000000000000000, -1.000000000000000000 ) ) ;
#9653=CARTESIAN_POINT ( 'NONE',  ( 7.105427357599999217E-15, 0.000000000000000000, 136.3944487250000179 ) ) ;
#9666=CARTESIAN_POINT ( 'NONE',  ( 27.92857142909999979, -3.420150602509999660E-15, 187.9396849849999853 ) ) ;
#9673=ADVANCED_FACE ( 'NONE', ( #9954 ), #31052, .T. ) ;
#9679=ADVANCED_FACE ( 'NONE', ( #29139 ), #15133, .T. ) ;
#9682=CARTESIAN_POINT ( 'NONE',  ( -24.34131725939277757, -12.79741914669601144, 4.782075047738786999 ) ) ;
#9690=CARTESIAN_POINT ( 'NONE',  ( 0.000000000000000000, 0.000000000000000000, 140.0000000000000000 ) ) ;
#9691=CARTESIAN_POINT ( 'NONE',  ( -6.394884621839999216E-14, -26.80000000000000071, 226.0999999999999943 ) ) ;
#9698=CARTESIAN_POINT ( 'NONE',  ( -1.100000000000000311, -26.77741585740000474, 225.0970590044875621 ) ) ;
#9708=VERTEX_POINT ( 'NONE', #5838 ) ;
#9711=VERTEX_POINT ( 'NONE', #24894 ) ;
#9712=EDGE_CURVE ( 'NONE', #31042, #2824, #16482, .T. ) ;
#9718=CIRCLE ( 'NONE', #12749, 3.000000000000001332 ) ;
#9722=DIRECTION ( 'NONE',  ( -1.000000000000000000, 5.665498452320000818E-16, 0.000000000000000000 ) ) ;
#9725=B_SPLINE_CURVE_WITH_KNOTS ( 'NONE', 3,
 ( #17125, #5164, #7225, #28937, #24528, #12097, #2968, #17278, #26579, #474, #14774, #5019, #19184, #24376 ),
 .UNSPECIFIED., .F., .F.,
 ( 4, 2, 2, 2, 2, 2, 4 ),
 ( 0.000000000000000000, 0.2499999999999525935, 0.3749999999999519273, 0.4374999999999515943, 0.4999999999999513722, 0.7499999999999755751, 1.000000000000000000 ),
 .UNSPECIFIED. ) ;
#9732=CARTESIAN_POINT ( 'NONE',  ( 27.63177371719999798, -3.383804566139999704E-15, 192.6394760450000092 ) ) ;
#9741=DIRECTION ( 'NONE',  ( 0.000000000000000000, -1.000000000000000000, 0.000000000000000000 ) ) ;
#9744=VECTOR ( 'NONE', #25158, 1000.000000000000000 ) ;
#9773=AXIS2_PLACEMENT_3D ( 'NONE', #30325, #15852, #8432 ) ;
#9780=CARTESIAN_POINT ( 'NONE',  ( 7.379546049855187029, -26.49401563815924376, 21.93856359977218418 ) ) ;
#9794=AXIS2_PLACEMENT_3D ( 'NONE', #1110, #29899, #8325 ) ;
#9798=EDGE_LOOP ( 'NONE', ( #400, #28977, #21067, #20511 ) ) ;
#9805=DIRECTION ( 'NONE',  ( 1.000000000000000000, 0.000000000000000000, 0.000000000000000000 ) ) ;
#9807=AXIS2_PLACEMENT_3D ( 'NONE', #27144, #3525, #22428 ) ;
#9814=CARTESIAN_POINT ( 'NONE',  ( 27.50000000000000000, -3.367667472999999580E-15, 115.0000000010000036 ) ) ;
#9818=CARTESIAN_POINT ( 'NONE',  ( 22.78981481966842182, -14.10205219082176065, 5.737227008641060166 ) ) ;
#9819=CARTESIAN_POINT ( 'NONE',  ( 1.065814103639999922E-14, 0.000000000000000000, 36.78285841159999592 ) ) ;
#9821=EDGE_CURVE ( 'NONE', #27542, #17245, #25022, .T. ) ;
#9822=DIRECTION ( 'NONE',  ( 1.000000000000000000, -1.224606353819999829E-16, 0.000000000000000000 ) ) ;
#9833=VERTEX_POINT ( 'NONE', #8657 ) ;
#9834=DIRECTION ( 'NONE',  ( 0.3633921898465273803, -0.9316362575375355393, 0.000000000000000000 ) ) ;
#9837=ORIENTED_EDGE ( 'NONE', *, *, #1167, .F. ) ;
#9839=CARTESIAN_POINT ( 'NONE',  ( 24.49999999470000134, -3.000285566199999922E-15, 39.99999999930000172 ) ) ;
#9860=ADVANCED_FACE ( 'NONE', ( #9441 ), #24087, .F. ) ;
#9861=DIRECTION ( 'NONE',  ( 0.9316362575375356503, 0.3633921898465274913, 0.000000000000000000 ) ) ;
#9863=CARTESIAN_POINT ( 'NONE',  ( 22.63992238019999803, -14.34133587289999845, 225.0000000000000000 ) ) ;
#9882=FACE_OUTER_BOUND ( 'NONE', #21612, .T. ) ;
#9887=CARTESIAN_POINT ( 'NONE',  ( 15.49562240950000103, -7.676231176589999983, 5.000000000000000000 ) ) ;
#9893=FACE_OUTER_BOUND ( 'NONE', #7918, .T. ) ;
#9901=EDGE_CURVE ( 'NONE', #7727, #16212, #21524, .T. ) ;
#9913=EDGE_LOOP ( 'NONE', ( #12762, #485, #12185, #16601, #14704, #16447 ) ) ;
#9915=CARTESIAN_POINT ( 'NONE',  ( -7.453090060300250563, -2.907137518772508589, 202.0000000000000000 ) ) ;
#9925=CARTESIAN_POINT ( 'NONE',  ( -22.92405521513462929, -13.88330634431700972, 5.957452580073338666 ) ) ;
#9930=CIRCLE ( 'NONE', #21994, 28.50000000000000000 ) ;
#9934=CARTESIAN_POINT ( 'NONE',  ( 6.336630981016743824, -26.76091511895456421, 21.17299964012854119 ) ) ;
#9936=VECTOR ( 'NONE', #25271, 1000.000000000000000 ) ;
#9946=ORIENTED_EDGE ( 'NONE', *, *, #9283, .F. ) ;
#9951=AXIS2_PLACEMENT_3D ( 'NONE', #16339, #28451, #30668 ) ;
#9954=FACE_OUTER_BOUND ( 'NONE', #13613, .T. ) ;
#9964=CARTESIAN_POINT ( 'NONE',  ( 0.000000000000000000, 0.000000000000000000, 41.66046017469999896 ) ) ;
#9966=ORIENTED_EDGE ( 'NONE', *, *, #1620, .F. ) ;
#9970=DIRECTION ( 'NONE',  ( -0.7071067811865475727, 0.7071067811865475727, 0.000000000000000000 ) ) ;
#9975=DIRECTION ( 'NONE',  ( 0.8090169943751909232, 0.5877852522921378498, 0.000000000000000000 ) ) ;
#9976=CARTESIAN_POINT ( 'NONE',  ( 27.92857142909999979, -3.420150602509999660E-15, 37.93968498519999599 ) ) ;
#9980=ORIENTED_EDGE ( 'NONE', *, *, #186, .F. ) ;
#9983=DIRECTION ( 'NONE',  ( 0.000000000000000000, 0.000000000000000000, 1.000000000000000000 ) ) ;
#9992=ORIENTED_EDGE ( 'NONE', *, *, #30762, .T. ) ;
#9998=CARTESIAN_POINT ( 'NONE',  ( 0.9598841921113454578, -27.48329941562163370, 224.4438356452711503 ) ) ;
#10002=DIRECTION ( 'NONE',  ( 1.000000000000000000, 0.000000000000000000, 0.000000000000000000 ) ) ;
#10007=CARTESIAN_POINT ( 'NONE',  ( 23.73992238018677625, -12.43607998452291419, 224.9035646525462937 ) ) ;
#10011=DIRECTION ( 'NONE',  ( 1.000000000000000000, 0.000000000000000000, 0.000000000000000000 ) ) ;
#10019=VECTOR ( 'NONE', #7299, 1000.000000000000000 ) ;
#10021=CARTESIAN_POINT ( 'NONE',  ( -24.14619884835838093, -13.16136950043478748, 5.880491002298545489 ) ) ;
#10022=DIRECTION ( 'NONE',  ( 0.000000000000000000, 0.000000000000000000, -1.000000000000000000 ) ) ;
#10024=CARTESIAN_POINT ( 'NONE',  ( -11.08346179031915568, -28.41490585489482967, 86.39444872449999480 ) ) ;
#10026=VECTOR ( 'NONE', #21492, 1000.000000000000000 ) ;
#10029=ORIENTED_EDGE ( 'NONE', *, *, #9375, .T. ) ;
#10034=EDGE_CURVE ( 'NONE', #18767, #22309, #15995, .T. ) ;
#10035=EDGE_LOOP ( 'NONE', ( #24630, #290, #20740, #6204 ) ) ;
#10041=CARTESIAN_POINT ( 'NONE',  ( 0.000000000000000000, 0.000000000000000000, 140.0000000000000000 ) ) ;
#10044=VERTEX_POINT ( 'NONE', #11731 ) ;
#10047=EDGE_CURVE ( 'NONE', #11948, #16822, #31075, .T. ) ;
#10051=CARTESIAN_POINT ( 'NONE',  ( 0.000000000000000000, 0.000000000000000000, 90.00000000000000000 ) ) ;
#10071=VERTEX_POINT ( 'NONE', #21335 ) ;
#10081=FACE_OUTER_BOUND ( 'NONE', #4457, .T. ) ;
#10082=DIRECTION ( 'NONE',  ( -0.9316362575375349842, 0.3633921898465292122, -0.000000000000000000 ) ) ;
#10084=CARTESIAN_POINT ( 'NONE',  ( -27.54391552379999908, 3.373045395960000230E-15, 42.95625301639999805 ) ) ;
#10100=ORIENTED_EDGE ( 'NONE', *, *, #23764, .F. ) ;
#10110=ORIENTED_EDGE ( 'NONE', *, *, #26962, .F. ) ;
#10115=ORIENTED_EDGE ( 'NONE', *, *, #4712, .T. ) ;
#10124=CARTESIAN_POINT ( 'NONE',  ( -26.62724484483129572, -3.508068424019920695, 193.2171415880000325 ) ) ;
#10134=ORIENTED_EDGE ( 'NONE', *, *, #29615, .T. ) ;
#10144=VERTEX_POINT ( 'NONE', #27948 ) ;
#10146=AXIS2_PLACEMENT_3D ( 'NONE', #3168, #7884, #5840 ) ;
#10151=CARTESIAN_POINT ( 'NONE',  ( -9.738910687886855655, -24.96785170200598714, 186.7828584120000244 ) ) ;
#10154=DIRECTION ( 'NONE',  ( -0.8660254037843289066, -0.5000000000001899592, 0.000000000000000000 ) ) ;
#10170=CARTESIAN_POINT ( 'NONE',  ( 3.552713678799999608E-15, -3.552713678799999608E-15, 136.7828584120000244 ) ) ;
#10173=CARTESIAN_POINT ( 'NONE',  ( -20.77057278543777485, -16.95162108973866921, 93.21714158846111786 ) ) ;
#10176=ADVANCED_FACE ( 'NONE', ( #16295 ), #14102, .F. ) ;
#10186=ORIENTED_EDGE ( 'NONE', *, *, #24494, .T. ) ;
#10194=DIRECTION ( 'NONE',  ( 1.000000000000000000, 0.000000000000000000, 0.000000000000000000 ) ) ;
#10199=DIRECTION ( 'NONE',  ( 0.000000000000000000, 0.000000000000000000, -1.000000000000000000 ) ) ;
#10205=CARTESIAN_POINT ( 'NONE',  ( -24.34663841809999951, -12.78636765230000094, 5.000000000000000000 ) ) ;
#10208=CARTESIAN_POINT ( 'NONE',  ( -26.80000000069999899, 3.281945028329999726E-15, 143.2171415869999862 ) ) ;
#10211=DIRECTION ( 'NONE',  ( 0.000000000000000000, 0.000000000000000000, 1.000000000000000000 ) ) ;
#10212=CARTESIAN_POINT ( 'NONE',  ( 24.29812717141672707, -12.87956648207215515, 225.4905541419588815 ) ) ;
#10213=ORIENTED_EDGE ( 'NONE', *, *, #26629, .T. ) ;
#10221=AXIS2_PLACEMENT_3D ( 'NONE', #807, #15416, #1264 ) ;
#10232=LINE ( 'NONE', #19832, #31027 ) ;
#10234=EDGE_CURVE ( 'NONE', #1598, #10318, #717, .T. ) ;
#10236=LINE ( 'NONE', #10387, #7214 ) ;
#10237=LINE ( 'NONE', #17458, #17019 ) ;
#10243=CIRCLE ( 'NONE', #18265, 4.000000004070001225 ) ;
#10246=CIRCLE ( 'NONE', #8195, 3.200000000000000178 ) ;
#10254=EDGE_CURVE ( 'NONE', #4699, #6773, #6381, .T. ) ;
#10260=VERTEX_POINT ( 'NONE', #19125 ) ;
#10268=DIRECTION ( 'NONE',  ( 0.3633921898465276024, -0.9316362575375355393, -6.071532165918824830E-14 ) ) ;
#10272=AXIS2_PLACEMENT_3D ( 'NONE', #18785, #6832, #8718 ) ;
#10276=DIRECTION ( 'NONE',  ( 0.000000000000000000, 0.000000000000000000, -1.000000000000000000 ) ) ;
#10282=CARTESIAN_POINT ( 'NONE',  ( 23.32129337744305886, -14.57293380325871723, 225.5561643542927470 ) ) ;
#10284=TOROIDAL_SURFACE ( 'NONE', #27599, 24.50000000000000000, 3.200000000000000178 ) ;
#10289=EDGE_CURVE ( 'NONE', #1493, #11656, #9385, .T. ) ;
#10291=ORIENTED_EDGE ( 'NONE', *, *, #15967, .F. ) ;
#10303=DIRECTION ( 'NONE',  ( 1.000000000000000000, 0.000000000000000000, 0.000000000000000000 ) ) ;
#10316=B_SPLINE_CURVE_WITH_KNOTS ( 'NONE', 3,
 ( #23926, #9590, #4716, #7074 ),
 .UNSPECIFIED., .F., .F.,
 ( 4, 4 ),
 ( 0.000000000000000000, 1.000000000000000000 ),
 .UNSPECIFIED. ) ;
#10318=VERTEX_POINT ( 'NONE', #10151 ) ;
#10320=CARTESIAN_POINT ( 'NONE',  ( 23.68723484229111875, -12.53725850769392380, 224.5052107121046276 ) ) ;
#10325=CARTESIAN_POINT ( 'NONE',  ( -6.496986506900674918, -26.00150201275824102, 208.5476012337068425 ) ) ;
#10332=FACE_OUTER_BOUND ( 'NONE', #13220, .T. ) ;
#10333=CARTESIAN_POINT ( 'NONE',  ( -5.393907605749490131, -26.25263145716210644, 20.79431568259033369 ) ) ;
#10337=DIRECTION ( 'NONE',  ( 0.000000000000000000, 0.000000000000000000, 1.000000000000000000 ) ) ;
#10339=VERTEX_POINT ( 'NONE', #26979 ) ;
#10348=ADVANCED_FACE ( 'NONE', ( #17217 ), #25481, .F. ) ;
#10352=ORIENTED_EDGE ( 'NONE', *, *, #1838, .F. ) ;
#10363=CARTESIAN_POINT ( 'NONE',  ( -27.69999999930000101, 3.392159599999999562E-15, 40.00000000000000000 ) ) ;
#10365=DIRECTION ( 'NONE',  ( 0.000000000000000000, 0.000000000000000000, -1.000000000000000000 ) ) ;
#10366=CARTESIAN_POINT ( 'NONE',  ( -19.36389667587700458, -18.53702679572192835, 43.21714158842222986 ) ) ;
#10369=ORIENTED_EDGE ( 'NONE', *, *, #13450, .F. ) ;
#10380=ORIENTED_EDGE ( 'NONE', *, *, #29638, .F. ) ;
#10387=CARTESIAN_POINT ( 'NONE',  ( -18.95046173579999760, -18.95046173579999760, 115.0000000000000000 ) ) ;
#10390=ADVANCED_FACE ( 'NONE', ( #10607 ), #10458, .T. ) ;
#10398=DIRECTION ( 'NONE',  ( 0.3633921898465276024, -0.9316362575375355393, 0.000000000000000000 ) ) ;
#10400=DIRECTION ( 'NONE',  ( 0.000000000000000000, 0.000000000000000000, 1.000000000000000000 ) ) ;
#10404=AXIS2_PLACEMENT_3D ( 'NONE', #11270, #20877, #30473 ) ;
#10405=ADVANCED_FACE ( 'NONE', ( #27747 ), #10760, .T. ) ;
#10408=EDGE_LOOP ( 'NONE', ( #10817, #4594, #10801, #11312 ) ) ;
#10409=DIRECTION ( 'NONE',  ( 1.000000000000000000, 0.000000000000000000, 0.000000000000000000 ) ) ;
#10417=VERTEX_POINT ( 'NONE', #18464 ) ;
#10418=DIRECTION ( 'NONE',  ( 0.000000000000000000, 0.000000000000000000, 1.000000000000000000 ) ) ;
#10426=CARTESIAN_POINT ( 'NONE',  ( 4.684462318791906554, -27.09927246286415325, 209.5983106348512877 ) ) ;
#10431=CARTESIAN_POINT ( 'NONE',  ( -25.43121960300666373, -8.635379644106540908, 193.2171415880000040 ) ) ;
#10434=CARTESIAN_POINT ( 'NONE',  ( 23.81569860410000317, -13.75000000000000000, 226.0999999999999943 ) ) ;
#10436=CARTESIAN_POINT ( 'NONE',  ( -23.26185891368683301, -14.66761890392226242, 224.7132485884542064 ) ) ;
#10440=CARTESIAN_POINT ( 'NONE',  ( 23.24663841807413434, -14.69162354064478215, 224.9035402886169095 ) ) ;
#10447=EDGE_LOOP ( 'NONE', ( #7176, #14850, #9432, #14639 ) ) ;
#10449=AXIS2_PLACEMENT_3D ( 'NONE', #675, #15286, #7732 ) ;
#10458=PLANE ( 'NONE',  #381 ) ;
#10474=CARTESIAN_POINT ( 'NONE',  ( -22.63992238019999803, -14.34133587289999845, 5.000000000000000000 ) ) ;
#10477=CARTESIAN_POINT ( 'NONE',  ( -23.24667624907491259, -14.69156368041574723, 4.854326830129346071 ) ) ;
#10482=ORIENTED_EDGE ( 'NONE', *, *, #23096, .F. ) ;
#10484=DIRECTION ( 'NONE',  ( 0.000000000000000000, 0.000000000000000000, -1.000000000000000000 ) ) ;
#10485=CARTESIAN_POINT ( 'NONE',  ( -26.84464184930000030, 3.287411897469999975E-15, 87.43750406049998958 ) ) ;
#10488=DIRECTION ( 'NONE',  ( -1.224606353819999829E-16, -1.000000000000000000, 0.000000000000000000 ) ) ;
#10489=B_SPLINE_CURVE_WITH_KNOTS ( 'NONE', 3,
 ( #26301, #14191, #4437, #11362, #9460, #20960, #7105, #30566, #16690, #28190 ),
 .UNSPECIFIED., .F., .F.,
 ( 4, 2, 2, 2, 4 ),
 ( 0.000000000000000000, 0.2500000000000000000, 0.5000000000000000000, 0.7500000000000000000, 1.000000000000000000 ),
 .UNSPECIFIED. ) ;
#10497=ORIENTED_EDGE ( 'NONE', *, *, #1586, .F. ) ;
#10506=ORIENTED_EDGE ( 'NONE', *, *, #19533, .F. ) ;
#10511=CARTESIAN_POINT ( 'NONE',  ( -28.50000000000000000, 3.490128108389999698E-15, 190.0000000000000000 ) ) ;
#10513=CARTESIAN_POINT ( 'NONE',  ( 23.25788685383077592, -13.43083806724684948, 86.78285841136666079 ) ) ;
#10516=AXIS2_PLACEMENT_3D ( 'NONE', #18427, #6470, #16072 ) ;
#10518=CARTESIAN_POINT ( 'NONE',  ( 4.679341198149911563, -26.38945575071662830, 209.5097050137637211 ) ) ;
#10520=CARTESIAN_POINT ( 'NONE',  ( -26.62724484483073439, -3.508068424025491794, 43.21714158835001030 ) ) ;
#10523=CARTESIAN_POINT ( 'NONE',  ( 7.297190580108170899, -25.78810378223603195, 22.11652997304829427 ) ) ;
#10541=CARTESIAN_POINT ( 'NONE',  ( 2.131628207279999844E-14, -5.329070518200000398E-15, 86.78285841159998881 ) ) ;
#10557=LINE ( 'NONE', #20151, #21338 ) ;
#10560=DIRECTION ( 'NONE',  ( 0.3633921898465289901, 0.9316362575375348731, -8.673617379884029161E-15 ) ) ;
#10565=CARTESIAN_POINT ( 'NONE',  ( -4.684462318791891455, -27.09927246286417102, 20.40168936514870168 ) ) ;
#10568=VERTEX_POINT ( 'NONE', #16715 ) ;
#10579=EDGE_CURVE ( 'NONE', #18294, #25078, #29998, .T. ) ;
#10583=DIRECTION ( 'NONE',  ( 0.000000000000000000, 0.000000000000000000, 1.000000000000000000 ) ) ;
#10584=CARTESIAN_POINT ( 'NONE',  ( -1.099928585426612759, -27.47799405182390231, 5.145501061710134216 ) ) ;
#10600=ORIENTED_EDGE ( 'NONE', *, *, #8259, .F. ) ;
#10604=DIRECTION ( 'NONE',  ( -0.9316362575375349842, 0.3633921898465292122, -0.000000000000000000 ) ) ;
#10607=FACE_OUTER_BOUND ( 'NONE', #4300, .T. ) ;
#10611=CARTESIAN_POINT ( 'NONE',  ( -27.92857142909999979, 3.420150602519999655E-15, 192.0603150150000147 ) ) ;
#10626=DIRECTION ( 'NONE',  ( 0.9316362575375356503, 0.3633921898465274913, 0.000000000000000000 ) ) ;
#10627=ORIENTED_EDGE ( 'NONE', *, *, #11105, .T. ) ;
#10631=CARTESIAN_POINT ( 'NONE',  ( -25.51870711004141157, -8.199261060474288598, 93.21714158836661568 ) ) ;
#10632=DIRECTION ( 'NONE',  ( 0.7071067811865475727, -0.7071067811865475727, 0.000000000000000000 ) ) ;
#10638=CARTESIAN_POINT ( 'NONE',  ( 0.000000000000000000, 0.000000000000000000, 115.0000000000000000 ) ) ;
#10643=EDGE_LOOP ( 'NONE', ( #9191, #27901, #12767, #3759, #23413, #21149, #10369, #8941, #6341, #5138, #25038, #13599, #7878, #29289, #13434, #11959, #30221, #8036, #27168, #28675, #7358, #24948, #28667, #13028, #23509, #8857, #19786, #22933, #6941, #21923, #24880, #23462, #7116, #31034, #3565, #17450, #16137, #30969, #28567, #2768, #25441, #29516, #1857, #1004 ) ) ;
#10657=CARTESIAN_POINT ( 'NONE',  ( 23.60764285305539545, -12.68553248495022423, 4.262772992568688579 ) ) ;
#10660=CARTESIAN_POINT ( 'NONE',  ( 26.80000000069999899, -3.281945028320000125E-15, 86.78285841090000474 ) ) ;
#10668=CARTESIAN_POINT ( 'NONE',  ( 7.107063564515522458, -25.84129680694968911, 21.94110913170587551 ) ) ;
#10671=ADVANCED_FACE ( 'NONE', ( #30401 ), #22490, .F. ) ;
#10672=ORIENTED_EDGE ( 'NONE', *, *, #26962, .T. ) ;
#10684=CARTESIAN_POINT ( 'NONE',  ( -1.087565149828547018, -27.47889317205697779, 4.782085928244144135 ) ) ;
#10693=B_SPLINE_CURVE_WITH_KNOTS ( 'NONE', 3,
 ( #23429, #9084, #1856, #3903, #21057, #6264, #18679, #6722, #13497, #26091 ),
 .UNSPECIFIED., .F., .F.,
 ( 4, 2, 2, 2, 4 ),
 ( 0.000000000000000000, 0.2500000000000000000, 0.5000000000000000000, 0.7500000000000000000, 1.000000000000000000 ),
 .UNSPECIFIED. ) ;
#10698=EDGE_CURVE ( 'NONE', #23553, #11358, #3891, .T. ) ;
#10700=CARTESIAN_POINT ( 'NONE',  ( 0.000000000000000000, 0.000000000000000000, 140.0000000000000000 ) ) ;
#10713=VERTEX_POINT ( 'NONE', #28334 ) ;
#10722=CARTESIAN_POINT ( 'NONE',  ( 9.993285220779439371, -25.61999708228226069, 202.0000000000000000 ) ) ;
#10726=ADVANCED_FACE ( 'NONE', ( #18425 ), #25680, .T. ) ;
#10730=CARTESIAN_POINT ( 'NONE',  ( -25.94284618478184967, -6.948772836044501133, 193.2171415879999756 ) ) ;
#10736=CARTESIAN_POINT ( 'NONE',  ( 18.95046173579999760, -18.95046173579999760, 86.78285841159998881 ) ) ;
#10739=ORIENTED_EDGE ( 'NONE', *, *, #11600, .F. ) ;
#10745=CARTESIAN_POINT ( 'NONE',  ( 27.06563796000000366, -3.314475221599999482E-15, 138.0597313979999967 ) ) ;
#10753=CARTESIAN_POINT ( 'NONE',  ( -26.80000000000000071, 9.769962616700000205E-15, 186.7828584120000244 ) ) ;
#10755=ORIENTED_EDGE ( 'NONE', *, *, #22457, .T. ) ;
#10760=CYLINDRICAL_SURFACE ( 'NONE', #21981, 27.50000000000000000 ) ;
#10763=COLOUR_RGB ( '', 0.72549020, 0.75294118, 0.79215686) ;
#10768=CARTESIAN_POINT ( 'NONE',  ( 0.9891023320736628266, -26.78175549074274642, 5.486606153706005351 ) ) ;
#10772=CARTESIAN_POINT ( 'NONE',  ( 9.738910687886868089, -24.96785170200598358, 115.0000000000000000 ) ) ;
#10781=FACE_OUTER_BOUND ( 'NONE', #21928, .T. ) ;
#10784=CARTESIAN_POINT ( 'NONE',  ( 27.50000000000000000, 1.776356839399999804E-15, 86.39444872449999480 ) ) ;
#10785=VERTEX_POINT ( 'NONE', #24699 ) ;
#10801=ORIENTED_EDGE ( 'NONE', *, *, #17586, .T. ) ;
#10814=AXIS2_PLACEMENT_3D ( 'NONE', #25884, #6827, #23208 ) ;
#10817=ORIENTED_EDGE ( 'NONE', *, *, #16638, .T. ) ;
#10824=DIRECTION ( 'NONE',  ( 0.3633921898465291567, 0.9316362575375349842, -1.850371707708594444E-14 ) ) ;
#10825=B_SPLINE_CURVE_WITH_KNOTS ( 'NONE', 5,
 ( #15821, #29667, #8564, #13133, #885, #17847 ),
 .UNSPECIFIED., .F., .F.,
 ( 6, 6 ),
 ( -2.300779637600000260, 0.000000000000000000 ),
 .UNSPECIFIED. ) ;
#10831=PRODUCT ( 'Cradle Body', 'Cradle Body', '', ( #28137 ) ) ;
#10834=CARTESIAN_POINT ( 'NONE',  ( -24.83284505762695815, -10.07844553579556823, 43.21714158839643005 ) ) ;
#10835=CARTESIAN_POINT ( 'NONE',  ( 24.34663841808528417, -12.78636765232546146, 225.0964597117140045 ) ) ;
#10842=ORIENTED_EDGE ( 'NONE', *, *, #17728, .T. ) ;
#10847=CARTESIAN_POINT ( 'NONE',  ( 0.000000000000000000, 0.000000000000000000, 90.00000000000000000 ) ) ;
#10851=EDGE_CURVE ( 'NONE', #24389, #16212, #20164, .T. ) ;
#10857=EDGE_CURVE ( 'NONE', #13261, #2824, #10232, .T. ) ;
#10860=EDGE_CURVE ( 'NONE', #17478, #9711, #14454, .T. ) ;
#10864=DIRECTION ( 'NONE',  ( 0.000000000000000000, 0.000000000000000000, 1.000000000000000000 ) ) ;
#10869=FACE_OUTER_BOUND ( 'NONE', #22176, .T. ) ;
#10878=CARTESIAN_POINT ( 'NONE',  ( -9.993285220779425160, -25.61999708228226069, 27.99999999999999645 ) ) ;
#10880=EDGE_LOOP ( 'NONE', ( #13124, #6459, #2900, #4944, #27760, #9966 ) ) ;
#10884=DIRECTION ( 'NONE',  ( -1.224606353819999829E-16, -1.000000000000000000, 0.000000000000000000 ) ) ;
#10885=ORIENTED_EDGE ( 'NONE', *, *, #9283, .T. ) ;
#10888=CARTESIAN_POINT ( 'NONE',  ( 6.756062549273604390, -26.65810324902503581, 208.5456572472911034 ) ) ;
#10894=CARTESIAN_POINT ( 'NONE',  ( -9.993285220779425160, -25.61999708228226069, 202.0000000000000000 ) ) ;
#10895=CARTESIAN_POINT ( 'NONE',  ( 0.000000000000000000, 0.000000000000000000, 20.00000000000000355 ) ) ;
#10916=DIRECTION ( 'NONE',  ( 0.000000000000000000, 0.000000000000000000, -1.000000000000000000 ) ) ;
#10918=CARTESIAN_POINT ( 'NONE',  ( 9.738910687886932038, -24.96785170200595161, 43.21714158840000408 ) ) ;
#10921=ADVANCED_FACE ( 'NONE', ( #6278 ), #28530, .F. ) ;
#10923=VECTOR ( 'NONE', #22109, 1000.000000000000000 ) ;
#10930=CARTESIAN_POINT ( 'NONE',  ( 1.099927927705516062, -26.77741881808359992, 5.145878552788805571 ) ) ;
#10931=CARTESIAN_POINT ( 'NONE',  ( -26.84464183080000055, 3.287411895199999866E-15, 92.56249624490000372 ) ) ;
#10954=EDGE_LOOP ( 'NONE', ( #20826, #21277, #13107, #5367 ) ) ;
#10957=AXIS2_PLACEMENT_3D ( 'NONE', #21245, #1318, #14014 ) ;
#10963=CARTESIAN_POINT ( 'NONE',  ( -23.64633388399750658, -12.61377020593197784, 225.6389823649609525 ) ) ;
#10986=CARTESIAN_POINT ( 'NONE',  ( -27.92857142909999979, 3.420150602519999655E-15, 192.0603150150000147 ) ) ;
#10987=CIRCLE ( 'NONE', #17514, 27.50000000000000000 ) ;
#10991=CIRCLE ( 'NONE', #20017, 4.000000000000001776 ) ;
#11011=DIRECTION ( 'NONE',  ( 0.000000000000000000, 0.000000000000000000, -1.000000000000000000 ) ) ;
#11018=B_SPLINE_CURVE_WITH_KNOTS ( 'NONE', 3,
 ( #26187, #4622, #16887, #12472, #14389, #23988, #9501, #7449, #7141, #31062, #14228, #26646, #75, #24137 ),
 .UNSPECIFIED., .F., .F.,
 ( 4, 2, 2, 2, 2, 2, 4 ),
 ( 0.000000000000000000, 0.2500000000000006106, 0.3750000000000016098, 0.4375000000000014433, 0.5000000000000013323, 0.7500000000000006661, 1.000000000000000000 ),
 .UNSPECIFIED. ) ;
#11019=CARTESIAN_POINT ( 'NONE',  ( 23.20948082139999968, -13.40000000000000036, 226.0999999999999943 ) ) ;
#11022=ORIENTED_EDGE ( 'NONE', *, *, #7708, .T. ) ;
#11023=VERTEX_POINT ( 'NONE', #16340 ) ;
#11028=CARTESIAN_POINT ( 'NONE',  ( -22.96035733413718916, -13.82212301906527863, 224.0048062721249664 ) ) ;
#11033=CARTESIAN_POINT ( 'NONE',  ( -9.797681423453962424, -25.69548940455785413, 26.16126510391729454 ) ) ;
#11035=ORIENTED_EDGE ( 'NONE', *, *, #27794, .F. ) ;
#11037=AXIS2_PLACEMENT_3D ( 'NONE', #3327, #13229, #15298 ) ;
#11052=DIRECTION ( 'NONE',  ( -1.224606353819999829E-16, -1.000000000000000000, 0.000000000000000000 ) ) ;
#11056=DIRECTION ( 'NONE',  ( 0.9316362575375356503, 0.3633921898465274913, 0.000000000000000000 ) ) ;
#11060=DIRECTION ( 'NONE',  ( 0.000000000000000000, 0.000000000000000000, 1.000000000000000000 ) ) ;
#11063=DIRECTION ( 'NONE',  ( -1.000000000000000000, 5.665498452320000818E-16, 0.000000000000000000 ) ) ;
#11064=ORIENTED_EDGE ( 'NONE', *, *, #9065, .T. ) ;
#11073=CARTESIAN_POINT ( 'NONE',  ( -11.08346179031913437, -28.41490585489481191, 143.6055512749999821 ) ) ;
#11077=AXIS2_PLACEMENT_3D ( 'NONE', #19834, #26912, #12580 ) ;
#11091=CARTESIAN_POINT ( 'NONE',  ( -9.738910687886855655, -24.96785170200598714, 136.7828584120000244 ) ) ;
#11105=EDGE_CURVE ( 'NONE', #13694, #7124, #12629, .T. ) ;
#11117=ORIENTED_EDGE ( 'NONE', *, *, #19157, .T. ) ;
#11132=CIRCLE ( 'NONE', #22179, 26.80000000000000071 ) ;
#11134=DIRECTION ( 'NONE',  ( 1.000000000000000000, 0.000000000000000000, 0.000000000000000000 ) ) ;
#11143=ORIENTED_EDGE ( 'NONE', *, *, #255, .F. ) ;
#11145=ORIENTED_EDGE ( 'NONE', *, *, #17385, .F. ) ;
#11149=EDGE_CURVE ( 'NONE', #6137, #27823, #13962, .T. ) ;
#11151=VERTEX_POINT ( 'NONE', #27473 ) ;
#11158=DIRECTION ( 'NONE',  ( 0.9316362575375349842, -0.3633921898465292122, 0.000000000000000000 ) ) ;
#11174=ADVANCED_FACE ( 'NONE', ( #5312 ), #17946, .T. ) ;
#11175=DIRECTION ( 'NONE',  ( 1.000000000000000000, -1.224606353819998843E-16, 0.000000000000000000 ) ) ;
#11195=CARTESIAN_POINT ( 'NONE',  ( 23.28322851840398755, -13.27226524188811752, 6.100000000000007638 ) ) ;
#11208=CARTESIAN_POINT ( 'NONE',  ( 23.95771897998607969, -13.50170546740720035, 223.9280906791277062 ) ) ;
#11211=ORIENTED_EDGE ( 'NONE', *, *, #12589, .F. ) ;
#11223=ORIENTED_EDGE ( 'NONE', *, *, #9204, .T. ) ;
#11228=CARTESIAN_POINT ( 'NONE',  ( 23.70578532274842942, -13.93854223037613238, 3.912293196490389757 ) ) ;
#11233=CARTESIAN_POINT ( 'NONE',  ( -0.6805610060751490220, -26.79155681327128491, 224.1233511992632828 ) ) ;
#11240=DIRECTION ( 'NONE',  ( 0.000000000000000000, 0.000000000000000000, 1.000000000000000000 ) ) ;
#11246=CYLINDRICAL_SURFACE ( 'NONE', #10272, 26.80000000000002203 ) ;
#11249=CARTESIAN_POINT ( 'NONE',  ( 22.65536398230910820, -14.31703479027868831, 4.711904017054809657 ) ) ;
#11259=TOROIDAL_SURFACE ( 'NONE', #28826, 30.50000000000000000, 3.000000000000000000 ) ;
#11269=ORIENTED_EDGE ( 'NONE', *, *, #1416, .T. ) ;
#11270=CARTESIAN_POINT ( 'NONE',  ( 7.453090060300315400, -2.907137518772522355, 202.0000000000000000 ) ) ;
#11274=AXIS2_PLACEMENT_3D ( 'NONE', #29310, #7757, #17359 ) ;
#11278=EDGE_CURVE ( 'NONE', #18284, #25472, #22533, .T. ) ;
#11288=DIRECTION ( 'NONE',  ( 0.000000000000000000, 0.000000000000000000, -1.000000000000000000 ) ) ;
#11300=AXIS2_PLACEMENT_3D ( 'NONE', #1780, #23651, #26157 ) ;
#11301=CIRCLE ( 'NONE', #28882, 3.200000004570001888 ) ;
#11303=ORIENTED_EDGE ( 'NONE', *, *, #23615, .F. ) ;
#11312=ORIENTED_EDGE ( 'NONE', *, *, #24288, .F. ) ;
#11325=CIRCLE ( 'NONE', #5782, 28.50000000000000000 ) ;
#11328=CARTESIAN_POINT ( 'NONE',  ( -0.9003584927496220969, -26.78512143699428094, 5.633487050009015285 ) ) ;
#11334=DIRECTION ( 'NONE',  ( -1.000000000000000000, 0.000000000000000000, 0.000000000000000000 ) ) ;
#11337=CARTESIAN_POINT ( 'NONE',  ( 27.50000000000000000, -3.367667472999999580E-15, 65.00000000000000000 ) ) ;
#11338=ORIENTED_EDGE ( 'NONE', *, *, #4593, .T. ) ;
#11341=CARTESIAN_POINT ( 'NONE',  ( 0.6479068412426576273, -26.79235971056621324, 4.090187300791521707 ) ) ;
#11352=CARTESIAN_POINT ( 'NONE',  ( -24.49999999589999788, 3.000285566369999841E-15, 40.00000000000000000 ) ) ;
#11356=CARTESIAN_POINT ( 'NONE',  ( 23.73988890810274910, -12.43614388128991877, 5.145878552484940194 ) ) ;
#11358=VERTEX_POINT ( 'NONE', #6701 ) ;
#11361=CARTESIAN_POINT ( 'NONE',  ( -8.986416953306164856, -25.99194954040540040, 206.0369953409331174 ) ) ;
#11362=CARTESIAN_POINT ( 'NONE',  ( 23.67414648230973739, -12.56096907828687392, 225.5575347054845281 ) ) ;
#11385=FACE_OUTER_BOUND ( 'NONE', #7287, .T. ) ;
#11395=CARTESIAN_POINT ( 'NONE',  ( -23.73992238018677980, -12.43607998452291774, 5.097059004422684225 ) ) ;
#11398=CARTESIAN_POINT ( 'NONE',  ( -23.13685276725654916, -13.52579547987099140, 226.1000000000000227 ) ) ;
#11400=CARTESIAN_POINT ( 'NONE',  ( 26.62724484483131349, -3.508068424019962883, 136.7828584120000528 ) ) ;
#11406=CARTESIAN_POINT ( 'NONE',  ( 6.984668861240829862, -26.60192251835760402, 21.60853132520131936 ) ) ;
#11412=DIRECTION ( 'NONE',  ( 0.3633921898465272138, -0.9316362575375356503, -1.850371707708593498E-14 ) ) ;
#11437=AXIS2_PLACEMENT_3D ( 'NONE', #3918, #20751, #29725 ) ;
#11440=EDGE_LOOP ( 'NONE', ( #17400, #10672, #7933, #23322, #11733, #2409 ) ) ;
#11453=CARTESIAN_POINT ( 'NONE',  ( -23.81569860410000317, -13.75000000000000000, 6.099999999630000502 ) ) ;
#11459=VECTOR ( 'NONE', #28062, 1000.000000000000114 ) ;
#11482=CARTESIAN_POINT ( 'NONE',  ( -0.6479069172523121978, -26.79235980091754143, 5.909812225168041167 ) ) ;
#11488=CARTESIAN_POINT ( 'NONE',  ( -10.35667741062608371, -26.55163333981974816, 140.0000000000000000 ) ) ;
#11489=TOROIDAL_SURFACE ( 'NONE', #31078, 24.50000000000000000, 4.000000000000000000 ) ;
#11492=VERTEX_POINT ( 'NONE', #18134 ) ;
#11494=CARTESIAN_POINT ( 'NONE',  ( 1.018915990056934673, -26.78112376029977426, 4.579415541090104291 ) ) ;
#11504=DIRECTION ( 'NONE',  ( 0.000000000000000000, 0.000000000000000000, 1.000000000000000000 ) ) ;
#11506=CARTESIAN_POINT ( 'NONE',  ( 0.000000000000000000, 0.000000000000000000, 190.0000000000000000 ) ) ;
#11510=CARTESIAN_POINT ( 'NONE',  ( -24.08673398027933388, -11.88135228261326226, -0.000000000000000000 ) ) ;
#11511=EDGE_CURVE ( 'NONE', #2408, #17004, #16476, .T. ) ;
#11523=DIRECTION ( 'NONE',  ( 1.000000000000000000, 0.000000000000000000, 0.000000000000000000 ) ) ;
#11531=DIRECTION ( 'NONE',  ( -0.9316362575375349842, 0.3633921898465292122, -0.000000000000000000 ) ) ;
#11535=CARTESIAN_POINT ( 'NONE',  ( 23.24667624907481667, -14.69156368041588934, 5.145673169868544505 ) ) ;
#11541=ORIENTED_EDGE ( 'NONE', *, *, #26945, .T. ) ;
#11544=CARTESIAN_POINT ( 'NONE',  ( 8.903108651239925564, -22.82508830966962421, 140.0000000000000000 ) ) ;
#11557=CARTESIAN_POINT ( 'NONE',  ( 26.62825631580874131, -3.503650093567661106, -0.000000000000000000 ) ) ;
#11558=LINE ( 'NONE', #25727, #16523 ) ;
#11565=DIRECTION ( 'NONE',  ( 0.000000000000000000, 0.000000000000000000, 1.000000000000000000 ) ) ;
#11569=ORIENTED_EDGE ( 'NONE', *, *, #947, .F. ) ;
#11578=CARTESIAN_POINT ( 'NONE',  ( 27.54391550599999761, -3.373045393770000084E-15, 37.04374668510000390 ) ) ;
#11586=CARTESIAN_POINT ( 'NONE',  ( -27.06563796000000366, 3.314475221609999872E-15, 188.0597313979999967 ) ) ;
#11592=DIRECTION ( 'NONE',  ( 0.000000000000000000, 0.000000000000000000, 1.000000000000000000 ) ) ;
#11595=CARTESIAN_POINT ( 'NONE',  ( 0.1474953887282549891, -26.80000000000001492, 226.0999999999999943 ) ) ;
#11600=EDGE_CURVE ( 'NONE', #6881, #24307, #15704, .T. ) ;
#11609=CARTESIAN_POINT ( 'NONE',  ( -0.9950318224731415917, -27.48257863589062566, 224.5094458579580987 ) ) ;
#11613=ORIENTED_EDGE ( 'NONE', *, *, #8085, .F. ) ;
#11633=EDGE_CURVE ( 'NONE', #4159, #15947, #30040, .T. ) ;
#11642=ADVANCED_FACE ( 'NONE', ( #17746 ), #29033, .F. ) ;
#11643=CARTESIAN_POINT ( 'NONE',  ( 27.92857142909999979, -3.420150602509999660E-15, 187.9396849849999853 ) ) ;
#11655=DIRECTION ( 'NONE',  ( -0.9316362575375356503, -0.3633921898465274913, 0.000000000000000000 ) ) ;
#11656=VERTEX_POINT ( 'NONE', #29723 ) ;
#11667=CIRCLE ( 'NONE', #3608, 27.50000000000000000 ) ;
#11677=DIRECTION ( 'NONE',  ( 1.000000000000000000, 0.000000000000000000, 0.000000000000000000 ) ) ;
#11691=ORIENTED_EDGE ( 'NONE', *, *, #11633, .F. ) ;
#11703=EDGE_CURVE ( 'NONE', #4659, #21418, #6933, .T. ) ;
#11714=LINE ( 'NONE', #1974, #20231 ) ;
#11716=CARTESIAN_POINT ( 'NONE',  ( 8.754113545170000556E-10, -26.80000000020000073, 230.0000000000000000 ) ) ;
#11717=VERTEX_POINT ( 'NONE', #23595 ) ;
#11724=DIRECTION ( 'NONE',  ( 1.000000000000000000, 0.000000000000000000, 0.000000000000000000 ) ) ;
#11726=ORIENTED_EDGE ( 'NONE', *, *, #21391, .F. ) ;
#11731=CARTESIAN_POINT ( 'NONE',  ( -10.35667741062608371, -26.55163333981974816, 90.00000000000000000 ) ) ;
#11733=ORIENTED_EDGE ( 'NONE', *, *, #5945, .T. ) ;
#11741=ORIENTED_EDGE ( 'NONE', *, *, #7883, .F. ) ;
#11743=CARTESIAN_POINT ( 'NONE',  ( 0.2892544100089353698, -26.79878419707955572, 226.0714905181768017 ) ) ;
#11748=AXIS2_PLACEMENT_3D ( 'NONE', #13421, #10916, #13587 ) ;
#11752=CARTESIAN_POINT ( 'NONE',  ( -11.08346179031915568, -28.41490585489482967, 36.39444872449999480 ) ) ;
#11756=EDGE_CURVE ( 'NONE', #20656, #4699, #28547, .T. ) ;
#11773=VERTEX_POINT ( 'NONE', #1870 ) ;
#11777=DIRECTION ( 'NONE',  ( -1.000000000000000000, 5.665498452320000818E-16, 0.000000000000000000 ) ) ;
#11784=CARTESIAN_POINT ( 'NONE',  ( -18.95046173579999760, -18.95046173579999760, 43.21714158840000408 ) ) ;
#11795=CARTESIAN_POINT ( 'NONE',  ( -23.73992238019999945, -12.43607998449999918, 5.000000000000000000 ) ) ;
#11798=ORIENTED_EDGE ( 'NONE', *, *, #20055, .F. ) ;
#11801=AXIS2_PLACEMENT_3D ( 'NONE', #16611, #25609, #4353 ) ;
#11805=CARTESIAN_POINT ( 'NONE',  ( -3.552713678799999608E-15, 0.000000000000000000, 193.2171415880000040 ) ) ;
#11811=ADVANCED_FACE ( 'NONE', ( #13829 ), #2031, .F. ) ;
#11815=FACE_OUTER_BOUND ( 'NONE', #27696, .T. ) ;
#11821=DIRECTION ( 'NONE',  ( 0.9316362575375356503, 0.3633921898465274913, 0.000000000000000000 ) ) ;
#11823=CARTESIAN_POINT ( 'NONE',  ( -8.903108651239966420, -22.82508830966961000, 40.00000000000000000 ) ) ;
#11835=CARTESIAN_POINT ( 'NONE',  ( -1.421085471519999843E-14, -1.065814103639999922E-14, 136.7828584120000244 ) ) ;
#11838=VERTEX_POINT ( 'NONE', #4690 ) ;
#11843=LINE ( 'NONE', #6811, #2744 ) ;
#11844=ORIENTED_EDGE ( 'NONE', *, *, #20932, .T. ) ;
#11846=VERTEX_POINT ( 'NONE', #8943 ) ;
#11849=CARTESIAN_POINT ( 'NONE',  ( 27.06563796540000411, -3.314475222259999564E-15, 38.05973140639999741 ) ) ;
#11850=PRODUCT_DEFINITION_FORMATION_WITH_SPECIFIED_SOURCE ( 'ANY', '', #10831, .NOT_KNOWN. ) ;
#11851=CARTESIAN_POINT ( 'NONE',  ( -8.903108651239966420, -22.82508830966961000, 90.00000000000000000 ) ) ;
#11853=ORIENTED_EDGE ( 'NONE', *, *, #3778, .T. ) ;
#11856=EDGE_CURVE ( 'NONE', #20367, #1634, #21052, .T. ) ;
#11860=CARTESIAN_POINT ( 'NONE',  ( -22.86552662831838489, -13.97920826416505946, 225.8816713824261910 ) ) ;
#11871=CARTESIAN_POINT ( 'NONE',  ( -9.738910687886987105, -24.96785170200594095, 93.21714158839999698 ) ) ;
#11875=CARTESIAN_POINT ( 'NONE',  ( 0.000000000000000000, 0.000000000000000000, 115.0000000000000000 ) ) ;
#11877=CYLINDRICAL_SURFACE ( 'NONE', #18839, 27.50000000000000000 ) ;
#11881=CARTESIAN_POINT ( 'NONE',  ( -3.552713678799999608E-15, 0.000000000000000000, 93.21714158839999698 ) ) ;
#11885=ORIENTED_EDGE ( 'NONE', *, *, #12141, .T. ) ;
#11889=CARTESIAN_POINT ( 'NONE',  ( 0.000000000000000000, 0.000000000000000000, 40.00000000000000000 ) ) ;
#11895=CARTESIAN_POINT ( 'NONE',  ( 10.06596365874881194, -25.80632433378973900, 40.00000000000000000 ) ) ;
#11898=DIRECTION ( 'NONE',  ( 0.000000000000000000, 0.000000000000000000, 1.000000000000000000 ) ) ;
#11901=CARTESIAN_POINT ( 'NONE',  ( 0.000000000000000000, 0.000000000000000000, 191.6604601750000256 ) ) ;
#11905=CARTESIAN_POINT ( 'NONE',  ( 10.14902473058288912, -26.01926976374856437, 137.9396849850000137 ) ) ;
#11907=AXIS2_PLACEMENT_3D ( 'NONE', #14879, #12044, #24621 ) ;
#11913=DIRECTION ( 'NONE',  ( 0.3633921898465291567, 0.9316362575375349842, 0.000000000000000000 ) ) ;
#11915=VERTEX_POINT ( 'NONE', #7658 ) ;
#11940=CARTESIAN_POINT ( 'NONE',  ( -1.421085471519999843E-14, -1.065814103639999922E-14, 136.7828584120000244 ) ) ;
#11946=CIRCLE ( 'NONE', #2418, 26.80000000000000071 ) ;
#11948=VERTEX_POINT ( 'NONE', #25124 ) ;
#11957=ORIENTED_EDGE ( 'NONE', *, *, #19991, .F. ) ;
#11959=ORIENTED_EDGE ( 'NONE', *, *, #6124, .T. ) ;
#11961=EDGE_LOOP ( 'NONE', ( #29787, #722, #16067, #10842 ) ) ;
#11969=CARTESIAN_POINT ( 'NONE',  ( 11.08346179031909884, -28.41490585489484744, 143.6055512749999821 ) ) ;
#11971=CARTESIAN_POINT ( 'NONE',  ( 2.873028037699999811E-09, -3.314704954960000014E-09, 230.0000000000000000 ) ) ;
#11985=EDGE_CURVE ( 'NONE', #14204, #30811, #22723, .T. ) ;
#12005=DIRECTION ( 'NONE',  ( 1.000000000000000000, 0.000000000000000000, 0.000000000000000000 ) ) ;
#12006=ORIENTED_EDGE ( 'NONE', *, *, #17325, .T. ) ;
#12012=CYLINDRICAL_SURFACE ( 'NONE', #14994, 27.50000000000000000 ) ;
#12021=CARTESIAN_POINT ( 'NONE',  ( 22.63992238021892334, -14.34133587286723710, 5.097059004917531944 ) ) ;
#12023=DIRECTION ( 'NONE',  ( 0.000000000000000000, -1.000000000000000000, 0.000000000000000000 ) ) ;
#12024=CARTESIAN_POINT ( 'NONE',  ( 0.000000000000000000, 0.000000000000000000, 40.00000000000000000 ) ) ;
#12027=CIRCLE ( 'NONE', #14554, 26.80000000000000071 ) ;
#12035=VERTEX_POINT ( 'NONE', #13316 ) ;
#12042=ORIENTED_EDGE ( 'NONE', *, *, #7790, .T. ) ;
#12044=DIRECTION ( 'NONE',  ( 0.000000000000000000, 0.000000000000000000, 1.000000000000000000 ) ) ;
#12045=COLOUR_RGB ( '', 0.72549020, 0.75294118, 0.79215686) ;
#12048=CARTESIAN_POINT ( 'NONE',  ( -23.81569860410000317, -13.75000000000000000, 3.900000000369999942 ) ) ;
#12057=EDGE_CURVE ( 'NONE', #16896, #13818, #28419, .T. ) ;
#12062=CARTESIAN_POINT ( 'NONE',  ( -28.50000000000000000, 3.490128108389999698E-15, 90.00000000000000000 ) ) ;
#12067=CARTESIAN_POINT ( 'NONE',  ( -18.95046173579999760, -18.95046173579999760, 186.7828584120000244 ) ) ;
#12069=VERTEX_POINT ( 'NONE', #4037 ) ;
#12070=CARTESIAN_POINT ( 'NONE',  ( 7.105427357599999217E-15, 3.552713678799999608E-15, 193.6055512750000105 ) ) ;
#12071=ORIENTED_EDGE ( 'NONE', *, *, #27532, .F. ) ;
#12076=AXIS2_PLACEMENT_3D ( 'NONE', #8946, #11158, #15881 ) ;
#12078=VERTEX_POINT ( 'NONE', #6394 ) ;
#12079=CARTESIAN_POINT ( 'NONE',  ( 0.000000000000000000, 0.000000000000000000, 115.0000000000000000 ) ) ;
#12092=DIRECTION ( 'NONE',  ( 1.000000000000000000, -1.224606353819998843E-16, 0.000000000000000000 ) ) ;
#12094=DIRECTION ( 'NONE',  ( 1.000000000000000000, 0.000000000000000000, 0.000000000000000000 ) ) ;
#12097=CARTESIAN_POINT ( 'NONE',  ( 0.9242233386863408784, -26.78436825977087565, 224.4020708179980659 ) ) ;
#12105=CARTESIAN_POINT ( 'NONE',  ( 24.08956650209805872, -13.26503430050375876, 4.040453396065998959 ) ) ;
#12107=EDGE_LOOP ( 'NONE', ( #10029, #20668, #449, #10506, #2984 ) ) ;
#12113=ORIENTED_EDGE ( 'NONE', *, *, #8628, .T. ) ;
#12114=DIRECTION ( 'NONE',  ( -0.9316362575375349842, 0.3633921898465292122, -0.000000000000000000 ) ) ;
#12119=EDGE_CURVE ( 'NONE', #8812, #5207, #4664, .T. ) ;
#12130=CARTESIAN_POINT ( 'NONE',  ( -23.76736455417796279, -13.83371703020049637, 226.1000000000011312 ) ) ;
#12131=CARTESIAN_POINT ( 'NONE',  ( 9.509259942401945054, -25.80376675868338765, 25.15654267891509122 ) ) ;
#12141=EDGE_CURVE ( 'NONE', #20382, #25546, #16499, .T. ) ;
#12147=VERTEX_POINT ( 'NONE', #16456 ) ;
#12157=CARTESIAN_POINT ( 'NONE',  ( -10.14902473071754940, -26.01926976409365722, 87.93968498540000667 ) ) ;
#12165=LINE ( 'NONE', #9814, #10019 ) ;
#12174=EDGE_LOOP ( 'NONE', ( #17744, #28264, #26407, #30429, #9591, #5603, #24441, #23715, #13892, #23658 ) ) ;
#12179=ORIENTED_EDGE ( 'NONE', *, *, #9821, .T. ) ;
#12185=ORIENTED_EDGE ( 'NONE', *, *, #840, .F. ) ;
#12197=CARTESIAN_POINT ( 'NONE',  ( -2.332928517029999895E-09, 3.208345589200000119E-09, 230.0000000000000000 ) ) ;
#12201=ORIENTED_EDGE ( 'NONE', *, *, #26945, .F. ) ;
#12202=CARTESIAN_POINT ( 'NONE',  ( -26.80000000069999899, 3.281945028329999726E-15, 192.8898184869999852 ) ) ;
#12203=DIRECTION ( 'NONE',  ( -1.224606353819999829E-16, -1.000000000000000000, 0.000000000000000000 ) ) ;
#12210=CARTESIAN_POINT ( 'NONE',  ( -0.09707459355099370968, -26.79999999950000955, 226.1000000000000512 ) ) ;
#12215=CARTESIAN_POINT ( 'NONE',  ( -23.81569860410000317, -13.75000000000000000, 223.8999999999999773 ) ) ;
#12218=ORIENTED_EDGE ( 'NONE', *, *, #10034, .F. ) ;
#12226=VERTEX_POINT ( 'NONE', #3328 ) ;
#12227=DIRECTION ( 'NONE',  ( 0.9316362575375348731, -0.3633921898465292122, 0.000000000000000000 ) ) ;
#12241=LINE ( 'NONE', #9887, #3226 ) ;
#12258=AXIS2_PLACEMENT_3D ( 'NONE', #8592, #20725, #27637 ) ;
#12273=DIRECTION ( 'NONE',  ( 0.8090169943751909232, 0.5877852522921378498, 0.000000000000000000 ) ) ;
#12278=CARTESIAN_POINT ( 'NONE',  ( -23.06380069493458862, -13.64989377471593279, 6.071490516014675265 ) ) ;
#12283=TOROIDAL_SURFACE ( 'NONE', #16301, 30.50000000000000000, 3.000000000000000000 ) ;
#12289=EDGE_CURVE ( 'NONE', #17932, #10339, #25567, .T. ) ;
#12300=DIRECTION ( 'NONE',  ( 0.000000000000000000, 0.000000000000000000, 1.000000000000000000 ) ) ;
#12309=ORIENTED_EDGE ( 'NONE', *, *, #10289, .F. ) ;
#12313=ORIENTED_EDGE ( 'NONE', *, *, #14303, .T. ) ;
#12315=DIRECTION ( 'NONE',  ( 1.000000000000000000, 0.000000000000000000, 0.000000000000000000 ) ) ;
#12321=CIRCLE ( 'NONE', #4284, 26.80000000340000099 ) ;
#12323=EDGE_CURVE ( 'NONE', #14421, #13324, #27060, .T. ) ;
#12328=CYLINDRICAL_SURFACE ( 'NONE', #486, 26.80000000000002203 ) ;
#12347=ORIENTED_EDGE ( 'NONE', *, *, #224, .T. ) ;
#12352=EDGE_CURVE ( 'NONE', #22757, #20880, #23006, .T. ) ;
#12362=DIRECTION ( 'NONE',  ( 0.000000000000000000, 0.000000000000000000, 1.000000000000000000 ) ) ;
#12364=LINE ( 'NONE', #21973, #19290 ) ;
#12366=CARTESIAN_POINT ( 'NONE',  ( -2.373469614669185379, -26.70001233586149070, 210.0000000000000568 ) ) ;
#12369=CARTESIAN_POINT ( 'NONE',  ( 0.8360625678816901996, -27.48733645973267770, 4.281332030192536386 ) ) ;
#12377=EDGE_CURVE ( 'NONE', #26900, #24004, #13300, .T. ) ;
#12383=VERTEX_POINT ( 'NONE', #4115 ) ;
#12393=FACE_OUTER_BOUND ( 'NONE', #17137, .T. ) ;
#12402=DIRECTION ( 'NONE',  ( 0.3633921898465273803, -0.9316362575375355393, -1.040834085586083783E-14 ) ) ;
#12413=ORIENTED_EDGE ( 'NONE', *, *, #18793, .F. ) ;
#12417=ORIENTED_EDGE ( 'NONE', *, *, #23946, .T. ) ;
#12421=AXIS2_PLACEMENT_3D ( 'NONE', #23243, #20405, #18511 ) ;
#12423=ORIENTED_EDGE ( 'NONE', *, *, #22411, .F. ) ;
#12425=LINE ( 'NONE', #26908, #19300 ) ;
#12428=DIRECTION ( 'NONE',  ( 0.000000000000000000, 0.000000000000000000, 1.000000000000000000 ) ) ;
#12444=VERTEX_POINT ( 'NONE', #1767 ) ;
#12448=CARTESIAN_POINT ( 'NONE',  ( -23.20948082139999968, -13.40000000000000036, 223.8999999999999773 ) ) ;
#12449=CARTESIAN_POINT ( 'NONE',  ( 14.94562240850000023, -8.628859120750000500, 225.0000000000000000 ) ) ;
#12450=ORIENTED_EDGE ( 'NONE', *, *, #28078, .F. ) ;
#12452=ORIENTED_EDGE ( 'NONE', *, *, #20784, .T. ) ;
#12455=VECTOR ( 'NONE', #8461, 1000.000000000000000 ) ;
#12472=CARTESIAN_POINT ( 'NONE',  ( 1.019043873895764341, -27.48159911132826494, 5.420262664917122386 ) ) ;
#12477=TOROIDAL_SURFACE ( 'NONE', #27547, 24.50000000000000000, 4.000000000000000000 ) ;
#12482=ORIENTED_EDGE ( 'NONE', *, *, #20624, .F. ) ;
#12484=AXIS2_PLACEMENT_3D ( 'NONE', #31000, #9122, #21411 ) ;
#12495=CARTESIAN_POINT ( 'NONE',  ( -8.903108651239966420, -22.82508830966961000, 40.00000000000000000 ) ) ;
#12498=DIRECTION ( 'NONE',  ( 0.3633921898465276024, -0.9316362575375355393, 0.000000000000000000 ) ) ;
#12510=CARTESIAN_POINT ( 'NONE',  ( 26.80000000000000071, -1.776356839399999804E-15, 143.2171415880000040 ) ) ;
#12515=CARTESIAN_POINT ( 'NONE',  ( -3.918707624292968372, -26.51317744985242442, 209.7461278024016735 ) ) ;
#12522=CARTESIAN_POINT ( 'NONE',  ( -24.77829191970622702, -10.21159038398081087, 93.21714158839905906 ) ) ;
#12529=TOROIDAL_SURFACE ( 'NONE', #30122, 29.80000000000000071, 3.000000000000000000 ) ;
#12537=ORIENTED_EDGE ( 'NONE', *, *, #17662, .F. ) ;
#12541=CARTESIAN_POINT ( 'NONE',  ( -3.552713678799999608E-15, 0.000000000000000000, 143.2171415880000040 ) ) ;
#12545=DIRECTION ( 'NONE',  ( 1.000000000000000000, -1.224606353819999829E-16, 0.000000000000000000 ) ) ;
#12554=CARTESIAN_POINT ( 'NONE',  ( 0.6425564541914388084, -27.49266737062501065, 225.9130852755266403 ) ) ;
#12561=CARTESIAN_POINT ( 'NONE',  ( -26.93395386830000149, 3.298349104069999855E-15, 142.2432411360000231 ) ) ;
#12565=ORIENTED_EDGE ( 'NONE', *, *, #6373, .T. ) ;
#12573=ORIENTED_EDGE ( 'NONE', *, *, #10851, .F. ) ;
#12574=VERTEX_POINT ( 'NONE', #5352 ) ;
#12575=CIRCLE ( 'NONE', #16669, 2.999999999999999556 ) ;
#12579=CARTESIAN_POINT ( 'NONE',  ( -27.76135143630000002, 3.399672735959999724E-15, 87.66141409829998565 ) ) ;
#12580=DIRECTION ( 'NONE',  ( 0.8090169943751909232, 0.5877852522921378498, 0.000000000000000000 ) ) ;
#12589=EDGE_CURVE ( 'NONE', #25831, #27584, #9171, .T. ) ;
#12593=CARTESIAN_POINT ( 'NONE',  ( -23.25354871331287043, -14.68148953535444790, 225.2179249493744635 ) ) ;
#12605=CARTESIAN_POINT ( 'NONE',  ( 0.000000000000000000, 0.000000000000000000, 40.00000000000000000 ) ) ;
#12624=CARTESIAN_POINT ( 'NONE',  ( -8.903108651239966420, -22.82508830966961000, 90.00000000000000000 ) ) ;
#12625=CARTESIAN_POINT ( 'NONE',  ( -0.9565336352369326889, -27.48338672414943318, 5.548095501889124925 ) ) ;
#12626=CARTESIAN_POINT ( 'NONE',  ( -24.50000001620000134, 3.000285568850000245E-15, 139.9999999960000139 ) ) ;
#12629=B_SPLINE_CURVE_WITH_KNOTS ( 'NONE', 3,
 ( #24817, #29374, #22304, #8273, #22616, #3252, #5918, #7817, #27021, #17413 ),
 .UNSPECIFIED., .F., .F.,
 ( 4, 2, 2, 2, 4 ),
 ( 0.000000000000000000, 0.2500000000000000000, 0.5000000000000000000, 0.7500000000000000000, 1.000000000000000000 ),
 .UNSPECIFIED. ) ;
#12640=EDGE_CURVE ( 'NONE', #16404, #27663, #10237, .T. ) ;
#12641=CARTESIAN_POINT ( 'NONE',  ( 24.05715877174375095, -13.32261293489436227, 5.994883228945302456 ) ) ;
#12642=CIRCLE ( 'NONE', #26730, 27.50000000000000000 ) ;
#12643=VERTEX_POINT ( 'NONE', #3141 ) ;
#12646=AXIS2_PLACEMENT_3D ( 'NONE', #19557, #17341, #24433 ) ;
#12661=AXIS2_PLACEMENT_3D ( 'NONE', #959, #25017, #29892 ) ;
#12663=CARTESIAN_POINT ( 'NONE',  ( 16.20306687547020630, -21.42689369263764831, 36.78285841147714308 ) ) ;
#12665=CARTESIAN_POINT ( 'NONE',  ( -27.92857142820000149, 1.776356839399999804E-15, 187.9396849849999853 ) ) ;
#12667=CARTESIAN_POINT ( 'NONE',  ( 10.82908725742651512, -27.76276047461856322, 43.21714158840000408 ) ) ;
#12672=CARTESIAN_POINT ( 'NONE',  ( 1.099928585400369085, -27.47799405182496457, 4.854498941781074883 ) ) ;
#12676=CARTESIAN_POINT ( 'NONE',  ( -21.27344192715451499, -16.32329153680506195, 93.21714158846666010 ) ) ;
#12709=EDGE_CURVE ( 'NONE', #4812, #28386, #29729, .T. ) ;
#12711=CARTESIAN_POINT ( 'NONE',  ( 9.738910687886871642, -24.96785170200599069, 202.5331693087865403 ) ) ;
#12713=CARTESIAN_POINT ( 'NONE',  ( -24.77829191970622347, -10.21159038398080376, 43.21714158839912301 ) ) ;
#12720=CIRCLE ( 'NONE', #30324, 3.200000000000002398 ) ;
#12729=AXIS2_PLACEMENT_3D ( 'NONE', #17148, #22347, #25008 ) ;
#12734=DIRECTION ( 'NONE',  ( 0.000000000000000000, 0.000000000000000000, 1.000000000000000000 ) ) ;
#12735=CARTESIAN_POINT ( 'NONE',  ( 0.000000000000000000, 0.000000000000000000, 88.33953982530000815 ) ) ;
#12749=AXIS2_PLACEMENT_3D ( 'NONE', #5475, #5789, #22780 ) ;
#12759=DIRECTION ( 'NONE',  ( 0.3633921898465274913, -0.9316362575375355393, -0.000000000000000000 ) ) ;
#12760=CYLINDRICAL_SURFACE ( 'NONE', #241, 1.099999999999998979 ) ;
#12761=ADVANCED_FACE ( 'NONE', ( #23132 ), #12477, .T. ) ;
#12762=ORIENTED_EDGE ( 'NONE', *, *, #26063, .T. ) ;
#12767=ORIENTED_EDGE ( 'NONE', *, *, #25683, .F. ) ;
#12773=CIRCLE ( 'NONE', #4245, 2.999999999999999556 ) ;
#12778=AXIS2_PLACEMENT_3D ( 'NONE', #24245, #18903, #21430 ) ;
#12779=CIRCLE ( 'NONE', #12258, 4.000000004070001225 ) ;
#12781=B_SPLINE_CURVE_WITH_KNOTS ( 'NONE', 3,
 ( #27151, #10477, #29663, #8093, #15346, #15969, #16123, #27931, #4329, #14084 ),
 .UNSPECIFIED., .F., .F.,
 ( 4, 2, 2, 2, 4 ),
 ( 0.000000000000000000, 0.2500000000000000000, 0.5000000000000000000, 0.7500000000000000000, 1.000000000000000000 ),
 .UNSPECIFIED. ) ;
#12786=CARTESIAN_POINT ( 'NONE',  ( -26.80000000069999899, 3.281945028329999726E-15, 193.2171415869999862 ) ) ;
#12787=CARTESIAN_POINT ( 'NONE',  ( -2.962149026499999369E-14, -27.50000000069999828, 6.100000000000000533 ) ) ;
#12791=CARTESIAN_POINT ( 'NONE',  ( -10.06596365874885812, -25.80632433378972124, 190.0000000000000000 ) ) ;
#12792=CARTESIAN_POINT ( 'NONE',  ( 18.95046173579999760, -18.95046173579999760, 193.2171415880000040 ) ) ;
#12793=FACE_OUTER_BOUND ( 'NONE', #10643, .T. ) ;
#12794=CARTESIAN_POINT ( 'NONE',  ( 10.14902473071748545, -26.01926976409366077, 37.93968498539999956 ) ) ;
#12800=AXIS2_PLACEMENT_3D ( 'NONE', #9388, #10022, #2624 ) ;
#12813=VECTOR ( 'NONE', #13602, 1000.000000000000000 ) ;
#12815=DIRECTION ( 'NONE',  ( -0.9316362575375349842, 0.3633921898465292122, -0.000000000000000000 ) ) ;
#12820=DIRECTION ( 'NONE',  ( -0.3090169943750401549, -0.9510565162951233331, -1.149808922022230860E-31 ) ) ;
#12822=CARTESIAN_POINT ( 'NONE',  ( 0.1455402980897219090, -27.50000000000000711, 223.8999999999999773 ) ) ;
#12829=CARTESIAN_POINT ( 'NONE',  ( 0.000000000000000000, 0.000000000000000000, 90.00000000000000000 ) ) ;
#12832=DIRECTION ( 'NONE',  ( -0.8090169943751909232, 0.5877852522921378498, 0.000000000000000000 ) ) ;
#12833=CARTESIAN_POINT ( 'NONE',  ( 27.23548386990000125, -3.335274659639999982E-15, 141.6604601740000078 ) ) ;
#12843=CARTESIAN_POINT ( 'NONE',  ( -26.80000000069999899, 3.281945028329999726E-15, 87.11018146770000214 ) ) ;
#12845=ORIENTED_EDGE ( 'NONE', *, *, #12323, .T. ) ;
#12850=ORIENTED_EDGE ( 'NONE', *, *, #27103, .T. ) ;
#12857=CARTESIAN_POINT ( 'NONE',  ( -23.52368442185878195, -12.84078897091760929, 225.9137588022049385 ) ) ;
#12860=FACE_OUTER_BOUND ( 'NONE', #19239, .T. ) ;
#12861=CARTESIAN_POINT ( 'NONE',  ( -2.664535259099999568E-14, -26.80000000000000071, 115.0000000000000000 ) ) ;
#12864=CARTESIAN_POINT ( 'NONE',  ( -9.993285220779545952, -25.61999708228220740, 143.6055512749999821 ) ) ;
#12866=DIRECTION ( 'NONE',  ( 0.000000000000000000, 0.000000000000000000, -1.000000000000000000 ) ) ;
#12868=B_SPLINE_CURVE_WITH_KNOTS ( 'NONE', 3,
 ( #10474, #27605, #8717, #25573, #6206, #29660, #30128, #1031, #8090, #1182, #13606, #3852, #3688, #17681 ),
 .UNSPECIFIED., .F., .F.,
 ( 4, 2, 2, 2, 2, 2, 4 ),
 ( 0.000000000000000000, 0.2500000000000015543, 0.3750000000000019984, 0.4375000000000020539, 0.5000000000000021094, 0.7500000000000011102, 1.000000000000000000 ),
 .UNSPECIFIED. ) ;
#12874=CARTESIAN_POINT ( 'NONE',  ( 5.159343048259787068, -26.29982486972313183, 209.3149099368865791 ) ) ;
#12884=ORIENTED_EDGE ( 'NONE', *, *, #20600, .F. ) ;
#12906=DIRECTION ( 'NONE',  ( 1.000000000000000000, 0.000000000000000000, 0.000000000000000000 ) ) ;
#12909=CARTESIAN_POINT ( 'NONE',  ( -27.23548387100000312, 3.552713678799999608E-15, 38.33953982530000104 ) ) ;
#12910=DIRECTION ( 'NONE',  ( 0.3633921898465276024, -0.9316362575375355393, 2.168404344971008868E-14 ) ) ;
#12911=CARTESIAN_POINT ( 'NONE',  ( -27.50000000000000000, 3.552713678799999608E-15, 93.60555127549999099 ) ) ;
#12912=VERTEX_POINT ( 'NONE', #18027 ) ;
#12915=DIRECTION ( 'NONE',  ( 0.3633921898465274913, -0.9316362575375355393, -0.000000000000000000 ) ) ;
#12925=ORIENTED_EDGE ( 'NONE', *, *, #23939, .F. ) ;
#12926=CARTESIAN_POINT ( 'NONE',  ( 0.000000000000000000, 0.000000000000000000, 0.000000000000000000 ) ) ;
#12939=DIRECTION ( 'NONE',  ( 0.000000000000000000, 1.000000000000000000, 0.000000000000000000 ) ) ;
#12940=TOROIDAL_SURFACE ( 'NONE', #13430, 24.50000000000000000, 4.000000000000000000 ) ;
#12949=CARTESIAN_POINT ( 'NONE',  ( 23.70578532235928648, -13.93854223105014967, 223.9122931966472834 ) ) ;
#12970=FACE_OUTER_BOUND ( 'NONE', #20495, .T. ) ;
#12973=CARTESIAN_POINT ( 'NONE',  ( 0.5612683727491727392, -26.79446734626967341, 5.957452581394321101 ) ) ;
#12978=DIRECTION ( 'NONE',  ( -0.7071067811865475727, -0.7071067811865475727, 0.000000000000000000 ) ) ;
#12980=CARTESIAN_POINT ( 'NONE',  ( 27.06563794070000029, -3.314475219239999417E-15, 141.9402686260000053 ) ) ;
#12981=CARTESIAN_POINT ( 'NONE',  ( -9.481612630793593510, -25.06681236668577739, 204.0987691141152709 ) ) ;
#12989=CARTESIAN_POINT ( 'NONE',  ( -27.06563796540000411, 3.314475222269999560E-15, 88.05973140640000452 ) ) ;
#12991=AXIS2_PLACEMENT_3D ( 'NONE', #18507, #28109, #4350 ) ;
#12992=DIRECTION ( 'NONE',  ( 0.000000000000000000, 0.000000000000000000, 1.000000000000000000 ) ) ;
#12994=CYLINDRICAL_SURFACE ( 'NONE', #24748, 26.80000000000002203 ) ;
#12997=ORIENTED_EDGE ( 'NONE', *, *, #8643, .F. ) ;
#13000=AXIS2_PLACEMENT_3D ( 'NONE', #27483, #29700, #11134 ) ;
#13015=CARTESIAN_POINT ( 'NONE',  ( 23.64677485494184950, -12.61282738993112140, 4.366512952121566649 ) ) ;
#13021=CARTESIAN_POINT ( 'NONE',  ( 8.730899654840385438, -25.33966640892203159, 206.0387695587929215 ) ) ;
#13023=CARTESIAN_POINT ( 'NONE',  ( -20.77057278543776420, -16.95162108973865855, 43.21714158846112497 ) ) ;
#13025=CARTESIAN_POINT ( 'NONE',  ( 9.251510797979356937, -25.15273151106422844, 25.14734585054994653 ) ) ;
#13028=ORIENTED_EDGE ( 'NONE', *, *, #10851, .T. ) ;
#13032=ORIENTED_EDGE ( 'NONE', *, *, #106, .F. ) ;
#13033=EDGE_CURVE ( 'NONE', #5307, #21098, #15522, .T. ) ;
#13036=ORIENTED_EDGE ( 'NONE', *, *, #3135, .F. ) ;
#13047=CARTESIAN_POINT ( 'NONE',  ( -26.80000000069999899, 3.281945028329999726E-15, 93.21714158910000947 ) ) ;
#13067=ORIENTED_EDGE ( 'NONE', *, *, #22554, .T. ) ;
#13068=CARTESIAN_POINT ( 'NONE',  ( -8.982833346883255743, -25.99322455654492359, 23.95590625169068133 ) ) ;
#13072=DIRECTION ( 'NONE',  ( -1.000000000000000000, 5.665498452320000818E-16, 0.000000000000000000 ) ) ;
#13080=ORIENTED_EDGE ( 'NONE', *, *, #19559, .T. ) ;
#13088=DIRECTION ( 'NONE',  ( -0.3633921898465291567, -0.9316362575375348731, 0.000000000000000000 ) ) ;
#13091=DIRECTION ( 'NONE',  ( -0.9316362575375349842, 0.3633921898465292122, -0.000000000000000000 ) ) ;
#13102=ORIENTED_EDGE ( 'NONE', *, *, #23764, .T. ) ;
#13107=ORIENTED_EDGE ( 'NONE', *, *, #25408, .T. ) ;
#13124=ORIENTED_EDGE ( 'NONE', *, *, #17384, .T. ) ;
#13128=B_SPLINE_CURVE_WITH_KNOTS ( 'NONE', 3,
 ( #27859, #6142, #27543, #27393, #975, #10565, #20622, #24888, #17629, #6308, #8335, #5988, #25037, #8182, #22830, #13068, #15582, #24727, #3467, #25189, #11033, #3161, #29910, #10878 ),
 .UNSPECIFIED., .F., .F.,
 ( 4, 2, 2, 2, 2, 2, 2, 2, 2, 2, 2, 4 ),
 ( 8.673617379884035472E-19, 0.001576261392767898308, 0.002364392089151846378, 0.003152522785535794448, 0.004728784178303689287, 0.005516914874687638658, 0.006305045571071588896, 0.007881306963839485036, 0.009457568356607382043, 0.01024569905299133402, 0.01103382974937528599, 0.01261009114214319340 ),
 .UNSPECIFIED. ) ;
#13133=CARTESIAN_POINT ( 'NONE',  ( 27.63177371740000154, -3.383804566150000094E-15, 142.6394760449999808 ) ) ;
#13143=ADVANCED_FACE ( 'NONE', ( #14111 ), #7496, .T. ) ;
#13152=VERTEX_POINT ( 'NONE', #16149 ) ;
#13164=DIRECTION ( 'NONE',  ( -0.000000000000000000, -0.000000000000000000, -1.000000000000000000 ) ) ;
#13166=CARTESIAN_POINT ( 'NONE',  ( 21.30888436558567633, -16.34772642260384856, 86.78285841148333191 ) ) ;
#13175=EDGE_LOOP ( 'NONE', ( #14187, #4216, #23524, #524 ) ) ;
#13178=CARTESIAN_POINT ( 'NONE',  ( 18.95046173579999760, -18.95046173579999760, 115.0000000000000000 ) ) ;
#13185=LINE ( 'NONE', #15103, #9744 ) ;
#13194=CARTESIAN_POINT ( 'NONE',  ( 24.49999999589999788, -3.000285566359999846E-15, 140.0000000000000000 ) ) ;
#13212=ORIENTED_EDGE ( 'NONE', *, *, #22467, .F. ) ;
#13214=CARTESIAN_POINT ( 'NONE',  ( 0.000000000000000000, 0.000000000000000000, 140.0000000000000000 ) ) ;
#13220=EDGE_LOOP ( 'NONE', ( #22330, #5764, #25581, #1716 ) ) ;
#13223=CARTESIAN_POINT ( 'NONE',  ( 0.000000000000000000, 0.000000000000000000, 20.00000000000000000 ) ) ;
#13229=DIRECTION ( 'NONE',  ( 0.000000000000000000, 0.000000000000000000, 1.000000000000000000 ) ) ;
#13230=CARTESIAN_POINT ( 'NONE',  ( -20.19490051663601093, -17.70600380938601148, 0.000000000000000000 ) ) ;
#13236=CIRCLE ( 'NONE', #27330, 26.80000000000000071 ) ;
#13238=CARTESIAN_POINT ( 'NONE',  ( -1.100000000000000089, -27.47799119230000287, 5.000000000000000000 ) ) ;
#13242=CARTESIAN_POINT ( 'NONE',  ( -23.32129337769715960, -14.57293380285341655, 224.4438356449677485 ) ) ;
#13247=CARTESIAN_POINT ( 'NONE',  ( -2.664535259099999568E-14, -26.80000000000000071, 210.0000000000000284 ) ) ;
#13248=ORIENTED_EDGE ( 'NONE', *, *, #17338, .T. ) ;
#13255=CARTESIAN_POINT ( 'NONE',  ( 26.93395402219999824, -3.298349122899999616E-15, 137.7567592739999895 ) ) ;
#13260=CIRCLE ( 'NONE', #24324, 4.000000000000000888 ) ;
#13261=VERTEX_POINT ( 'NONE', #2312 ) ;
#13263=VERTEX_POINT ( 'NONE', #11895 ) ;
#13267=ORIENTED_EDGE ( 'NONE', *, *, #4639, .T. ) ;
#13282=CARTESIAN_POINT ( 'NONE',  ( -3.907985046680000082E-14, -26.80000000000000071, 6.099999999630000502 ) ) ;
#13284=FACE_OUTER_BOUND ( 'NONE', #202, .T. ) ;
#13293=DIRECTION ( 'NONE',  ( -1.000000000000000000, 5.665498452320000818E-16, 0.000000000000000000 ) ) ;
#13297=CARTESIAN_POINT ( 'NONE',  ( 26.80000000069999899, -3.281945028320000125E-15, 186.7828584129999854 ) ) ;
#13300=B_SPLINE_CURVE_WITH_KNOTS ( 'NONE', 5,
 ( #6156, #6322, #13395, #3483, #22687, #3807 ),
 .UNSPECIFIED., .F., .F.,
 ( 6, 6 ),
 ( 0.000000000000000000, 2.319814964739999930 ),
 .UNSPECIFIED. ) ;
#13302=AXIS2_PLACEMENT_3D ( 'NONE', #21219, #13672, #16644 ) ;
#13304=CARTESIAN_POINT ( 'NONE',  ( -10.82908725742656308, -27.76276047461853835, 43.21714158840000408 ) ) ;
#13311=ORIENTED_EDGE ( 'NONE', *, *, #13554, .F. ) ;
#13316=CARTESIAN_POINT ( 'NONE',  ( -23.20948082139999968, -13.40000000000000036, 6.099999999630000502 ) ) ;
#13324=VERTEX_POINT ( 'NONE', #422 ) ;
#13342=CARTESIAN_POINT ( 'NONE',  ( 3.664716979113602946, -26.54951320538905080, 20.19324488679039931 ) ) ;
#13343=ORIENTED_EDGE ( 'NONE', *, *, #27570, .F. ) ;
#13346=ORIENTED_EDGE ( 'NONE', *, *, #8892, .F. ) ;
#13351=VERTEX_POINT ( 'NONE', #3064 ) ;
#13354=DIRECTION ( 'NONE',  ( 1.000000000000000000, 0.000000000000000000, 0.000000000000000000 ) ) ;
#13379=CARTESIAN_POINT ( 'NONE',  ( -22.68420274106557599, -14.27219891856329781, 224.5770195892032177 ) ) ;
#13381=CARTESIAN_POINT ( 'NONE',  ( 1.087555312692434661, -26.77834283312493824, 4.781945490036553004 ) ) ;
#13386=ORIENTED_EDGE ( 'NONE', *, *, #4297, .F. ) ;
#13393=DIRECTION ( 'NONE',  ( 0.8090169943751909232, 0.5877852522921378498, 0.000000000000000000 ) ) ;
#13395=CARTESIAN_POINT ( 'NONE',  ( 26.93395402219999824, -3.298349122909999612E-15, 187.7567592740000180 ) ) ;
#13400=CARTESIAN_POINT ( 'NONE',  ( -6.112318018889845384, -26.81313817375427178, 208.9612952676429245 ) ) ;
#13408=CARTESIAN_POINT ( 'NONE',  ( -27.69999999930000101, 3.392159599999999562E-15, 90.00000000000000000 ) ) ;
#13409=VERTEX_POINT ( 'NONE', #28726 ) ;
#13417=ORIENTED_EDGE ( 'NONE', *, *, #28501, .F. ) ;
#13421=CARTESIAN_POINT ( 'NONE',  ( -7.105427357599999217E-15, -7.105427357599999217E-15, 36.78285841159999592 ) ) ;
#13423=DIRECTION ( 'NONE',  ( 0.000000000000000000, 0.000000000000000000, 1.000000000000000000 ) ) ;
#13424=B_SPLINE_CURVE_WITH_KNOTS ( 'NONE', 3,
 ( #7928, #5421, #9682, #5112, #19597, #29176, #5272, #571, #19750, #12048 ),
 .UNSPECIFIED., .F., .F.,
 ( 4, 2, 2, 2, 4 ),
 ( 0.000000000000000000, 0.2500000000000000000, 0.5000000000000000000, 0.7500000000000000000, 1.000000000000000000 ),
 .UNSPECIFIED. ) ;
#13430=AXIS2_PLACEMENT_3D ( 'NONE', #10041, #304, #9722 ) ;
#13434=ORIENTED_EDGE ( 'NONE', *, *, #26012, .F. ) ;
#13436=CYLINDRICAL_SURFACE ( 'NONE', #21527, 27.50000000000000000 ) ;
#13444=CARTESIAN_POINT ( 'NONE',  ( 9.944224317832768278, -25.63928765730900139, 26.94315197391175332 ) ) ;
#13445=CARTESIAN_POINT ( 'NONE',  ( -9.738910687886857431, -24.96785170200598714, 202.5331423531274311 ) ) ;
#13450=EDGE_CURVE ( 'NONE', #11773, #15620, #27494, .T. ) ;
#13455=AXIS2_PLACEMENT_3D ( 'NONE', #16943, #128, #7649 ) ;
#13457=CIRCLE ( 'NONE', #432, 4.000000004070001225 ) ;
#13458=DIRECTION ( 'NONE',  ( 1.000000000000000000, 0.000000000000000000, 0.000000000000000000 ) ) ;
#13465=ORIENTED_EDGE ( 'NONE', *, *, #5330, .F. ) ;
#13473=AXIS2_PLACEMENT_3D ( 'NONE', #28100, #8899, #15986 ) ;
#13475=VECTOR ( 'NONE', #21191, 1000.000000000000000 ) ;
#13487=CARTESIAN_POINT ( 'NONE',  ( -1.099929244070900536, -27.47799402545702563, 225.1456731700734792 ) ) ;
#13492=CARTESIAN_POINT ( 'NONE',  ( -23.24663841807413434, -14.69162354064478571, 5.096459710828290746 ) ) ;
#13495=AXIS2_PLACEMENT_3D ( 'NONE', #30544, #8972, #25511 ) ;
#13497=CARTESIAN_POINT ( 'NONE',  ( -23.86403265537058616, -13.66628296746374893, 223.9000000000011426 ) ) ;
#13511=VECTOR ( 'NONE', #27333, 1000.000000000000000 ) ;
#13512=ADVANCED_FACE ( 'NONE', ( #13284 ), #18008, .T. ) ;
#13519=DIRECTION ( 'NONE',  ( -1.224606353819999829E-16, -1.000000000000000000, 0.000000000000000000 ) ) ;
#13525=CARTESIAN_POINT ( 'NONE',  ( -10.14902473054660348, -26.01926976365539090, 137.9396849850000137 ) ) ;
#13528=DIRECTION ( 'NONE',  ( 0.3633921898465289901, 0.9316362575375348731, -1.734723475976805832E-14 ) ) ;
#13531=CYLINDRICAL_SURFACE ( 'NONE', #29322, 26.80000000000002203 ) ;
#13537=DIRECTION ( 'NONE',  ( 0.000000000000000000, -0.000000000000000000, 1.000000000000000000 ) ) ;
#13551=DIRECTION ( 'NONE',  ( 0.000000000000000000, 0.000000000000000000, 1.000000000000000000 ) ) ;
#13554=EDGE_CURVE ( 'NONE', #18252, #9397, #11558, .T. ) ;
#13557=CARTESIAN_POINT ( 'NONE',  ( -27.23548386990000125, 3.335274659649999582E-15, 138.3395398259999922 ) ) ;
#13563=CARTESIAN_POINT ( 'NONE',  ( -5.654928157491454499, -26.91331636611315759, 209.2041907114654862 ) ) ;
#13575=CARTESIAN_POINT ( 'NONE',  ( -13.11056599509667464, -23.44705117439653819, 36.78285841135430445 ) ) ;
#13577=CARTESIAN_POINT ( 'NONE',  ( -24.83284505762695815, -10.07844553579556823, 93.21714158839638742 ) ) ;
#13579=ORIENTED_EDGE ( 'NONE', *, *, #19236, .F. ) ;
#13581=CARTESIAN_POINT ( 'NONE',  ( 26.80000000069999899, -3.281945028320000125E-15, 186.7828584129999854 ) ) ;
#13582=VERTEX_POINT ( 'NONE', #11091 ) ;
#13587=DIRECTION ( 'NONE',  ( 0.3090169943750400994, -0.9510565162951234441, 0.000000000000000000 ) ) ;
#13591=VECTOR ( 'NONE', #12428, 1000.000000000000000 ) ;
#13596=CARTESIAN_POINT ( 'NONE',  ( -1.099927927707951447, -26.77741881808350044, 224.8541214485396722 ) ) ;
#13599=ORIENTED_EDGE ( 'NONE', *, *, #4593, .F. ) ;
#13602=DIRECTION ( 'NONE',  ( 1.000000000000000000, -1.224606353819999829E-16, 0.000000000000000000 ) ) ;
#13604=ORIENTED_EDGE ( 'NONE', *, *, #7405, .F. ) ;
#13606=CARTESIAN_POINT ( 'NONE',  ( -22.95800506017165077, -13.82601854610103409, 4.006804826634700945 ) ) ;
#13607=DIRECTION ( 'NONE',  ( 0.3633921898465273803, -0.9316362575375355393, -2.081668171172167567E-14 ) ) ;
#13611=CARTESIAN_POINT ( 'NONE',  ( 27.23548386990000125, -3.335274659639999982E-15, 191.6604601740000078 ) ) ;
#13613=EDGE_LOOP ( 'NONE', ( #2407, #30814, #17228, #11885 ) ) ;
#13614=ADVANCED_FACE ( 'NONE', ( #25570 ), #27593, .T. ) ;
#13620=ADVANCED_FACE ( 'NONE', ( #16578 ), #15527, .F. ) ;
#13623=CIRCLE ( 'NONE', #19643, 3.000000000000001332 ) ;
#13629=ORIENTED_EDGE ( 'NONE', *, *, #30930, .T. ) ;
#13633=EDGE_CURVE ( 'NONE', #8882, #27430, #12165, .T. ) ;
#13634=CARTESIAN_POINT ( 'NONE',  ( -27.23548386990000125, 3.335274659649999582E-15, 188.3395398260000206 ) ) ;
#13641=ORIENTED_EDGE ( 'NONE', *, *, #80, .T. ) ;
#13656=EDGE_CURVE ( 'NONE', #17696, #6778, #11018, .T. ) ;
#13657=CARTESIAN_POINT ( 'NONE',  ( -2.947640775130000104E-14, -27.50000000000000000, 223.8999999999999773 ) ) ;
#13658=ORIENTED_EDGE ( 'NONE', *, *, #18659, .F. ) ;
#13660=ORIENTED_EDGE ( 'NONE', *, *, #29983, .F. ) ;
#13666=EDGE_LOOP ( 'NONE', ( #15571, #3788, #4623, #6544, #462 ) ) ;
#13667=EDGE_CURVE ( 'NONE', #6732, #25385, #27905, .T. ) ;
#13672=DIRECTION ( 'NONE',  ( 0.000000000000000000, 0.000000000000000000, 1.000000000000000000 ) ) ;
#13674=CARTESIAN_POINT ( 'NONE',  ( -3.552713678799999608E-15, 0.000000000000000000, 43.21714158840000408 ) ) ;
#13677=VERTEX_POINT ( 'NONE', #2578 ) ;
#13678=CARTESIAN_POINT ( 'NONE',  ( 9.993285220779439371, -25.61999708228226069, 115.0000000000000000 ) ) ;
#13679=EDGE_CURVE ( 'NONE', #7142, #22455, #20766, .T. ) ;
#13691=ADVANCED_FACE ( 'NONE', ( #2731 ), #12328, .F. ) ;
#13692=DIRECTION ( 'NONE',  ( 1.000000000000000000, 0.000000000000000000, 0.000000000000000000 ) ) ;
#13694=VERTEX_POINT ( 'NONE', #7748 ) ;
#13697=AXIS2_PLACEMENT_3D ( 'NONE', #14480, #16982, #29518 ) ;
#13702=EDGE_CURVE ( 'NONE', #4180, #902, #14044, .T. ) ;
#13707=AXIS2_PLACEMENT_3D ( 'NONE', #82, #11565, #16893 ) ;
#13708=CARTESIAN_POINT ( 'NONE',  ( -2.962149026499999369E-14, -27.50000000069999828, 6.100000000000000533 ) ) ;
#13713=CARTESIAN_POINT ( 'NONE',  ( 23.61599683838066710, -12.66993935541866634, 5.719315393927735691 ) ) ;
#13719=CARTESIAN_POINT ( 'NONE',  ( -23.53911279557259206, -12.81252279922326132, 224.1183286170036411 ) ) ;
#13735=ORIENTED_EDGE ( 'NONE', *, *, #22900, .T. ) ;
#13737=DIRECTION ( 'NONE',  ( 0.000000000000000000, 0.000000000000000000, -1.000000000000000000 ) ) ;
#13745=CARTESIAN_POINT ( 'NONE',  ( 23.34643930336224216, -14.53345043318084251, 4.357489521687117673 ) ) ;
#13751=CARTESIAN_POINT ( 'NONE',  ( -23.20948082139999968, -13.40000000000000036, 6.099999999630000502 ) ) ;
#13753=CARTESIAN_POINT ( 'NONE',  ( -23.20948082139999968, -13.40000000000000036, 226.0999999999999943 ) ) ;
#13755=DIRECTION ( 'NONE',  ( 0.000000000000000000, 0.000000000000000000, 1.000000000000000000 ) ) ;
#13756=DIRECTION ( 'NONE',  ( -0.000000000000000000, -0.000000000000000000, -1.000000000000000000 ) ) ;
#13758=CARTESIAN_POINT ( 'NONE',  ( 26.80000000069999899, -3.281945028320000125E-15, 211.6085707940000020 ) ) ;
#13759=FACE_OUTER_BOUND ( 'NONE', #30252, .T. ) ;
#13770=AXIS2_PLACEMENT_3D ( 'NONE', #5827, #1115, #20155 ) ;
#13771=CIRCLE ( 'NONE', #24303, 2.999999999999999556 ) ;
#13772=AXIS2_PLACEMENT_3D ( 'NONE', #26446, #24548, #12273 ) ;
#13776=CARTESIAN_POINT ( 'NONE',  ( -24.08956650190513571, -13.26503430085140955, 225.9595466043619751 ) ) ;
#13778=ORIENTED_EDGE ( 'NONE', *, *, #28078, .T. ) ;
#13789=AXIS2_PLACEMENT_3D ( 'NONE', #23188, #23348, #8688 ) ;
#13816=EDGE_LOOP ( 'NONE', ( #12309, #14837, #3395, #15424 ) ) ;
#13818=VERTEX_POINT ( 'NONE', #20487 ) ;
#13821=ORIENTED_EDGE ( 'NONE', *, *, #13450, .T. ) ;
#13824=CARTESIAN_POINT ( 'NONE',  ( 26.80000000000000071, -1.776356839399999804E-15, 43.21714158840000408 ) ) ;
#13829=FACE_OUTER_BOUND ( 'NONE', #25981, .T. ) ;
#13831=B_SPLINE_CURVE_WITH_KNOTS ( 'NONE', 5,
 ( #22696, #24909, #27884, #25211, #27718, #17649 ),
 .UNSPECIFIED., .F., .F.,
 ( 6, 6 ),
 ( 0.000000000000000000, 2.300779717540000213 ),
 .UNSPECIFIED. ) ;
#13834=CARTESIAN_POINT ( 'NONE',  ( 27.50000000000000000, -3.367667472999999580E-15, 93.60555127639999284 ) ) ;
#13837=ORIENTED_EDGE ( 'NONE', *, *, #24595, .F. ) ;
#13848=DIRECTION ( 'NONE',  ( 0.000000000000000000, 0.000000000000000000, 1.000000000000000000 ) ) ;
#13853=DIRECTION ( 'NONE',  ( -1.224606353819999829E-16, -1.000000000000000000, 0.000000000000000000 ) ) ;
#13862=EDGE_CURVE ( 'NONE', #10144, #6778, #28943, .T. ) ;
#13864=VERTEX_POINT ( 'NONE', #17648 ) ;
#13870=DIRECTION ( 'NONE',  ( -1.000000000000000000, 5.665498452320000818E-16, 0.000000000000000000 ) ) ;
#13879=CARTESIAN_POINT ( 'NONE',  ( 23.81569860410000317, -13.75000000000000000, 226.0999999999999943 ) ) ;
#13880=CARTESIAN_POINT ( 'NONE',  ( -23.63672937765306159, -12.63153181569432881, 224.3233986254962815 ) ) ;
#13883=LINE ( 'NONE', #21122, #20856 ) ;
#13884=EDGE_CURVE ( 'NONE', #5307, #28386, #2460, .T. ) ;
#13885=DIRECTION ( 'NONE',  ( 0.000000000000000000, 0.000000000000000000, -1.000000000000000000 ) ) ;
#13892=ORIENTED_EDGE ( 'NONE', *, *, #13884, .T. ) ;
#13895=ORIENTED_EDGE ( 'NONE', *, *, #1586, .T. ) ;
#13909=CARTESIAN_POINT ( 'NONE',  ( -1.071233843433221589, -26.77863813582381525, 224.7119040166546995 ) ) ;
#13914=CARTESIAN_POINT ( 'NONE',  ( -22.65536946396631279, -14.31703147662669018, 225.2878164648193149 ) ) ;
#13917=CARTESIAN_POINT ( 'NONE',  ( 21.30571717078112215, -16.35234564651914013, -0.000000000000000000 ) ) ;
#13931=CARTESIAN_POINT ( 'NONE',  ( 0.000000000000000000, 0.000000000000000000, 20.00000000000000355 ) ) ;
#13937=CARTESIAN_POINT ( 'NONE',  ( 10.06596365874881194, -25.80632433378973900, 90.00000000000000000 ) ) ;
#13948=SURFACE_STYLE_USAGE ( .BOTH. , #9209 ) ;
#13954=AXIS2_PLACEMENT_3D ( 'NONE', #28455, #23750, #6890 ) ;
#13962=CIRCLE ( 'NONE', #7894, 27.92857142820000149 ) ;
#13966=TOROIDAL_SURFACE ( 'NONE', #28532, 24.50000000000000000, 4.000000000000000000 ) ;
#13983=AXIS2_PLACEMENT_3D ( 'NONE', #26193, #16434, #25893 ) ;
#13989=B_SPLINE_CURVE_WITH_KNOTS ( 'NONE', 3,
 ( #5625, #768, #13166, #10513, #20112, #22473, #3109, #22163, #15226, #10660 ),
 .UNSPECIFIED., .F., .F.,
 ( 4, 2, 2, 2, 4 ),
 ( 0.000000000000000000, 0.2499999999999998890, 0.4999999999999997780, 0.7499999999999998890, 1.000000000000000000 ),
 .UNSPECIFIED. ) ;
#13993=CARTESIAN_POINT ( 'NONE',  ( 27.76135144259999876, -3.399672736709999763E-15, 92.33858589269999584 ) ) ;
#14006=DIRECTION ( 'NONE',  ( -0.7071067811865475727, -0.7071067811865475727, 0.000000000000000000 ) ) ;
#14014=DIRECTION ( 'NONE',  ( 1.000000000000000000, 0.000000000000000000, 0.000000000000000000 ) ) ;
#14015=DIRECTION ( 'NONE',  ( 0.000000000000000000, 0.000000000000000000, 1.000000000000000000 ) ) ;
#14020=EDGE_CURVE ( 'NONE', #17448, #12574, #18018, .T. ) ;
#14023=ORIENTED_EDGE ( 'NONE', *, *, #12640, .T. ) ;
#14039=DIRECTION ( 'NONE',  ( 0.000000000000000000, 0.000000000000000000, 1.000000000000000000 ) ) ;
#14043=DIRECTION ( 'NONE',  ( 0.3633921898465289901, 0.9316362575375348731, 4.336808689942014581E-15 ) ) ;
#14044=CIRCLE ( 'NONE', #1975, 3.000000000000001332 ) ;
#14055=EDGE_LOOP ( 'NONE', ( #4007, #30185, #20237, #1486 ) ) ;
#14060=EDGE_CURVE ( 'NONE', #22441, #5682, #22012, .T. ) ;
#14071=ORIENTED_EDGE ( 'NONE', *, *, #1945, .T. ) ;
#14074=CIRCLE ( 'NONE', #25625, 26.80000000000000071 ) ;
#14076=CARTESIAN_POINT ( 'NONE',  ( 23.26050567054135243, -13.42703864535239155, -0.000000000000000000 ) ) ;
#14077=ADVANCED_FACE ( 'NONE', ( #2809 ), #18532, .F. ) ;
#14084=CARTESIAN_POINT ( 'NONE',  ( -23.81569860410000317, -13.75000000000000000, 3.900000000369999942 ) ) ;
#14095=DIRECTION ( 'NONE',  ( 0.000000000000000000, 0.000000000000000000, 1.000000000000000000 ) ) ;
#14102=CYLINDRICAL_SURFACE ( 'NONE', #10404, 8.000000000000000000 ) ;
#14111=FACE_OUTER_BOUND ( 'NONE', #21884, .T. ) ;
#14116=DIRECTION ( 'NONE',  ( 0.000000000000000000, 0.000000000000000000, 1.000000000000000000 ) ) ;
#14117=DIRECTION ( 'NONE',  ( 1.000000000000000000, 0.000000000000000000, 0.000000000000000000 ) ) ;
#14126=EDGE_CURVE ( 'NONE', #23934, #29406, #22207, .T. ) ;
#14127=ORIENTED_EDGE ( 'NONE', *, *, #9235, .F. ) ;
#14139=EDGE_LOOP ( 'NONE', ( #29744, #26469, #30757, #18416 ) ) ;
#14149=ORIENTED_EDGE ( 'NONE', *, *, #17683, .F. ) ;
#14161=CARTESIAN_POINT ( 'NONE',  ( 27.76135143710000008, -3.399672736040000081E-15, 187.6614141010000196 ) ) ;
#14167=AXIS2_PLACEMENT_3D ( 'NONE', #14530, #28682, #24270 ) ;
#14169=VECTOR ( 'NONE', #28687, 1000.000000000000000 ) ;
#14171=EDGE_LOOP ( 'NONE', ( #25190, #6926, #30218, #28392 ) ) ;
#14183=DIRECTION ( 'NONE',  ( 0.000000000000000000, 0.000000000000000000, 1.000000000000000000 ) ) ;
#14186=EDGE_CURVE ( 'NONE', #25078, #4771, #25578, .T. ) ;
#14187=ORIENTED_EDGE ( 'NONE', *, *, #2318, .F. ) ;
#14191=CARTESIAN_POINT ( 'NONE',  ( 23.73988791505310303, -12.43614577697740486, 225.1459679062442660 ) ) ;
#14195=EDGE_CURVE ( 'NONE', #17360, #23934, #24210, .T. ) ;
#14196=B_SPLINE_CURVE_WITH_KNOTS ( 'NONE', 3,
 ( #873, #10930, #17675, #10768, #3216, #8086, #3367, #15339, #12973, #29802, #20369, #13282 ),
 .UNSPECIFIED., .F., .F.,
 ( 4, 2, 2, 2, 2, 4 ),
 ( 0.000000000000000000, 0.2500000000000013878, 0.3750000000000012212, 0.5000000000000011102, 0.7500000000000005551, 1.000000000000000000 ),
 .UNSPECIFIED. ) ;
#14204=VERTEX_POINT ( 'NONE', #20111 ) ;
#14228=CARTESIAN_POINT ( 'NONE',  ( 0.4949169532526843107, -27.49533956265200629, 5.993098012594048285 ) ) ;
#14235=DIRECTION ( 'NONE',  ( -0.9316362575375349842, 0.3633921898465292122, -0.000000000000000000 ) ) ;
#14236=DIRECTION ( 'NONE',  ( 1.000000000000000000, 0.000000000000000000, 0.000000000000000000 ) ) ;
#14238=ORIENTED_EDGE ( 'NONE', *, *, #29277, .F. ) ;
#14243=DIRECTION ( 'NONE',  ( -0.8090169943751909232, 0.5877852522921378498, 0.000000000000000000 ) ) ;
#14250=AXIS2_PLACEMENT_3D ( 'NONE', #17627, #5523, #521 ) ;
#14251=VERTEX_POINT ( 'NONE', #5780 ) ;
#14254=B_SPLINE_CURVE_WITH_KNOTS ( 'NONE', 3,
 ( #29052, #4672, #439, #21984, #17092, #10021, #19616, #29198, #23888, #7645 ),
 .UNSPECIFIED., .F., .F.,
 ( 4, 2, 2, 2, 4 ),
 ( 0.000000000000000000, 0.2500000000000000000, 0.5000000000000000000, 0.7500000000000000000, 1.000000000000000000 ),
 .UNSPECIFIED. ) ;
#14264=ADVANCED_FACE ( 'NONE', ( #17723 ), #21061, .F. ) ;
#14269=CARTESIAN_POINT ( 'NONE',  ( -3.552713678799999608E-15, -3.552713678799999608E-15, 93.21714158839999698 ) ) ;
#14293=AXIS2_PLACEMENT_3D ( 'NONE', #4435, #14039, #23792 ) ;
#14297=ORIENTED_EDGE ( 'NONE', *, *, #14976, .F. ) ;
#14303=EDGE_CURVE ( 'NONE', #8486, #26548, #26581, .T. ) ;
#14304=CARTESIAN_POINT ( 'NONE',  ( -30.50000000000000000, 2.720046410330000188E-15, 36.39444872449999480 ) ) ;
#14318=DIRECTION ( 'NONE',  ( -1.000000000000000000, 0.000000000000000000, 0.000000000000000000 ) ) ;
#14319=AXIS2_PLACEMENT_3D ( 'NONE', #3741, #10211, #27041 ) ;
#14350=ORIENTED_EDGE ( 'NONE', *, *, #24288, .T. ) ;
#14351=EDGE_CURVE ( 'NONE', #9711, #27663, #3958, .T. ) ;
#14364=DIRECTION ( 'NONE',  ( 1.000000000000000000, 0.000000000000000000, 0.000000000000000000 ) ) ;
#14377=CARTESIAN_POINT ( 'NONE',  ( 26.80000000069999899, -3.281945028320000125E-15, 230.0000000000000000 ) ) ;
#14384=ORIENTED_EDGE ( 'NONE', *, *, #16439, .T. ) ;
#14389=CARTESIAN_POINT ( 'NONE',  ( 0.9877995823961871480, -27.48272658602460083, 5.490987494730114271 ) ) ;
#14394=CARTESIAN_POINT ( 'NONE',  ( 8.903108651239925564, -22.82508830966962421, 140.0000000000000000 ) ) ;
#14395=CARTESIAN_POINT ( 'NONE',  ( -1.421085471519999843E-14, -1.421085471519999843E-14, 37.93968498539999956 ) ) ;
#14403=ORIENTED_EDGE ( 'NONE', *, *, #24459, .F. ) ;
#14417=DIRECTION ( 'NONE',  ( -0.9316362575375349842, 0.3633921898465292122, -0.000000000000000000 ) ) ;
#14421=VERTEX_POINT ( 'NONE', #23419 ) ;
#14422=CARTESIAN_POINT ( 'NONE',  ( 1.100000000000000089, -17.25771824079999917, 5.000000000000000000 ) ) ;
#14440=FACE_OUTER_BOUND ( 'NONE', #8725, .T. ) ;
#14442=B_SPLINE_CURVE_WITH_KNOTS ( 'NONE', 3,
 ( #19348, #16978, #26583, #13342, #24987, #19814, #17888, #27350, #17587, #1077, #3272, #10668, #10523, #27197, #15539, #17733, #20263, #13025, #3746, #24683, #5792, #29860, #3117, #22634 ),
 .UNSPECIFIED., .F., .F.,
 ( 4, 2, 2, 2, 2, 2, 2, 2, 2, 2, 2, 4 ),
 ( 6.505213034913026604E-19, 0.001577043753785921246, 0.002365565630678883279, 0.003154087507571844660, 0.004731131261357764822, 0.005519653138250724470, 0.006308175015143684117, 0.007885218768929599942, 0.009462262522715517502, 0.01025078439960847194, 0.01103930627650142639, 0.01261635003028733874 ),
 .UNSPECIFIED. ) ;
#14454=CIRCLE ( 'NONE', #19480, 27.23548387100000312 ) ;
#14455=CIRCLE ( 'NONE', #27003, 4.000000004070001225 ) ;
#14476=CARTESIAN_POINT ( 'NONE',  ( 0.000000000000000000, 0.000000000000000000, 190.0000000000000000 ) ) ;
#14480=CARTESIAN_POINT ( 'NONE',  ( 0.000000000000000000, 0.000000000000000000, 115.0000000000000000 ) ) ;
#14492=DIRECTION ( 'NONE',  ( 0.3633921898465292122, 0.9316362575375348731, -1.387778780781445360E-14 ) ) ;
#14493=CARTESIAN_POINT ( 'NONE',  ( -9.993285220779425160, -25.61999708228226069, 115.0000000000000000 ) ) ;
#14506=DIRECTION ( 'NONE',  ( 0.5000000000001898481, -0.8660254037843291286, 0.000000000000000000 ) ) ;
#14508=CARTESIAN_POINT ( 'NONE',  ( -23.24663841807413434, -14.69162354064478215, 225.0964597109269221 ) ) ;
#14519=CARTESIAN_POINT ( 'NONE',  ( 26.80000000069999899, -3.281945028320000125E-15, 136.7828584130000138 ) ) ;
#14524=ORIENTED_EDGE ( 'NONE', *, *, #17758, .T. ) ;
#14529=ADVANCED_FACE ( 'NONE', ( #19299 ), #15513, .T. ) ;
#14530=CARTESIAN_POINT ( 'NONE',  ( -3.552713678799999608E-15, -3.552713678799999608E-15, 93.21714158839999698 ) ) ;
#14538=ORIENTED_EDGE ( 'NONE', *, *, #13884, .F. ) ;
#14544=DIRECTION ( 'NONE',  ( 0.000000000000000000, 0.000000000000000000, 1.000000000000000000 ) ) ;
#14547=CARTESIAN_POINT ( 'NONE',  ( 22.64694720651011650, -14.33102249085027680, 5.218051573047087111 ) ) ;
#14554=AXIS2_PLACEMENT_3D ( 'NONE', #4782, #30903, #9805 ) ;
#14565=CARTESIAN_POINT ( 'NONE',  ( -3.552713678799999608E-15, 0.000000000000000000, 143.2171415880000040 ) ) ;
#14569=DIRECTION ( 'NONE',  ( -1.224606353819999829E-16, -1.000000000000000000, 0.000000000000000000 ) ) ;
#14582=EDGE_CURVE ( 'NONE', #10785, #19471, #1168, .T. ) ;
#14590=CARTESIAN_POINT ( 'NONE',  ( -0.8178280288081285487, -26.78758467685877775, 225.7372270131871517 ) ) ;
#14605=CARTESIAN_POINT ( 'NONE',  ( 7.453090060300407771, -2.907137518772282991, 27.99999999999999645 ) ) ;
#14612=CARTESIAN_POINT ( 'NONE',  ( -9.993285220779547728, -25.61999708228220030, 43.60555127550000520 ) ) ;
#14615=ORIENTED_EDGE ( 'NONE', *, *, #15641, .T. ) ;
#14620=DIRECTION ( 'NONE',  ( 0.3633921898465289901, 0.9316362575375348731, -2.168404344971007290E-15 ) ) ;
#14629=B_SPLINE_CURVE_WITH_KNOTS ( 'NONE', 3,
 ( #8862, #13596, #13909, #30117, #1643, #25721, #8546, #11233, #23364, #30742, #27748, #20837 ),
 .UNSPECIFIED., .F., .F.,
 ( 4, 2, 2, 2, 2, 4 ),
 ( 0.000000000000000000, 0.2499999999999830136, 0.3749999999999746314, 0.4999999999999662492, 0.7499999999999830136, 1.000000000000000000 ),
 .UNSPECIFIED. ) ;
#14639=ORIENTED_EDGE ( 'NONE', *, *, #23286, .F. ) ;
#14653=CARTESIAN_POINT ( 'NONE',  ( -22.71671780387977790, -14.21943167064913105, 5.548968161578956781 ) ) ;
#14657=CARTESIAN_POINT ( 'NONE',  ( -2.664535259099999568E-14, -26.80000000000000071, 20.00000000000000355 ) ) ;
#14658=ADVANCED_FACE ( 'NONE', ( #10781 ), #6209, .T. ) ;
#14661=CARTESIAN_POINT ( 'NONE',  ( -23.24663841809999809, -14.69162354060000020, 225.0000000000000000 ) ) ;
#14662=CARTESIAN_POINT ( 'NONE',  ( 2.639254916689341979, -27.37824394259287786, 20.00000000000000711 ) ) ;
#14668=DIRECTION ( 'NONE',  ( 1.000000000000000000, 0.000000000000000000, 0.000000000000000000 ) ) ;
#14669=ORIENTED_EDGE ( 'NONE', *, *, #19991, .T. ) ;
#14670=ADVANCED_FACE ( 'NONE', ( #17996 ), #23084, .T. ) ;
#14671=CARTESIAN_POINT ( 'NONE',  ( 28.50000000000000000, -3.490128108379999702E-15, 90.00000000000000000 ) ) ;
#14673=VERTEX_POINT ( 'NONE', #1343 ) ;
#14676=ORIENTED_EDGE ( 'NONE', *, *, #24737, .T. ) ;
#14681=CYLINDRICAL_SURFACE ( 'NONE', #19990, 26.80000000000002203 ) ;
#14684=ORIENTED_EDGE ( 'NONE', *, *, #2189, .F. ) ;
#14685=CIRCLE ( 'NONE', #5122, 4.000000000000001776 ) ;
#14686=CYLINDRICAL_SURFACE ( 'NONE', #7505, 1.099999999999999867 ) ;
#14694=CARTESIAN_POINT ( 'NONE',  ( 26.80000000069999899, -3.281945028320000125E-15, 87.11018146770000214 ) ) ;
#14695=CARTESIAN_POINT ( 'NONE',  ( 23.24667624907482377, -14.69156368041588934, 225.1456731698967246 ) ) ;
#14697=CARTESIAN_POINT ( 'NONE',  ( 22.73383167118559456, -14.19258501486319268, 5.597929191417664541 ) ) ;
#14699=DIRECTION ( 'NONE',  ( 0.9316362575375356503, 0.3633921898465274913, 0.000000000000000000 ) ) ;
#14704=ORIENTED_EDGE ( 'NONE', *, *, #29581, .T. ) ;
#14710=ORIENTED_EDGE ( 'NONE', *, *, #23489, .T. ) ;
#14712=CARTESIAN_POINT ( 'NONE',  ( -27.50000000000000000, 3.367667473009999970E-15, 165.0000000000000000 ) ) ;
#14721=AXIS2_PLACEMENT_3D ( 'NONE', #18751, #9622, #11523 ) ;
#14727=ORIENTED_EDGE ( 'NONE', *, *, #30110, .F. ) ;
#14728=DIRECTION ( 'NONE',  ( 0.000000000000000000, 0.000000000000000000, 1.000000000000000000 ) ) ;
#14729=CARTESIAN_POINT ( 'NONE',  ( 23.73992238019999945, -12.43607998449999918, 225.0000000000000000 ) ) ;
#14737=EDGE_CURVE ( 'NONE', #9526, #20878, #12781, .T. ) ;
#14750=EDGE_LOOP ( 'NONE', ( #18363, #25819, #22712, #21441, #8098, #22070 ) ) ;
#14754=AXIS2_PLACEMENT_3D ( 'NONE', #28473, #6603, #13692 ) ;
#14761=CARTESIAN_POINT ( 'NONE',  ( 27.50000000000000000, -3.367667472999999580E-15, 86.71909809219998522 ) ) ;
#14774=CARTESIAN_POINT ( 'NONE',  ( 0.4946807726542973849, -26.79522487520557661, 224.0068048305045068 ) ) ;
#14775=CARTESIAN_POINT ( 'NONE',  ( -10.06596365874885812, -25.80632433378972124, 40.00000000000000000 ) ) ;
#14790=EDGE_CURVE ( 'NONE', #28212, #20745, #5258, .T. ) ;
#14804=CIRCLE ( 'NONE', #25866, 27.50000000000000000 ) ;
#14806=AXIS2_PLACEMENT_3D ( 'NONE', #15774, #30575, #11063 ) ;
#14813=DIRECTION ( 'NONE',  ( 0.8660254037843290176, 0.5000000000001899592, 1.018673689593249976E-32 ) ) ;
#14822=AXIS2_PLACEMENT_3D ( 'NONE', #30280, #11240, #23372 ) ;
#14833=EDGE_LOOP ( 'NONE', ( #26064, #24461, #30343, #3354 ) ) ;
#14835=CIRCLE ( 'NONE', #23319, 26.79999999889999884 ) ;
#14837=ORIENTED_EDGE ( 'NONE', *, *, #23107, .T. ) ;
#14841=EDGE_CURVE ( 'NONE', #1598, #17245, #21509, .T. ) ;
#14842=CARTESIAN_POINT ( 'NONE',  ( 0.000000000000000000, -17.25771824150000100, 225.0000000000000000 ) ) ;
#14850=ORIENTED_EDGE ( 'NONE', *, *, #11985, .F. ) ;
#14855=CARTESIAN_POINT ( 'NONE',  ( -27.63177371730000331, 3.383804566159999695E-15, 142.6394760449999808 ) ) ;
#14862=FACE_OUTER_BOUND ( 'NONE', #4344, .T. ) ;
#14877=VERTEX_POINT ( 'NONE', #390 ) ;
#14879=CARTESIAN_POINT ( 'NONE',  ( -3.552713678799999608E-15, -3.552713678799999608E-15, 193.6055512750000105 ) ) ;
#14880=ADVANCED_FACE ( 'NONE', ( #23994 ), #27531, .T. ) ;
#14887=ORIENTED_EDGE ( 'NONE', *, *, #677, .T. ) ;
#14893=CARTESIAN_POINT ( 'NONE',  ( 2.131628207279999844E-14, -5.329070518200000398E-15, 86.78285841159998881 ) ) ;
#14908=ORIENTED_EDGE ( 'NONE', *, *, #9712, .T. ) ;
#14927=DIRECTION ( 'NONE',  ( -0.3633921898465274913, 0.9316362575375355393, 0.000000000000000000 ) ) ;
#14930=LINE ( 'NONE', #2656, #19256 ) ;
#14941=ORIENTED_EDGE ( 'NONE', *, *, #26372, .F. ) ;
#14943=AXIS2_PLACEMENT_3D ( 'NONE', #17184, #28830, #26949 ) ;
#14953=CARTESIAN_POINT ( 'NONE',  ( -27.50000000000000000, 3.367667473009999970E-15, 86.71909809219998522 ) ) ;
#14970=CIRCLE ( 'NONE', #1402, 3.200000000000000178 ) ;
#14976=EDGE_CURVE ( 'NONE', #17664, #8508, #3405, .T. ) ;
#14981=EDGE_LOOP ( 'NONE', ( #15241, #10885, #2628, #640 ) ) ;
#14986=ORIENTED_EDGE ( 'NONE', *, *, #10579, .T. ) ;
#14994=AXIS2_PLACEMENT_3D ( 'NONE', #7296, #800, #19980 ) ;
#14997=DIRECTION ( 'NONE',  ( 0.9316362575375356503, 0.3633921898465274913, 0.000000000000000000 ) ) ;
#15004=VECTOR ( 'NONE', #3598, 1000.000000000000000 ) ;
#15010=ORIENTED_EDGE ( 'NONE', *, *, #13033, .T. ) ;
#15013=CARTESIAN_POINT ( 'NONE',  ( 9.897162125334208582, -25.37356426560172196, 191.6604601750000256 ) ) ;
#15018=ORIENTED_EDGE ( 'NONE', *, *, #21062, .T. ) ;
#15019=CARTESIAN_POINT ( 'NONE',  ( 23.92402432539614310, -13.56054118960007493, 6.087706803184607551 ) ) ;
#15020=SURFACE_STYLE_USAGE ( .BOTH. , #8377 ) ;
#15031=LINE ( 'NONE', #24624, #18554 ) ;
#15035=ADVANCED_FACE ( 'NONE', ( #11815 ), #8427, .T. ) ;
#15045=DIRECTION ( 'NONE',  ( 0.000000000000000000, 0.000000000000000000, -1.000000000000000000 ) ) ;
#15052=CARTESIAN_POINT ( 'NONE',  ( -3.931979172340965611, -26.51120696000498356, 20.25730302972669605 ) ) ;
#15062=ORIENTED_EDGE ( 'NONE', *, *, #18153, .T. ) ;
#15071=ORIENTED_EDGE ( 'NONE', *, *, #8085, .T. ) ;
#15081=EDGE_CURVE ( 'NONE', #13864, #25831, #13457, .T. ) ;
#15089=ORIENTED_EDGE ( 'NONE', *, *, #11278, .F. ) ;
#15096=ORIENTED_EDGE ( 'NONE', *, *, #1620, .T. ) ;
#15098=B_SPLINE_CURVE_WITH_KNOTS ( 'NONE', 3,
 ( #1070, #13487, #8762, #23103, #21049, #4052, #1544, #1850, #25928, #15685 ),
 .UNSPECIFIED., .F., .F.,
 ( 4, 2, 2, 2, 4 ),
 ( 0.000000000000000000, 0.2500000000000000000, 0.5000000000000001110, 0.7500000000000001110, 1.000000000000000000 ),
 .UNSPECIFIED. ) ;
#15099=ORIENTED_EDGE ( 'NONE', *, *, #17484, .F. ) ;
#15102=CARTESIAN_POINT ( 'NONE',  ( 18.95046173579999760, -18.95046173579999760, 230.0000000000000000 ) ) ;
#15103=CARTESIAN_POINT ( 'NONE',  ( -26.80000000069999899, 3.281945028329999726E-15, 115.0000000010000036 ) ) ;
#15125=ORIENTED_EDGE ( 'NONE', *, *, #26362, .T. ) ;
#15127=CARTESIAN_POINT ( 'NONE',  ( -3.552713678799999608E-15, -3.552713678799999608E-15, 143.2171415880000040 ) ) ;
#15132=ORIENTED_EDGE ( 'NONE', *, *, #12377, .F. ) ;
#15133=PLANE ( 'NONE',  #10449 ) ;
#15144=CIRCLE ( 'NONE', #15632, 4.000000000000001776 ) ;
#15147=CARTESIAN_POINT ( 'NONE',  ( -20.19076655603532799, -17.71015691556360494, 193.2171415880000040 ) ) ;
#15148=CARTESIAN_POINT ( 'NONE',  ( -0.6812178144568332705, -27.49175526154860805, 5.876143015413799908 ) ) ;
#15149=CARTESIAN_POINT ( 'NONE',  ( 23.36339467975494344, -14.50559736754933837, 225.6749683488453400 ) ) ;
#15151=LINE ( 'NONE', #20334, #8748 ) ;
#15172=CARTESIAN_POINT ( 'NONE',  ( 0.000000000000000000, 0.000000000000000000, 40.00000000000000000 ) ) ;
#15174=EDGE_CURVE ( 'NONE', #4659, #11492, #19995, .T. ) ;
#15177=CARTESIAN_POINT ( 'NONE',  ( -26.84464183080000055, 3.287411895199999866E-15, 42.56249624490000372 ) ) ;
#15193=DIRECTION ( 'NONE',  ( -1.000000000000000000, 1.224606353819999829E-16, 0.000000000000000000 ) ) ;
#15195=CARTESIAN_POINT ( 'NONE',  ( -4.679341198149895575, -26.38945575071663896, 20.49029498623629664 ) ) ;
#15203=CIRCLE ( 'NONE', #13707, 26.80000000000000071 ) ;
#15226=CARTESIAN_POINT ( 'NONE',  ( 26.80000000000001492, -1.754055898254314183, 86.78285841095834030 ) ) ;
#15230=CARTESIAN_POINT ( 'NONE',  ( 7.121574564636415694, -25.83919502053028339, 208.0635107809515318 ) ) ;
#15234=ORIENTED_EDGE ( 'NONE', *, *, #22900, .F. ) ;
#15241=ORIENTED_EDGE ( 'NONE', *, *, #30426, .F. ) ;
#15250=ADVANCED_FACE ( 'NONE', ( #27058, #29256 ), #2832, .F. ) ;
#15256=CARTESIAN_POINT ( 'NONE',  ( -27.76135144249999698, 3.399672736719999759E-15, 42.33858589270000294 ) ) ;
#15281=CARTESIAN_POINT ( 'NONE',  ( -0.5612696204402340960, -26.79446732153163424, 4.042548093418004029 ) ) ;
#15285=VERTEX_POINT ( 'NONE', #3133 ) ;
#15286=DIRECTION ( 'NONE',  ( 0.000000000000000000, 0.000000000000000000, -1.000000000000000000 ) ) ;
#15295=CIRCLE ( 'NONE', #29839, 27.23548387100000312 ) ;
#15298=DIRECTION ( 'NONE',  ( 1.000000000000000000, 0.000000000000000000, 0.000000000000000000 ) ) ;
#15300=VERTEX_POINT ( 'NONE', #22185 ) ;
#15303=DIRECTION ( 'NONE',  ( 0.3633921898465289901, 0.9316362575375348731, 1.301042606982604374E-14 ) ) ;
#15305=STYLED_ITEM ( 'NONE', ( #24768 ), #20057 ) ;
#15309=CARTESIAN_POINT ( 'NONE',  ( -24.50000001620000134, 3.000285568850000245E-15, 189.9999999960000139 ) ) ;
#15312=CARTESIAN_POINT ( 'NONE',  ( -23.20948082139999968, -13.40000000000000036, 3.900000000369999942 ) ) ;
#15313=VECTOR ( 'NONE', #10365, 1000.000000000000000 ) ;
#15314=ORIENTED_EDGE ( 'NONE', *, *, #4217, .F. ) ;
#15317=AXIS2_PLACEMENT_3D ( 'NONE', #26850, #16937, #2169 ) ;
#15328=CIRCLE ( 'NONE', #10814, 26.80000000000000071 ) ;
#15331=CARTESIAN_POINT ( 'NONE',  ( 0.000000000000000000, 0.000000000000000000, 115.0000000000000000 ) ) ;
#15332=B_SPLINE_CURVE_WITH_KNOTS ( 'NONE', 3,
 ( #22238, #14695, #695, #10282, #15149, #24750, #3186, #22397, #842, #10434 ),
 .UNSPECIFIED., .F., .F.,
 ( 4, 2, 2, 2, 4 ),
 ( 0.000000000000000000, 0.2500000000000000000, 0.5000000000000000000, 0.7500000000000000000, 1.000000000000000000 ),
 .UNSPECIFIED. ) ;
#15335=CARTESIAN_POINT ( 'NONE',  ( 11.08346179031908818, -28.41490585489483323, 43.60555127550001231 ) ) ;
#15339=CARTESIAN_POINT ( 'NONE',  ( 0.6805609921852766586, -26.79155681362076180, 5.876648811199404854 ) ) ;
#15340=CARTESIAN_POINT ( 'NONE',  ( -26.93395387809999875, 3.298349105260000080E-15, 92.24324102360000666 ) ) ;
#15346=CARTESIAN_POINT ( 'NONE',  ( -23.36339468011815157, -14.50559736696343727, 4.325031650548394779 ) ) ;
#15353=DIRECTION ( 'NONE',  ( 0.000000000000000000, 0.000000000000000000, 1.000000000000000000 ) ) ;
#15355=CARTESIAN_POINT ( 'NONE',  ( -7.662090775718862545, -25.68204763724676454, 22.48967911107480333 ) ) ;
#15361=CARTESIAN_POINT ( 'NONE',  ( -9.993285220779425160, -25.61999708228226069, 115.0000000000000000 ) ) ;
#15368=ADVANCED_FACE ( 'NONE', ( #1648 ), #28534, .F. ) ;
#15373=CARTESIAN_POINT ( 'NONE',  ( -14.94562240850000023, -8.628859120750000500, 225.0000000000000000 ) ) ;
#15379=CARTESIAN_POINT ( 'NONE',  ( 23.73450314244648496, -12.44732035365262313, 4.781948426524514240 ) ) ;
#15381=FACE_OUTER_BOUND ( 'NONE', #19266, .T. ) ;
#15391=EDGE_LOOP ( 'NONE', ( #5337, #15314, #17743, #9837 ) ) ;
#15393=ORIENTED_EDGE ( 'NONE', *, *, #8259, .T. ) ;
#15396=ORIENTED_EDGE ( 'NONE', *, *, #24409, .F. ) ;
#15401=ADVANCED_FACE ( 'NONE', ( #12970 ), #13436, .T. ) ;
#15407=ADVANCED_FACE ( 'NONE', ( #30278 ), #1333, .F. ) ;
#15416=DIRECTION ( 'NONE',  ( 0.9316362575375356503, 0.3633921898465274913, 0.000000000000000000 ) ) ;
#15424=ORIENTED_EDGE ( 'NONE', *, *, #619, .F. ) ;
#15434=EDGE_LOOP ( 'NONE', ( #15099, #10755, #11211, #76 ) ) ;
#15448=CARTESIAN_POINT ( 'NONE',  ( 9.590600648852312560, -25.77356060526425452, 204.6037742833236166 ) ) ;
#15461=EDGE_CURVE ( 'NONE', #7351, #30811, #28164, .T. ) ;
#15470=CIRCLE ( 'NONE', #18483, 4.000000000000001776 ) ;
#15494=CARTESIAN_POINT ( 'NONE',  ( 11.08346179031908640, -28.41490585489483678, 36.39444872449999480 ) ) ;
#15497=CARTESIAN_POINT ( 'NONE',  ( -8.727399452413349579, -25.34090985533206108, 206.0457211097556751 ) ) ;
#15503=CARTESIAN_POINT ( 'NONE',  ( -9.738910687886859208, -24.96785170200599069, 27.46683069121352005 ) ) ;
#15508=LINE ( 'NONE', #1359, #9936 ) ;
#15512=ORIENTED_EDGE ( 'NONE', *, *, #10047, .F. ) ;
#15513=TOROIDAL_SURFACE ( 'NONE', #6998, 29.80000000000000071, 3.000000000000000000 ) ;
#15515=ORIENTED_EDGE ( 'NONE', *, *, #80, .F. ) ;
#15516=ADVANCED_FACE ( 'NONE', ( #7445, #25010 ), #12012, .T. ) ;
#15517=CARTESIAN_POINT ( 'NONE',  ( 0.000000000000000000, 0.000000000000000000, 88.33953982530000815 ) ) ;
#15521=PLANE ( 'NONE',  #28009 ) ;
#15522=LINE ( 'NONE', #12861, #13511 ) ;
#15527=TOROIDAL_SURFACE ( 'NONE', #29099, 30.50000000000000000, 3.000000000000000000 ) ;
#15529=CARTESIAN_POINT ( 'NONE',  ( 23.31845629885299331, -13.20933888571149595, 3.912379060708174983 ) ) ;
#15536=CARTESIAN_POINT ( 'NONE',  ( 1.841797396446240631, -26.73663745407121795, 210.0000000000000284 ) ) ;
#15539=CARTESIAN_POINT ( 'NONE',  ( 8.160452367545499186, -25.52912514472581407, 23.07342428570553494 ) ) ;
#15551=CARTESIAN_POINT ( 'NONE',  ( 11.08346179031908285, -28.41490585489482967, 86.39444872449999480 ) ) ;
#15552=CARTESIAN_POINT ( 'NONE',  ( -27.50000000000000000, 3.367667473009999970E-15, 86.39444872359999295 ) ) ;
#15558=VERTEX_POINT ( 'NONE', #29730 ) ;
#15559=EDGE_CURVE ( 'NONE', #14877, #16822, #10991, .T. ) ;
#15562=CARTESIAN_POINT ( 'NONE',  ( -27.23548387100000312, 8.881784196999999612E-15, 41.66046017469999896 ) ) ;
#15571=ORIENTED_EDGE ( 'NONE', *, *, #3470, .F. ) ;
#15572=EDGE_CURVE ( 'NONE', #24391, #8738, #17041, .T. ) ;
#15576=LINE ( 'NONE', #1276, #23819 ) ;
#15582=CARTESIAN_POINT ( 'NONE',  ( -9.219833965033632950, -25.90918750570071438, 24.42156808705805560 ) ) ;
#15599=CARTESIAN_POINT ( 'NONE',  ( 7.365079183348029801, -26.49619795852259685, 208.0568234296057426 ) ) ;
#15609=CARTESIAN_POINT ( 'NONE',  ( -23.24667624907481667, -14.69156368041588934, 224.8543268298566602 ) ) ;
#15611=AXIS2_PLACEMENT_3D ( 'NONE', #20806, #30876, #23174 ) ;
#15615=ORIENTED_EDGE ( 'NONE', *, *, #4671, .F. ) ;
#15620=VERTEX_POINT ( 'NONE', #13047 ) ;
#15621=CARTESIAN_POINT ( 'NONE',  ( -3.552713678799999608E-15, 0.000000000000000000, 37.93968498539999956 ) ) ;
#15623=ORIENTED_EDGE ( 'NONE', *, *, #17978, .T. ) ;
#15624=ORIENTED_EDGE ( 'NONE', *, *, #20220, .T. ) ;
#15626=DIRECTION ( 'NONE',  ( 0.000000000000000000, 0.000000000000000000, 1.000000000000000000 ) ) ;
#15628=DIRECTION ( 'NONE',  ( 0.000000000000000000, 0.000000000000000000, 1.000000000000000000 ) ) ;
#15632=AXIS2_PLACEMENT_3D ( 'NONE', #7529, #24371, #12402 ) ;
#15636=DIRECTION ( 'NONE',  ( 0.5000000000001894040, 0.8660254037843291286, 0.000000000000000000 ) ) ;
#15641=EDGE_CURVE ( 'NONE', #4159, #27653, #16347, .T. ) ;
#15647=LINE ( 'NONE', #6370, #20195 ) ;
#15652=ORIENTED_EDGE ( 'NONE', *, *, #14351, .F. ) ;
#15658=CIRCLE ( 'NONE', #12646, 3.200000000000002398 ) ;
#15663=DIRECTION ( 'NONE',  ( -1.000000000000000000, 5.665498452320000818E-16, 0.000000000000000000 ) ) ;
#15667=ORIENTED_EDGE ( 'NONE', *, *, #20592, .T. ) ;
#15680=DIRECTION ( 'NONE',  ( 0.9316362575375356503, 0.3633921898465274913, 0.000000000000000000 ) ) ;
#15685=CARTESIAN_POINT ( 'NONE',  ( -2.947640775130000104E-14, -27.50000000000000000, 226.0999999999999943 ) ) ;
#15691=CIRCLE ( 'NONE', #17204, 3.199999983039998774 ) ;
#15698=VERTEX_POINT ( 'NONE', #30038 ) ;
#15704=LINE ( 'NONE', #3436, #12455 ) ;
#15707=CYLINDRICAL_SURFACE ( 'NONE', #11437, 27.50000000000000000 ) ;
#15709=CARTESIAN_POINT ( 'NONE',  ( -0.6483608311672878211, -27.49254329982247214, 4.090437960807658868 ) ) ;
#15710=DIRECTION ( 'NONE',  ( -0.3090169943750401549, -0.9510565162951233331, 0.000000000000000000 ) ) ;
#15717=CYLINDRICAL_SURFACE ( 'NONE', #12661, 26.80000000000002203 ) ;
#15723=CARTESIAN_POINT ( 'NONE',  ( 22.74701237783497731, -14.17144074696374290, 225.6389823648914330 ) ) ;
#15728=AXIS2_PLACEMENT_3D ( 'NONE', #17319, #22363, #10398 ) ;
#15731=CARTESIAN_POINT ( 'NONE',  ( -1.421085471519999843E-14, -3.552713678799999608E-15, 137.9396849850000137 ) ) ;
#15734=CIRCLE ( 'NONE', #14250, 27.50000000000000000 ) ;
#15740=CARTESIAN_POINT ( 'NONE',  ( 0.000000000000000000, 0.000000000000000000, 186.3944487260000074 ) ) ;
#15742=ADVANCED_FACE ( 'NONE', ( #3768 ), #4238, .F. ) ;
#15745=ORIENTED_EDGE ( 'NONE', *, *, #13554, .T. ) ;
#15747=ORIENTED_EDGE ( 'NONE', *, *, #23615, .T. ) ;
#15752=FACE_OUTER_BOUND ( 'NONE', #25515, .T. ) ;
#15762=DIRECTION ( 'NONE',  ( 0.000000000000000000, 0.000000000000000000, 1.000000000000000000 ) ) ;
#15771=CARTESIAN_POINT ( 'NONE',  ( 23.48807013355484585, -14.30280389817958842, 224.0869147245778947 ) ) ;
#15774=CARTESIAN_POINT ( 'NONE',  ( 0.000000000000000000, 0.000000000000000000, 140.0000000000000000 ) ) ;
#15775=VERTEX_POINT ( 'NONE', #25651 ) ;
#15776=CARTESIAN_POINT ( 'NONE',  ( -18.95046173579999760, -18.95046173579999760, 86.78285841159998881 ) ) ;
#15780=EDGE_CURVE ( 'NONE', #11492, #3101, #23566, .T. ) ;
#15782=CIRCLE ( 'NONE', #27836, 27.23548387080000310 ) ;
#15783=EDGE_LOOP ( 'NONE', ( #19705, #29747, #13660, #11569, #17140, #26552 ) ) ;
#15789=CIRCLE ( 'NONE', #23849, 4.000000004070001225 ) ;
#15792=CARTESIAN_POINT ( 'NONE',  ( 23.24663841807412723, -14.69162354064478571, 4.903540289168272892 ) ) ;
#15797=CARTESIAN_POINT ( 'NONE',  ( 0.000000000000000000, 3.552713678799999608E-15, 43.60555127550000520 ) ) ;
#15802=CARTESIAN_POINT ( 'NONE',  ( -1.421085471519999843E-14, -1.421085471519999843E-14, 36.39444872449999480 ) ) ;
#15804=CARTESIAN_POINT ( 'NONE',  ( 26.79999999930000243, -1.760380630484417619, 0.000000000000000000 ) ) ;
#15812=CIRCLE ( 'NONE', #27375, 27.50000000000000000 ) ;
#15815=CIRCLE ( 'NONE', #20829, 27.92857142840000151 ) ;
#15821=CARTESIAN_POINT ( 'NONE',  ( 27.50000000000000000, -3.367667472999999580E-15, 143.6055512739999926 ) ) ;
#15824=DIRECTION ( 'NONE',  ( 0.3633921898465272138, -0.9316362575375356503, 0.000000000000000000 ) ) ;
#15825=APPLICATION_CONTEXT ( 'automotive_design' ) ;
#15835=VECTOR ( 'NONE', #23299, 1000.000000000000114 ) ;
#15839=ORIENTED_EDGE ( 'NONE', *, *, #11985, .T. ) ;
#15852=DIRECTION ( 'NONE',  ( -1.224606353819999829E-16, -1.000000000000000000, 0.000000000000000000 ) ) ;
#15864=LINE ( 'NONE', #25631, #30839 ) ;
#15870=ORIENTED_EDGE ( 'NONE', *, *, #11600, .T. ) ;
#15875=ORIENTED_EDGE ( 'NONE', *, *, #21123, .F. ) ;
#15880=CYLINDRICAL_SURFACE ( 'NONE', #8399, 7.999999999999998224 ) ;
#15881=DIRECTION ( 'NONE',  ( 0.3633921898465291567, 0.9316362575375348731, 0.000000000000000000 ) ) ;
#15893=EDGE_CURVE ( 'NONE', #7025, #2249, #27047, .T. ) ;
#15899=VERTEX_POINT ( 'NONE', #11784 ) ;
#15900=CARTESIAN_POINT ( 'NONE',  ( -22.74701237787062169, -14.17144074690075328, 224.3610176349945391 ) ) ;
#15906=ORIENTED_EDGE ( 'NONE', *, *, #9079, .T. ) ;
#15911=CARTESIAN_POINT ( 'NONE',  ( 0.000000000000000000, 3.552713678799999608E-15, 193.2171415880000040 ) ) ;
#15921=CARTESIAN_POINT ( 'NONE',  ( 24.50000001620000134, -3.000285568839999855E-15, 190.0000000039999861 ) ) ;
#15925=CARTESIAN_POINT ( 'NONE',  ( 9.897162125400441823, -25.37356426577149193, 38.33953982530000104 ) ) ;
#15926=CARTESIAN_POINT ( 'NONE',  ( -1.100000000000000089, -26.77741585740000119, 5.000000000000000000 ) ) ;
#15938=CARTESIAN_POINT ( 'NONE',  ( -26.80000000000000071, 1.776356839399999804E-15, -2.842170943039999687E-14 ) ) ;
#15939=CARTESIAN_POINT ( 'NONE',  ( 26.80000000000001492, -1.754055898254314183, 186.7828584119999960 ) ) ;
#15944=CARTESIAN_POINT ( 'NONE',  ( -20.19076655603533510, -17.71015691556365468, 186.7828584120833284 ) ) ;
#15947=VERTEX_POINT ( 'NONE', #1375 ) ;
#15948=CARTESIAN_POINT ( 'NONE',  ( -9.738910687886855655, -24.96785170200598714, 115.0000000000000000 ) ) ;
#15953=AXIS2_PLACEMENT_3D ( 'NONE', #25363, #28022, #6467 ) ;
#15961=CARTESIAN_POINT ( 'NONE',  ( 20.19076655603537418, -17.71015691556361205, 136.7828584120000244 ) ) ;
#15966=CARTESIAN_POINT ( 'NONE',  ( 8.903108651239925564, -22.82508830966962421, 190.0000000000000000 ) ) ;
#15967=EDGE_CURVE ( 'NONE', #21131, #29406, #22767, .T. ) ;
#15969=CARTESIAN_POINT ( 'NONE',  ( -23.47117976039525189, -14.33053685688857826, 4.119508997195603150 ) ) ;
#15971=CARTESIAN_POINT ( 'NONE',  ( 23.73992238019999945, -12.43607998449999918, 225.0000000000000000 ) ) ;
#15972=CARTESIAN_POINT ( 'NONE',  ( 8.903108651239925564, -22.82508830966962421, 40.00000000000000000 ) ) ;
#15986=DIRECTION ( 'NONE',  ( 1.000000000000000000, -1.224606353819999829E-16, 0.000000000000000000 ) ) ;
#15995=CIRCLE ( 'NONE', #13473, 4.000000004070001225 ) ;
#16003=CARTESIAN_POINT ( 'NONE',  ( -27.50000000000000000, 3.367667473009999970E-15, 115.0000000000000000 ) ) ;
#16006=CARTESIAN_POINT ( 'NONE',  ( 23.25801811797813556, -13.31593093537183492, 3.899999999996501820 ) ) ;
#16007=CARTESIAN_POINT ( 'NONE',  ( 0.000000000000000000, 0.000000000000000000, 90.00000000000000000 ) ) ;
#16011=EDGE_CURVE ( 'NONE', #30396, #30479, #21039, .T. ) ;
#16031=ADVANCED_FACE ( 'NONE', ( #18823 ), #11489, .T. ) ;
#16034=DIRECTION ( 'NONE',  ( 0.000000000000000000, 0.000000000000000000, 1.000000000000000000 ) ) ;
#16041=EDGE_CURVE ( 'NONE', #16579, #17696, #30790, .T. ) ;
#16044=CARTESIAN_POINT ( 'NONE',  ( -0.4946807661028205794, -26.79522487538596565, 5.993195172251796876 ) ) ;
#16057=CARTESIAN_POINT ( 'NONE',  ( 1.100000000000000089, -26.77741585740000119, 5.000000000000000000 ) ) ;
#16065=EDGE_LOOP ( 'NONE', ( #9161, #28521, #28205, #20890 ) ) ;
#16067=ORIENTED_EDGE ( 'NONE', *, *, #17683, .T. ) ;
#16072=DIRECTION ( 'NONE',  ( 0.3633921898465276024, -0.9316362575375355393, 0.000000000000000000 ) ) ;
#16075=ORIENTED_EDGE ( 'NONE', *, *, #24613, .F. ) ;
#16078=CARTESIAN_POINT ( 'NONE',  ( -2.639254916689323327, -27.37824394259287430, 210.0000000000000284 ) ) ;
#16079=EDGE_CURVE ( 'NONE', #19872, #18447, #28550, .T. ) ;
#16086=DIRECTION ( 'NONE',  ( -1.000000000000000000, 5.665498452320000818E-16, 0.000000000000000000 ) ) ;
#16092=CARTESIAN_POINT ( 'NONE',  ( -24.76521256262105553, -10.24325429074770533, 93.21714158839978381 ) ) ;
#16099=ORIENTED_EDGE ( 'NONE', *, *, #27103, .F. ) ;
#16112=ORIENTED_EDGE ( 'NONE', *, *, #14060, .T. ) ;
#16122=CARTESIAN_POINT ( 'NONE',  ( 9.739400760072928875, -25.71769950840797847, 25.91465618243121938 ) ) ;
#16123=CARTESIAN_POINT ( 'NONE',  ( -23.53263993762945461, -14.22965940626688131, 4.040453395607338294 ) ) ;
#16134=ORIENTED_EDGE ( 'NONE', *, *, #20770, .F. ) ;
#16137=ORIENTED_EDGE ( 'NONE', *, *, #886, .T. ) ;
#16141=VERTEX_POINT ( 'NONE', #4660 ) ;
#16149=CARTESIAN_POINT ( 'NONE',  ( -26.80000000069999899, 3.281945028329999726E-15, 230.0000000000000000 ) ) ;
#16152=ADVANCED_FACE ( 'NONE', ( #23874 ), #23042, .T. ) ;
#16160=CARTESIAN_POINT ( 'NONE',  ( -8.903108651239966420, -22.82508830966961000, 90.00000000000000000 ) ) ;
#16168=ORIENTED_EDGE ( 'NONE', *, *, #14195, .T. ) ;
#16193=ADVANCED_FACE ( 'NONE', ( #24480 ), #26246, .T. ) ;
#16198=CARTESIAN_POINT ( 'NONE',  ( -15.49562240950000103, -7.676231176589999983, 225.0000000000000000 ) ) ;
#16201=CARTESIAN_POINT ( 'NONE',  ( -23.68823177905599309, -12.53428999867805160, 4.513393846701676537 ) ) ;
#16204=VERTEX_POINT ( 'NONE', #12510 ) ;
#16212=VERTEX_POINT ( 'NONE', #19759 ) ;
#16214=EDGE_CURVE ( 'NONE', #1526, #19354, #2629, .T. ) ;
#16216=ORIENTED_EDGE ( 'NONE', *, *, #11149, .F. ) ;
#16219=AXIS2_PLACEMENT_3D ( 'NONE', #18441, #13091, #29933 ) ;
#16221=DIRECTION ( 'NONE',  ( 0.3090169943750400994, -0.9510565162951234441, 0.000000000000000000 ) ) ;
#16230=FACE_OUTER_BOUND ( 'NONE', #15391, .T. ) ;
#16237=CARTESIAN_POINT ( 'NONE',  ( 0.000000000000000000, 0.000000000000000000, 140.0000000000000000 ) ) ;
#16243=LINE ( 'NONE', #18606, #7737 ) ;
#16246=CARTESIAN_POINT ( 'NONE',  ( 18.95046173579999760, -18.95046173579999760, 136.7828584120000244 ) ) ;
#16247=FACE_OUTER_BOUND ( 'NONE', #1088, .T. ) ;
#16253=DIRECTION ( 'NONE',  ( -1.000000000000000000, 5.665498452320000818E-16, 0.000000000000000000 ) ) ;
#16262=CARTESIAN_POINT ( 'NONE',  ( -23.65805500392816896, -12.59178324492199508, 5.597929191016143946 ) ) ;
#16263=ORIENTED_EDGE ( 'NONE', *, *, #14582, .F. ) ;
#16267=CARTESIAN_POINT ( 'NONE',  ( 20.19452343149548668, -17.70639519314953958, 0.000000000000000000 ) ) ;
#16273=CARTESIAN_POINT ( 'NONE',  ( 4.696583076644019528, -27.09716880376584314, 20.40570884047772893 ) ) ;
#16274=CARTESIAN_POINT ( 'NONE',  ( 23.06380069550898781, -13.64989377374051216, 3.928509483758267251 ) ) ;
#16275=LINE ( 'NONE', #4798, #18205 ) ;
#16283=VECTOR ( 'NONE', #9230, 1000.000000000000000 ) ;
#16284=EDGE_CURVE ( 'NONE', #29399, #9436, #20688, .T. ) ;
#16294=ORIENTED_EDGE ( 'NONE', *, *, #12709, .T. ) ;
#16295=FACE_OUTER_BOUND ( 'NONE', #24121, .T. ) ;
#16300=AXIS2_PLACEMENT_3D ( 'NONE', #4803, #24000, #21785 ) ;
#16301=AXIS2_PLACEMENT_3D ( 'NONE', #30261, #18292, #30889 ) ;
#16302=CARTESIAN_POINT ( 'NONE',  ( 27.76135144259999876, -3.399672736709999763E-15, 42.33858589270000294 ) ) ;
#16304=UNCERTAINTY_MEASURE_WITH_UNIT (LENGTH_MEASURE( 1.000000000000000082E-05 ), #1680, 'distance_accuracy_value', 'NONE');
#16305=CIRCLE ( 'NONE', #22843, 27.50000000000000000 ) ;
#16308=DIRECTION ( 'NONE',  ( -1.000000000000000000, 5.665498452320000818E-16, 0.000000000000000000 ) ) ;
#16309=EDGE_LOOP ( 'NONE', ( #23302, #29861, #16134, #7161 ) ) ;
#16336=CIRCLE ( 'NONE', #11801, 3.000000000000001332 ) ;
#16339=CARTESIAN_POINT ( 'NONE',  ( 0.000000000000000000, 0.000000000000000000, 115.0000000000000000 ) ) ;
#16340=CARTESIAN_POINT ( 'NONE',  ( 23.73992238019999945, -12.43607998449999918, 5.000000000000000000 ) ) ;
#16343=DIRECTION ( 'NONE',  ( -0.3090169943750401549, -0.9510565162951233331, 0.000000000000000000 ) ) ;
#16347=LINE ( 'NONE', #13678, #18510 ) ;
#16371=ORIENTED_EDGE ( 'NONE', *, *, #25781, .T. ) ;
#16372=DIRECTION ( 'NONE',  ( 1.000000000000000000, 0.000000000000000000, 0.000000000000000000 ) ) ;
#16393=DIRECTION ( 'NONE',  ( 0.000000000000000000, 0.000000000000000000, -1.000000000000000000 ) ) ;
#16402=DIRECTION ( 'NONE',  ( 0.000000000000000000, 0.000000000000000000, 1.000000000000000000 ) ) ;
#16404=VERTEX_POINT ( 'NONE', #28544 ) ;
#16408=ORIENTED_EDGE ( 'NONE', *, *, #14020, .T. ) ;
#16423=CARTESIAN_POINT ( 'NONE',  ( -22.71519155902493381, -14.22192772757401258, 225.5575347055555255 ) ) ;
#16428=VERTEX_POINT ( 'NONE', #23377 ) ;
#16433=EDGE_CURVE ( 'NONE', #2249, #18378, #26189, .T. ) ;
#16434=DIRECTION ( 'NONE',  ( -0.9316362575375349842, 0.3633921898465292122, -0.000000000000000000 ) ) ;
#16437=DIRECTION ( 'NONE',  ( -1.000000000000000000, 5.665498452320000818E-16, 0.000000000000000000 ) ) ;
#16439=EDGE_CURVE ( 'NONE', #28570, #19740, #19712, .T. ) ;
#16447=ORIENTED_EDGE ( 'NONE', *, *, #2934, .F. ) ;
#16448=CARTESIAN_POINT ( 'NONE',  ( 27.92857142909999979, -3.420150602509999660E-15, 37.93968498519999599 ) ) ;
#16455=CARTESIAN_POINT ( 'NONE',  ( 0.2860395612620135197, -27.49884598709296668, 223.9280906791276493 ) ) ;
#16456=CARTESIAN_POINT ( 'NONE',  ( 27.23548387180000319, -3.335274659869999873E-15, 41.66046017409999536 ) ) ;
#16461=VERTEX_POINT ( 'NONE', #1814 ) ;
#16462=CARTESIAN_POINT ( 'NONE',  ( 24.49999999589999788, -3.000285566359999846E-15, 90.00000000000000000 ) ) ;
#16475=VERTEX_POINT ( 'NONE', #28698 ) ;
#16476=CIRCLE ( 'NONE', #10957, 26.80000000000000071 ) ;
#16482=CIRCLE ( 'NONE', #16977, 26.80000000000000071 ) ;
#16492=CARTESIAN_POINT ( 'NONE',  ( -10.82908725742657730, -27.76276047461854901, 186.7828584120000244 ) ) ;
#16499=CIRCLE ( 'NONE', #12991, 4.000000004070001225 ) ;
#16507=DIRECTION ( 'NONE',  ( -1.000000000000000000, 0.000000000000000000, 0.000000000000000000 ) ) ;
#16511=CARTESIAN_POINT ( 'NONE',  ( 0.000000000000000000, -17.25771824150000100, 5.000000000000000000 ) ) ;
#16522=EDGE_LOOP ( 'NONE', ( #10352, #27428, #28105, #27690, #28842 ) ) ;
#16523=VECTOR ( 'NONE', #13756, 1000.000000000000000 ) ;
#16528=DIRECTION ( 'NONE',  ( 1.224606353819999829E-16, 1.000000000000000000, 0.000000000000000000 ) ) ;
#16533=DIRECTION ( 'NONE',  ( 0.3633921898465272138, -0.9316362575375356503, 1.850371707708593498E-14 ) ) ;
#16538=B_SPLINE_CURVE_WITH_KNOTS ( 'NONE', 3,
 ( #16057, #30385, #13381, #11494, #8811, #21097, #9120, #1435, #20619, #11341, #27693, #30217, #8649, #6608 ),
 .UNSPECIFIED., .F., .F.,
 ( 4, 2, 2, 2, 2, 2, 4 ),
 ( 0.000000000000000000, 0.2500000000000027756, 0.3750000000000041078, 0.4375000000000041633, 0.5000000000000042188, 0.7500000000000022204, 1.000000000000000000 ),
 .UNSPECIFIED. ) ;
#16541=CARTESIAN_POINT ( 'NONE',  ( -23.20948082139999968, -13.40000000000000036, 223.8999999999999773 ) ) ;
#16565=EDGE_CURVE ( 'NONE', #16141, #10785, #546, .T. ) ;
#16568=EDGE_LOOP ( 'NONE', ( #8492, #12347, #7500, #12884, #18207, #14941, #17138, #10291, #3499, #2565 ) ) ;
#16573=ORIENTED_EDGE ( 'NONE', *, *, #4504, .F. ) ;
#16578=FACE_OUTER_BOUND ( 'NONE', #8816, .T. ) ;
#16579=VERTEX_POINT ( 'NONE', #5242 ) ;
#16584=CARTESIAN_POINT ( 'NONE',  ( 1.100000000000000089, -26.77741585740000119, 225.0000000000000000 ) ) ;
#16587=ORIENTED_EDGE ( 'NONE', *, *, #26796, .F. ) ;
#16593=B_SPLINE_CURVE_WITH_KNOTS ( 'NONE', 5,
 ( #8904, #4349, #9061, #1529, #11586, #13634 ),
 .UNSPECIFIED., .F., .F.,
 ( 6, 6 ),
 ( -2.319814964989999950, 0.000000000000000000 ),
 .UNSPECIFIED. ) ;
#16597=LINE ( 'NONE', #9357, #9427 ) ;
#16600=AXIS2_PLACEMENT_3D ( 'NONE', #13223, #20912, #30510 ) ;
#16601=ORIENTED_EDGE ( 'NONE', *, *, #14195, .F. ) ;
#16607=CARTESIAN_POINT ( 'NONE',  ( -7.105427357599999217E-15, 0.000000000000000000, 86.78285841159998881 ) ) ;
#16611=CARTESIAN_POINT ( 'NONE',  ( 10.82908725742653999, -27.76276047461857033, 86.78285841159998881 ) ) ;
#16623=DIRECTION ( 'NONE',  ( 0.000000000000000000, 0.000000000000000000, 1.000000000000000000 ) ) ;
#16627=DIRECTION ( 'NONE',  ( 0.000000000000000000, 0.000000000000000000, 1.000000000000000000 ) ) ;
#16635=EDGE_CURVE ( 'NONE', #20468, #25887, #15691, .T. ) ;
#16638=EDGE_CURVE ( 'NONE', #5682, #5141, #15332, .T. ) ;
#16639=ORIENTED_EDGE ( 'NONE', *, *, #19706, .T. ) ;
#16644=DIRECTION ( 'NONE',  ( 1.000000000000000000, 0.000000000000000000, 0.000000000000000000 ) ) ;
#16654=CARTESIAN_POINT ( 'NONE',  ( 24.49999999589999788, -3.000285566359999846E-15, 40.00000000000000000 ) ) ;
#16667=TOROIDAL_SURFACE ( 'NONE', #14167, 29.80000000000000071, 3.000000000000000000 ) ;
#16669=AXIS2_PLACEMENT_3D ( 'NONE', #7810, #24193, #26702 ) ;
#16670=DIRECTION ( 'NONE',  ( 0.3633921898465291567, 0.9316362575375349842, 0.000000000000000000 ) ) ;
#16672=ORIENTED_EDGE ( 'NONE', *, *, #4497, .F. ) ;
#16677=ORIENTED_EDGE ( 'NONE', *, *, #9606, .F. ) ;
#16685=AXIS2_PLACEMENT_3D ( 'NONE', #12829, #14728, #3066 ) ;
#16690=CARTESIAN_POINT ( 'NONE',  ( 23.28210887557342446, -13.27420452015669738, 226.1000000000000227 ) ) ;
#16694=EDGE_CURVE ( 'NONE', #16896, #16475, #13831, .T. ) ;
#16704=AXIS2_PLACEMENT_3D ( 'NONE', #23723, #30367, #20761 ) ;
#16715=CARTESIAN_POINT ( 'NONE',  ( 18.95046173579999760, -18.95046173579999760, -2.842170943039999687E-14 ) ) ;
#16723=DIRECTION ( 'NONE',  ( 0.3633921898465272138, -0.9316362575375356503, -2.775557561562890089E-14 ) ) ;
#16728=CARTESIAN_POINT ( 'NONE',  ( 22.63992238019999803, -14.34133587289999845, 5.000000000000000000 ) ) ;
#16735=PLANE ( 'NONE',  #16300 ) ;
#16737=B_SPLINE_CURVE_WITH_KNOTS ( 'NONE', 3,
 ( #16728, #12021, #14547, #29156, #231, #14697, #17196, #19105, #9818, #28845, #16891, #19415, #31066, #26496 ),
 .UNSPECIFIED., .F., .F.,
 ( 4, 2, 2, 2, 2, 2, 4 ),
 ( 0.000000000000000000, 0.2500000000000003886, 0.3750000000000010547, 0.4375000000000007772, 0.5000000000000005551, 0.7500000000000002220, 1.000000000000000000 ),
 .UNSPECIFIED. ) ;
#16742=EDGE_CURVE ( 'NONE', #14204, #22999, #6689, .T. ) ;
#16747=AXIS2_PLACEMENT_3D ( 'NONE', #5985, #13537, #18088 ) ;
#16759=CARTESIAN_POINT ( 'NONE',  ( 1.099929244070992018, -27.47799402545701852, 224.8543268301346814 ) ) ;
#16762=AXIS2_PLACEMENT_3D ( 'NONE', #3983, #13737, #4302 ) ;
#16764=ORIENTED_EDGE ( 'NONE', *, *, #28591, .T. ) ;
#16767=AXIS2_PLACEMENT_3D ( 'NONE', #3420, #17433, #22477 ) ;
#16774=EDGE_CURVE ( 'NONE', #28706, #18380, #10489, .T. ) ;
#16784=DIRECTION ( 'NONE',  ( -0.9316362575375349842, 0.3633921898465292122, -0.000000000000000000 ) ) ;
#16793=AXIS2_PLACEMENT_3D ( 'NONE', #8913, #15680, #25290 ) ;
#16795=CYLINDRICAL_SURFACE ( 'NONE', #9579, 8.000000000000000000 ) ;
#16810=ADVANCED_FACE ( 'NONE', ( #19534 ), #7563, .F. ) ;
#16812=DIRECTION ( 'NONE',  ( -1.000000000000000000, 5.665498452320000818E-16, 0.000000000000000000 ) ) ;
#16822=VERTEX_POINT ( 'NONE', #505 ) ;
#16833=ORIENTED_EDGE ( 'NONE', *, *, #4464, .F. ) ;
#16837=DIRECTION ( 'NONE',  ( 1.000000000000000000, 0.000000000000000000, 0.000000000000000000 ) ) ;
#16841=DIRECTION ( 'NONE',  ( 0.000000000000000000, 0.000000000000000000, 1.000000000000000000 ) ) ;
#16852=AXIS2_PLACEMENT_3D ( 'NONE', #15921, #11052, #23327 ) ;
#16867=ORIENTED_EDGE ( 'NONE', *, *, #7961, .F. ) ;
#16872=DIRECTION ( 'NONE',  ( 0.000000000000000000, 0.000000000000000000, 1.000000000000000000 ) ) ;
#16878=CARTESIAN_POINT ( 'NONE',  ( 27.92857142820000149, 7.105427357599999217E-15, 142.0603150149999863 ) ) ;
#16887=CARTESIAN_POINT ( 'NONE',  ( 1.087565150579584028, -27.47889317205707727, 5.217914068007818429 ) ) ;
#16891=CARTESIAN_POINT ( 'NONE',  ( 22.95800505923639534, -13.82601854777970729, 5.993195172372761448 ) ) ;
#16892=DIRECTION ( 'NONE',  ( 0.000000000000000000, 0.000000000000000000, -1.000000000000000000 ) ) ;
#16893=DIRECTION ( 'NONE',  ( 1.000000000000000000, 0.000000000000000000, 0.000000000000000000 ) ) ;
#16896=VERTEX_POINT ( 'NONE', #17009 ) ;
#16900=CARTESIAN_POINT ( 'NONE',  ( 27.92857142860000152, 3.552713678799999608E-15, 92.06031501460000754 ) ) ;
#16922=DIRECTION ( 'NONE',  ( 1.000000000000000000, -1.224606353819998843E-16, 0.000000000000000000 ) ) ;
#16923=CARTESIAN_POINT ( 'NONE',  ( 23.45048833493306972, -12.97319122329745156, 224.0048062712651813 ) ) ;
#16926=DIRECTION ( 'NONE',  ( 0.000000000000000000, 0.000000000000000000, 1.000000000000000000 ) ) ;
#16937=DIRECTION ( 'NONE',  ( 0.000000000000000000, 0.000000000000000000, -1.000000000000000000 ) ) ;
#16939=ORIENTED_EDGE ( 'NONE', *, *, #27674, .F. ) ;
#16943=CARTESIAN_POINT ( 'NONE',  ( 0.000000000000000000, 0.000000000000000000, 210.0000000000000284 ) ) ;
#16950=ORIENTED_EDGE ( 'NONE', *, *, #22021, .F. ) ;
#16952=CYLINDRICAL_SURFACE ( 'NONE', #30260, 27.50000000000000000 ) ;
#16958=CARTESIAN_POINT ( 'NONE',  ( 27.76135143639999825, -3.399672735949999729E-15, 87.66141409839998744 ) ) ;
#16966=CARTESIAN_POINT ( 'NONE',  ( -8.903108651239966420, -22.82508830966961000, 40.00000000000000000 ) ) ;
#16971=AXIS2_PLACEMENT_3D ( 'NONE', #21071, #1718, #6429 ) ;
#16974=AXIS2_PLACEMENT_3D ( 'NONE', #12495, #12815, #24618 ) ;
#16977=AXIS2_PLACEMENT_3D ( 'NONE', #12926, #10418, #3167 ) ;
#16978=CARTESIAN_POINT ( 'NONE',  ( 2.373469614669200922, -26.70001233586149780, 19.99999999999999645 ) ) ;
#16979=VERTEX_POINT ( 'NONE', #3299 ) ;
#16982=DIRECTION ( 'NONE',  ( 0.000000000000000000, 0.000000000000000000, 1.000000000000000000 ) ) ;
#16991=ADVANCED_FACE ( 'NONE', ( #19985 ), #15717, .F. ) ;
#17002=CARTESIAN_POINT ( 'NONE',  ( -10.06596365874885812, -25.80632433378972124, 90.00000000000000000 ) ) ;
#17004=VERTEX_POINT ( 'NONE', #18228 ) ;
#17009=CARTESIAN_POINT ( 'NONE',  ( -27.50000000000000000, 3.367667473009999970E-15, 136.3944487260000074 ) ) ;
#17019=VECTOR ( 'NONE', #27217, 1000.000000000000000 ) ;
#17023=CARTESIAN_POINT ( 'NONE',  ( 23.67167941903707273, -13.99714051993749919, 6.071909320481077010 ) ) ;
#17025=ORIENTED_EDGE ( 'NONE', *, *, #8132, .F. ) ;
#17028=ORIENTED_EDGE ( 'NONE', *, *, #27509, .F. ) ;
#17029=DIRECTION ( 'NONE',  ( 0.000000000000000000, 0.000000000000000000, 1.000000000000000000 ) ) ;
#17030=AXIS2_PLACEMENT_3D ( 'NONE', #30331, #20569, #10824 ) ;
#17037=ADVANCED_FACE ( 'NONE', ( #17913 ), #27522, .T. ) ;
#17040=VERTEX_POINT ( 'NONE', #15562 ) ;
#17041=LINE ( 'NONE', #2572, #9458 ) ;
#17048=CARTESIAN_POINT ( 'NONE',  ( 26.84464183080000055, -3.287411895189999871E-15, 92.56249624490000372 ) ) ;
#17049=AXIS2_PLACEMENT_3D ( 'NONE', #11889, #4507, #19128 ) ;
#17068=DIRECTION ( 'NONE',  ( 0.9316362575375356503, 0.3633921898465274913, 0.000000000000000000 ) ) ;
#17080=CARTESIAN_POINT ( 'NONE',  ( 23.64633388422165083, -12.61377020549707417, 224.3610176357263128 ) ) ;
#17092=CARTESIAN_POINT ( 'NONE',  ( -24.24391315718250084, -12.98049462764927853, 5.674968348892686976 ) ) ;
#17098=ORIENTED_EDGE ( 'NONE', *, *, #3028, .F. ) ;
#17122=DIRECTION ( 'NONE',  ( 0.3633921898465273803, -0.9316362575375355393, 1.734723475976806306E-15 ) ) ;
#17125=CARTESIAN_POINT ( 'NONE',  ( 1.100000000000000089, -26.77741585740000119, 225.0000000000000000 ) ) ;
#17129=DIRECTION ( 'NONE',  ( 1.000000000000000000, 0.000000000000000000, 0.000000000000000000 ) ) ;
#17137=EDGE_LOOP ( 'NONE', ( #17492, #4876, #8237, #26238 ) ) ;
#17138=ORIENTED_EDGE ( 'NONE', *, *, #21269, .T. ) ;
#17140=ORIENTED_EDGE ( 'NONE', *, *, #981, .T. ) ;
#17146=EDGE_CURVE ( 'NONE', #902, #26900, #22246, .T. ) ;
#17148=CARTESIAN_POINT ( 'NONE',  ( 0.000000000000000000, 0.000000000000000000, 140.0000000000000000 ) ) ;
#17160=AXIS2_PLACEMENT_3D ( 'NONE', #22011, #12866, #22313 ) ;
#17168=AXIS2_PLACEMENT_3D ( 'NONE', #14842, #26946, #12315 ) ;
#17173=LINE ( 'NONE', #3158, #7303 ) ;
#17177=ORIENTED_EDGE ( 'NONE', *, *, #7194, .F. ) ;
#17178=VERTEX_POINT ( 'NONE', #12062 ) ;
#17181=CARTESIAN_POINT ( 'NONE',  ( -26.80000000000000071, 9.769962616700000205E-15, 36.78285841159999592 ) ) ;
#17183=ORIENTED_EDGE ( 'NONE', *, *, #27917, .T. ) ;
#17184=CARTESIAN_POINT ( 'NONE',  ( 0.000000000000000000, 0.000000000000000000, 40.00000000000000000 ) ) ;
#17185=AXIS2_PLACEMENT_3D ( 'NONE', #5160, #22015, #471 ) ;
#17193=CARTESIAN_POINT ( 'NONE',  ( 10.82908725742652223, -27.76276047461856678, 186.7828584120000244 ) ) ;
#17194=CARTESIAN_POINT ( 'NONE',  ( 7.453090060300407771, -2.907137518772283435, 210.0000000000000284 ) ) ;
#17196=CARTESIAN_POINT ( 'NONE',  ( 22.74641636092161434, -14.17229404674536042, 5.633487048338723824 ) ) ;
#17204=AXIS2_PLACEMENT_3D ( 'NONE', #12626, #26647, #17353 ) ;
#17217=FACE_OUTER_BOUND ( 'NONE', #5837, .T. ) ;
#17228=ORIENTED_EDGE ( 'NONE', *, *, #3291, .F. ) ;
#17245=VERTEX_POINT ( 'NONE', #26685 ) ;
#17255=AXIS2_PLACEMENT_3D ( 'NONE', #10024, #16784, #11913 ) ;
#17261=B_SPLINE_CURVE_WITH_KNOTS ( 'NONE', 3,
 ( #25367, #6154, #17497, #8192, #6000, #10426, #27102, #23004, #20018, #10888, #17796, #15599, #24743, #20478, #3175, #27406, #25201, #3805, #15448, #25050, #1131, #1453, #20324, #10722 ),
 .UNSPECIFIED., .F., .F.,
 ( 4, 2, 2, 2, 2, 2, 2, 2, 2, 2, 2, 4 ),
 ( 0.000000000000000000, 0.001576261392767915439, 0.002364392089151865026, 0.003152522785535814397, 0.004728784178303712706, 0.005516914874687660342, 0.006305045571071608845, 0.007881306963839505852, 0.009457568356607402860, 0.01024569905299135136, 0.01103382974937529813, 0.01261009114214319514 ),
 .UNSPECIFIED. ) ;
#17262=AXIS2_PLACEMENT_3D ( 'NONE', #29977, #12992, #24650 ) ;
#17269=CARTESIAN_POINT ( 'NONE',  ( 27.50000000000000000, -3.367667472999999580E-15, 93.60555127639999284 ) ) ;
#17275=LINE ( 'NONE', #22474, #21211 ) ;
#17278=CARTESIAN_POINT ( 'NONE',  ( 0.8466629623219488199, -26.78674366391425110, 224.2963572738258904 ) ) ;
#17281=AXIS2_PLACEMENT_3D ( 'NONE', #12667, #11056, #428 ) ;
#17294=VERTEX_POINT ( 'NONE', #25577 ) ;
#17303=DIRECTION ( 'NONE',  ( 0.000000000000000000, 0.000000000000000000, 1.000000000000000000 ) ) ;
#17306=TOROIDAL_SURFACE ( 'NONE', #1234, 24.50000000000000000, 3.200000000000000178 ) ;
#17319=CARTESIAN_POINT ( 'NONE',  ( 8.903108651239925564, -22.82508830966962421, 40.00000000000000000 ) ) ;
#17323=CIRCLE ( 'NONE', #6274, 2.999999999999999556 ) ;
#17325=EDGE_CURVE ( 'NONE', #12226, #18212, #27759, .T. ) ;
#17326=EDGE_CURVE ( 'NONE', #6137, #6530, #24759, .T. ) ;
#17329=ORIENTED_EDGE ( 'NONE', *, *, #25683, .T. ) ;
#17338=EDGE_CURVE ( 'NONE', #1526, #8364, #11714, .T. ) ;
#17341=DIRECTION ( 'NONE',  ( -0.9316362575375349842, 0.3633921898465292122, -0.000000000000000000 ) ) ;
#17348=AXIS2_PLACEMENT_3D ( 'NONE', #25995, #15762, #30239 ) ;
#17351=CARTESIAN_POINT ( 'NONE',  ( -18.95046173579999760, -18.95046173579999760, 193.2171415880000040 ) ) ;
#17353=DIRECTION ( 'NONE',  ( 1.000000000000000000, -1.224606353820000075E-16, 0.000000000000000000 ) ) ;
#17359=DIRECTION ( 'NONE',  ( 1.000000000000000000, -1.224606353820000075E-16, 0.000000000000000000 ) ) ;
#17360=VERTEX_POINT ( 'NONE', #16584 ) ;
#17370=DIRECTION ( 'NONE',  ( 0.000000000000000000, 0.000000000000000000, 1.000000000000000000 ) ) ;
#17373=CARTESIAN_POINT ( 'NONE',  ( -9.738910687886855655, -24.96785170200598714, 115.0000000000000000 ) ) ;
#17375=B_SPLINE_CURVE_WITH_KNOTS ( 'NONE', 3,
 ( #10753, #23038, #3665, #9434, #23192, #19037, #1484, #26279, #15944, #7080 ),
 .UNSPECIFIED., .F., .F.,
 ( 4, 2, 2, 2, 4 ),
 ( 0.000000000000000000, 0.2500000000000000555, 0.5000000000000001110, 0.7500000000000002220, 1.000000000000000000 ),
 .UNSPECIFIED. ) ;
#17379=CARTESIAN_POINT ( 'NONE',  ( -27.63177371730000331, 3.383804566159999695E-15, 192.6394760439999914 ) ) ;
#17380=CARTESIAN_POINT ( 'NONE',  ( 26.80000000000000071, -3.552713678799999608E-15, 193.2171415880000040 ) ) ;
#17381=VERTEX_POINT ( 'NONE', #2584 ) ;
#17384=EDGE_CURVE ( 'NONE', #6179, #10144, #16275, .T. ) ;
#17385=EDGE_CURVE ( 'NONE', #15899, #16404, #15203, .T. ) ;
#17393=DIRECTION ( 'NONE',  ( 0.8090169943751909232, 0.5877852522921378498, 0.000000000000000000 ) ) ;
#17398=CARTESIAN_POINT ( 'NONE',  ( -9.689803781819808393, -24.98716455116955970, 26.94264034010273434 ) ) ;
#17400=ORIENTED_EDGE ( 'NONE', *, *, #27403, .T. ) ;
#17413=CARTESIAN_POINT ( 'NONE',  ( -18.95046173579999760, -18.95046173579999760, 143.2171415880000040 ) ) ;
#17430=LINE ( 'NONE', #19803, #2128 ) ;
#17433=DIRECTION ( 'NONE',  ( 0.000000000000000000, 0.000000000000000000, 1.000000000000000000 ) ) ;
#17435=CARTESIAN_POINT ( 'NONE',  ( -22.29514036694590118, -14.89751301532326444, 43.21714158846668141 ) ) ;
#17444=EDGE_CURVE ( 'NONE', #18378, #28697, #1802, .T. ) ;
#17446=AXIS2_PLACEMENT_3D ( 'NONE', #30859, #23162, #23315 ) ;
#17448=VERTEX_POINT ( 'NONE', #9976 ) ;
#17449=AXIS2_PLACEMENT_3D ( 'NONE', #7970, #758, #19942 ) ;
#17450=ORIENTED_EDGE ( 'NONE', *, *, #10034, .T. ) ;
#17458=CARTESIAN_POINT ( 'NONE',  ( -9.738910687886855655, -24.96785170200598714, 115.0000000000000000 ) ) ;
#17469=VECTOR ( 'NONE', #3993, 1000.000000000000000 ) ;
#17478=VERTEX_POINT ( 'NONE', #26652 ) ;
#17484=EDGE_CURVE ( 'NONE', #8183, #26174, #21752, .T. ) ;
#17486=AXIS2_PLACEMENT_3D ( 'NONE', #10847, #20433, #22647 ) ;
#17490=CYLINDRICAL_SURFACE ( 'NONE', #17168, 1.100000000000000089 ) ;
#17492=ORIENTED_EDGE ( 'NONE', *, *, #5330, .T. ) ;
#17494=AXIS2_PLACEMENT_3D ( 'NONE', #6850, #1832, #25910 ) ;
#17495=CARTESIAN_POINT ( 'NONE',  ( 10.82908725742651512, -27.76276047461856322, 143.2171415880000040 ) ) ;
#17497=CARTESIAN_POINT ( 'NONE',  ( 3.160606383828830968, -27.32265456628853784, 209.9517185872548453 ) ) ;
#17509=CARTESIAN_POINT ( 'NONE',  ( -11.08346179031913437, -28.41490585489480480, 43.60555127550000520 ) ) ;
#17514=AXIS2_PLACEMENT_3D ( 'NONE', #15740, #20161, #22674 ) ;
#17517=VECTOR ( 'NONE', #17578, 1000.000000000000000 ) ;
#17533=VERTEX_POINT ( 'NONE', #12792 ) ;
#17535=AXIS2_PLACEMENT_3D ( 'NONE', #20377, #29968, #1505 ) ;
#17540=CARTESIAN_POINT ( 'NONE',  ( 23.24663841809999809, -14.69162354060000020, 225.0000000000000000 ) ) ;
#17542=CARTESIAN_POINT ( 'NONE',  ( -7.297190580108165570, -25.78810378223603195, 207.8834700269517270 ) ) ;
#17547=CARTESIAN_POINT ( 'NONE',  ( 0.000000000000000000, 0.000000000000000000, 115.0000000000000000 ) ) ;
#17548=CARTESIAN_POINT ( 'NONE',  ( -8.966526567020544292, -25.25634759429105003, 24.42360803256879720 ) ) ;
#17549=DIRECTION ( 'NONE',  ( 0.000000000000000000, 0.000000000000000000, -1.000000000000000000 ) ) ;
#17561=ORIENTED_EDGE ( 'NONE', *, *, #4678, .T. ) ;
#17562=CLOSED_SHELL ( 'NONE', ( #28933, #27939, #1452, #13691, #5662, #20227, #18589, #16991, #220, #11174, #20060, #3527, #14529, #13512, #7532, #3865, #8077, #30711, #20144, #13620, #8421, #10726, #2413, #10348, #22657, #7754, #15035, #2491, #9459, #20049, #10671, #13614, #15516, #26425, #16152, #8870, #28857, #9673, #9221, #10405, #21298, #29316, #8196, #22019, #16031, #30512, #15401, #10921, #12761, #26984, #16193, #13143, #22284, #17037, #5687, #4056, #14670, #7547, #7198, #1706, #25711, #27975, #1332, #11642, #14264, #14077, #4745, #2200, #17719, #24450, #19805, #19585, #30290, #30974, #30945, #8171, #27016, #14880, #8022, #15368, #29421, #9568, #504, #21452, #15407, #30854, #8403, #16810, #19625, #2355, #22584, #11811, #5270, #6862, #5795, #15250, #14658, #5208, #15742, #3318, #27230, #1326, #5338, #25792, #10390, #9679, #3174, #21966, #21770, #28899, #24951, #5002, #8349, #30615, #3670, #2541, #10176, #9860, #3898, #2582 ) ) ;
#17564=ORIENTED_EDGE ( 'NONE', *, *, #22922, .T. ) ;
#17578=DIRECTION ( 'NONE',  ( 0.000000000000000000, -1.000000000000000000, 0.000000000000000000 ) ) ;
#17583=CARTESIAN_POINT ( 'NONE',  ( 8.310304230308181772, -25.47941657935494675, 206.6944841980503043 ) ) ;
#17585=CARTESIAN_POINT ( 'NONE',  ( -25.90058877277586902, -6.940365930346065859, 43.21714158835417408 ) ) ;
#17586=EDGE_CURVE ( 'NONE', #14673, #23569, #23201, .T. ) ;
#17587=CARTESIAN_POINT ( 'NONE',  ( 5.851800771450333727, -26.15706768910720470, 21.02145656915469019 ) ) ;
#17610=DIRECTION ( 'NONE',  ( -0.000000000000000000, -0.000000000000000000, -1.000000000000000000 ) ) ;
#17619=CARTESIAN_POINT ( 'NONE',  ( -28.50000000000000000, 3.490128108389999698E-15, 140.0000000000000000 ) ) ;
#17624=CARTESIAN_POINT ( 'NONE',  ( -7.453090060300352704, -2.907137518772246132, 210.0000000000000284 ) ) ;
#17627=CARTESIAN_POINT ( 'NONE',  ( 0.000000000000000000, 0.000000000000000000, 0.000000000000000000 ) ) ;
#17629=CARTESIAN_POINT ( 'NONE',  ( -6.112033042629958501, -26.81582465834875251, 21.02319148660755133 ) ) ;
#17631=ORIENTED_EDGE ( 'NONE', *, *, #16565, .F. ) ;
#17633=ORIENTED_EDGE ( 'NONE', *, *, #16638, .F. ) ;
#17644=VECTOR ( 'NONE', #14927, 1000.000000000000114 ) ;
#17648=CARTESIAN_POINT ( 'NONE',  ( -28.50000000000000000, 3.490128108389999698E-15, 40.00000000000000000 ) ) ;
#17649=CARTESIAN_POINT ( 'NONE',  ( -27.92857142820000149, 5.329070518200000398E-15, 137.9396849850000137 ) ) ;
#17655=DIRECTION ( 'NONE',  ( 1.224606353819999829E-16, 1.000000000000000000, 0.000000000000000000 ) ) ;
#17658=FACE_OUTER_BOUND ( 'NONE', #14750, .T. ) ;
#17662=EDGE_CURVE ( 'NONE', #24922, #22997, #9180, .T. ) ;
#17664=VERTEX_POINT ( 'NONE', #6483 ) ;
#17667=VERTEX_POINT ( 'NONE', #10736 ) ;
#17675=CARTESIAN_POINT ( 'NONE',  ( 1.071233844162623683, -26.77863813579940455, 5.288095982889605473 ) ) ;
#17681=CARTESIAN_POINT ( 'NONE',  ( -23.20948082139999968, -13.40000000000000036, 3.900000000369999942 ) ) ;
#17683=EDGE_CURVE ( 'NONE', #12643, #24389, #28280, .T. ) ;
#17689=CARTESIAN_POINT ( 'NONE',  ( 1.100000000000000089, -27.47799119300000115, 225.0000000000000000 ) ) ;
#17693=CARTESIAN_POINT ( 'NONE',  ( -24.79654435811119484, -10.16723671460308154, 93.21714158839822062 ) ) ;
#17695=VECTOR ( 'NONE', #30143, 1000.000000000000000 ) ;
#17696=VERTEX_POINT ( 'NONE', #7110 ) ;
#17698=DIRECTION ( 'NONE',  ( 1.000000000000000000, -1.224606353820000075E-16, 0.000000000000000000 ) ) ;
#17705=ORIENTED_EDGE ( 'NONE', *, *, #25745, .T. ) ;
#17706=ORIENTED_EDGE ( 'NONE', *, *, #10254, .F. ) ;
#17718=DIRECTION ( 'NONE',  ( 0.8660254037843289066, -0.5000000000001899592, 0.000000000000000000 ) ) ;
#17719=ADVANCED_FACE ( 'NONE', ( #28195 ), #22753, .T. ) ;
#17722=AXIS2_PLACEMENT_3D ( 'NONE', #2627, #14015, #29203 ) ;
#17723=FACE_OUTER_BOUND ( 'NONE', #13816, .T. ) ;
#17728=EDGE_CURVE ( 'NONE', #24389, #27584, #31029, .T. ) ;
#17730=CARTESIAN_POINT ( 'NONE',  ( 2.898287520843013443, -26.64792758275491380, 209.9518913731128009 ) ) ;
#17733=CARTESIAN_POINT ( 'NONE',  ( 8.727399452413365566, -25.34090985533206108, 23.95427889024438173 ) ) ;
#17743=ORIENTED_EDGE ( 'NONE', *, *, #11278, .T. ) ;
#17744=ORIENTED_EDGE ( 'NONE', *, *, #17338, .F. ) ;
#17746=FACE_OUTER_BOUND ( 'NONE', #1338, .T. ) ;
#17758=EDGE_CURVE ( 'NONE', #28953, #19872, #6174, .T. ) ;
#17779=ORIENTED_EDGE ( 'NONE', *, *, #21062, .F. ) ;
#17780=CARTESIAN_POINT ( 'NONE',  ( -1.100000000000000089, -26.77741585740000119, 5.000000000000000000 ) ) ;
#17782=EDGE_LOOP ( 'NONE', ( #906, #13579, #1149, #25551 ) ) ;
#17784=ORIENTED_EDGE ( 'NONE', *, *, #26739, .F. ) ;
#17792=EDGE_LOOP ( 'NONE', ( #12997, #1831, #26621, #12482 ) ) ;
#17796=CARTESIAN_POINT ( 'NONE',  ( 6.965151789112639769, -26.60412671351617320, 208.3894876551769926 ) ) ;
#17801=CARTESIAN_POINT ( 'NONE',  ( -1.071537510008835126, -27.47917025540911951, 5.286989672262158102 ) ) ;
#17809=VECTOR ( 'NONE', #28813, 1000.000000000000000 ) ;
#17816=B_SPLINE_CURVE_WITH_KNOTS ( 'NONE', 3,
 ( #5635, #10835, #24842, #10212, #19959, #20421, #930, #29554, #30014, #8449 ),
 .UNSPECIFIED., .F., .F.,
 ( 4, 2, 2, 2, 4 ),
 ( 0.000000000000000000, 0.2500000000000000000, 0.5000000000000000000, 0.7500000000000000000, 1.000000000000000000 ),
 .UNSPECIFIED. ) ;
#17823=( NAMED_UNIT ( * ) PLANE_ANGLE_UNIT ( ) SI_UNIT ( $, .RADIAN. ) );
#17838=CARTESIAN_POINT ( 'NONE',  ( -27.23548387100000312, 1.421085471519999843E-14, 91.66046017469999185 ) ) ;
#17847=CARTESIAN_POINT ( 'NONE',  ( 27.92857142820000149, 7.105427357599999217E-15, 142.0603150149999863 ) ) ;
#17849=ORIENTED_EDGE ( 'NONE', *, *, #6964, .T. ) ;
#17851=DIRECTION ( 'NONE',  ( 0.000000000000000000, 0.000000000000000000, -1.000000000000000000 ) ) ;
#17852=CARTESIAN_POINT ( 'NONE',  ( -25.15951549259923326, -9.235088186050580461, 93.21714158838125286 ) ) ;
#17862=VERTEX_POINT ( 'NONE', #17619 ) ;
#17881=DIRECTION ( 'NONE',  ( 0.000000000000000000, 0.000000000000000000, 1.000000000000000000 ) ) ;
#17885=CARTESIAN_POINT ( 'NONE',  ( 5.852082250035302913, -26.15431190117149285, 208.9630145448510916 ) ) ;
#17887=CARTESIAN_POINT ( 'NONE',  ( -25.51870711004139380, -8.199261060474283269, 43.21714158836665831 ) ) ;
#17888=CARTESIAN_POINT ( 'NONE',  ( 4.671347416477003023, -26.39088508839783032, 20.48731328533980545 ) ) ;
#17893=CARTESIAN_POINT ( 'NONE',  ( 0.000000000000000000, 0.000000000000000000, 115.0000000000000000 ) ) ;
#17898=B_SPLINE_CURVE_WITH_KNOTS ( 'NONE', 3,
 ( #12786, #27108, #10124, #10730, #10431, #29620, #29303, #19879, #15147, #17351 ),
 .UNSPECIFIED., .F., .F.,
 ( 4, 2, 2, 2, 4 ),
 ( 0.000000000000000000, 0.2500000000000000000, 0.5000000000000000000, 0.7500000000000000000, 1.000000000000000000 ),
 .UNSPECIFIED. ) ;
#17913=FACE_OUTER_BOUND ( 'NONE', #11961, .T. ) ;
#17930=CARTESIAN_POINT ( 'NONE',  ( -1.099927927653325810, -26.77741881808574220, 4.854121423575340266 ) ) ;
#17932=VERTEX_POINT ( 'NONE', #24107 ) ;
#17940=ORIENTED_EDGE ( 'NONE', *, *, #29494, .T. ) ;
#17946=TOROIDAL_SURFACE ( 'NONE', #30536, 29.80000000000000071, 3.000000000000000000 ) ;
#17950=AXIS2_PLACEMENT_3D ( 'NONE', #8414, #10337, #27620 ) ;
#17958=CARTESIAN_POINT ( 'NONE',  ( 23.25354871338156570, -14.68148953523539468, 224.7820750499900839 ) ) ;
#17978=EDGE_CURVE ( 'NONE', #22441, #18380, #26928, .T. ) ;
#17984=CARTESIAN_POINT ( 'NONE',  ( -23.70259205116592227, -12.50815390717660058, 5.420582064722430538 ) ) ;
#17986=AXIS2_PLACEMENT_3D ( 'NONE', #684, #10276, #5538 ) ;
#17987=ORIENTED_EDGE ( 'NONE', *, *, #26458, .F. ) ;
#17993=DIRECTION ( 'NONE',  ( -0.7071067811865475727, 0.7071067811865475727, 0.000000000000000000 ) ) ;
#17996=FACE_OUTER_BOUND ( 'NONE', #24588, .T. ) ;
#18001=DIRECTION ( 'NONE',  ( 0.3633921898465276024, -0.9316362575375355393, -1.301042606982605321E-14 ) ) ;
#18007=CYLINDRICAL_SURFACE ( 'NONE', #1785, 26.80000000000002203 ) ;
#18008=TOROIDAL_SURFACE ( 'NONE', #30092, 29.80000000000000071, 3.000000000000000000 ) ;
#18010=CARTESIAN_POINT ( 'NONE',  ( -23.81569860410000317, -13.75000000000000000, 226.0999999999999943 ) ) ;
#18018=CIRCLE ( 'NONE', #4484, 4.000000004070001225 ) ;
#18020=VERTEX_POINT ( 'NONE', #12909 ) ;
#18024=B_SPLINE_CURVE_WITH_KNOTS ( 'NONE', 3,
 ( #23074, #8734, #6221, #27616, #4179, #8570, #13776, #1827, #8411, #18010 ),
 .UNSPECIFIED., .F., .F.,
 ( 4, 2, 2, 2, 4 ),
 ( 0.000000000000000000, 0.2500000000000000000, 0.5000000000000000000, 0.7500000000000000000, 1.000000000000000000 ),
 .UNSPECIFIED. ) ;
#18027=CARTESIAN_POINT ( 'NONE',  ( -9.897162125286943279, -25.37356426548037547, 138.3395398250000028 ) ) ;
#18037=DIRECTION ( 'NONE',  ( -0.9316362575375349842, 0.3633921898465292122, -0.000000000000000000 ) ) ;
#18041=VECTOR ( 'NONE', #26982, 1000.000000000000000 ) ;
#18045=CARTESIAN_POINT ( 'NONE',  ( -19.81582138730395926, -18.05844329259049985, 43.21714158843889919 ) ) ;
#18051=FACE_OUTER_BOUND ( 'NONE', #9798, .T. ) ;
#18053=ORIENTED_EDGE ( 'NONE', *, *, #23014, .T. ) ;
#18060=DIRECTION ( 'NONE',  ( 0.3633921898465272138, -0.9316362575375356503, 9.251858538542967489E-15 ) ) ;
#18062=CIRCLE ( 'NONE', #6013, 4.000000000000000888 ) ;
#18080=CARTESIAN_POINT ( 'NONE',  ( -27.63177371540000138, 3.383804565929999804E-15, 92.63947604839999883 ) ) ;
#18083=VECTOR ( 'NONE', #4099, 1000.000000000000000 ) ;
#18088=DIRECTION ( 'NONE',  ( -1.000000000000000000, 0.000000000000000000, 0.000000000000000000 ) ) ;
#18091=CARTESIAN_POINT ( 'NONE',  ( -0.9560303848909833535, -26.78297053551130702, 4.451032274715761794 ) ) ;
#18092=ORIENTED_EDGE ( 'NONE', *, *, #7848, .F. ) ;
#18099=ORIENTED_EDGE ( 'NONE', *, *, #8628, .F. ) ;
#18112=CARTESIAN_POINT ( 'NONE',  ( -4.195523629574152480, -27.17925737118813956, 209.7419767459480227 ) ) ;
#18123=CARTESIAN_POINT ( 'NONE',  ( 9.738910687886868089, -24.96785170200598358, 136.7828584120000244 ) ) ;
#18130=ORIENTED_EDGE ( 'NONE', *, *, #18856, .F. ) ;
#18134=CARTESIAN_POINT ( 'NONE',  ( 28.50000000000000000, -3.490128108379999702E-15, 140.0000000000000000 ) ) ;
#18153=EDGE_CURVE ( 'NONE', #17533, #7025, #14930, .T. ) ;
#18154=DIRECTION ( 'NONE',  ( 0.8090169943751909232, 0.5877852522921378498, 0.000000000000000000 ) ) ;
#18170=TOROIDAL_SURFACE ( 'NONE', #4614, 30.50000000000000000, 3.000000000000000000 ) ;
#18172=CARTESIAN_POINT ( 'NONE',  ( -1.065814103639999922E-14, 1.421085471519999843E-14, 186.3944487249999895 ) ) ;
#18205=VECTOR ( 'NONE', #12023, 1000.000000000000000 ) ;
#18207=ORIENTED_EDGE ( 'NONE', *, *, #20784, .F. ) ;
#18212=VERTEX_POINT ( 'NONE', #27038 ) ;
#18228=CARTESIAN_POINT ( 'NONE',  ( -18.95046173579999760, -18.95046173579999760, 36.78285841159999592 ) ) ;
#18237=VERTEX_POINT ( 'NONE', #473 ) ;
#18239=AXIS2_PLACEMENT_3D ( 'NONE', #25812, #8960, #13528 ) ;
#18243=VERTEX_POINT ( 'NONE', #3266 ) ;
#18244=CIRCLE ( 'NONE', #16747, 26.80000000000000071 ) ;
#18252=VERTEX_POINT ( 'NONE', #20575 ) ;
#18262=CARTESIAN_POINT ( 'NONE',  ( -26.80000000069999899, 3.281945028329999726E-15, 137.1101814800000227 ) ) ;
#18263=CARTESIAN_POINT ( 'NONE',  ( -25.94183207552246273, -6.953987411061866020, -0.000000000000000000 ) ) ;
#18265=AXIS2_PLACEMENT_3D ( 'NONE', #26125, #13853, #11175 ) ;
#18271=CARTESIAN_POINT ( 'NONE',  ( -9.221751571650349533, -25.90851042236080914, 205.5747784761970820 ) ) ;
#18281=EDGE_CURVE ( 'NONE', #13263, #6773, #8180, .T. ) ;
#18284=VERTEX_POINT ( 'NONE', #24835 ) ;
#18286=CARTESIAN_POINT ( 'NONE',  ( -16.20306687547018143, -21.42689369263768029, 36.78285841147716440 ) ) ;
#18292=DIRECTION ( 'NONE',  ( 0.000000000000000000, 0.000000000000000000, 1.000000000000000000 ) ) ;
#18294=VERTEX_POINT ( 'NONE', #10363 ) ;
#18301=CARTESIAN_POINT ( 'NONE',  ( 24.33346004068834034, -12.81155130650358132, 4.713248588629746827 ) ) ;
#18316=DIRECTION ( 'NONE',  ( -1.000000000000000000, 1.224606353819999829E-16, 0.000000000000000000 ) ) ;
#18327=B_SPLINE_CURVE_WITH_KNOTS ( 'NONE', 5,
 ( #5222, #11849, #23816, #9485, #2264, #21924 ),
 .UNSPECIFIED., .F., .F.,
 ( 6, 6 ),
 ( 0.000000000000000000, 2.319814892610000179 ),
 .UNSPECIFIED. ) ;
#18336=TOROIDAL_SURFACE ( 'NONE', #3255, 24.50000000000000000, 4.000000000000000000 ) ;
#18349=ORIENTED_EDGE ( 'NONE', *, *, #1919, .T. ) ;
#18356=FILL_AREA_STYLE ('',( #18814 ) ) ;
#18358=CARTESIAN_POINT ( 'NONE',  ( -7.105427357599999217E-15, 0.000000000000000000, 86.78285841159998881 ) ) ;
#18363=ORIENTED_EDGE ( 'NONE', *, *, #947, .T. ) ;
#18374=CARTESIAN_POINT ( 'NONE',  ( -23.24663841809999809, -14.69162354060000020, 5.000000000000000000 ) ) ;
#18377=CARTESIAN_POINT ( 'NONE',  ( -1.087768546147131588, -27.47890868157812605, 224.7820750495661741 ) ) ;
#18378=VERTEX_POINT ( 'NONE', #17380 ) ;
#18380=VERTEX_POINT ( 'NONE', #26985 ) ;
#18391=CARTESIAN_POINT ( 'NONE',  ( -0.09701118521228915825, -27.50000000070000539, 3.900000000000003020 ) ) ;
#18400=CARTESIAN_POINT ( 'NONE',  ( -1.087555935801710172, -26.77834284441886226, 5.218051574395796699 ) ) ;
#18405=FACE_OUTER_BOUND ( 'NONE', #1436, .T. ) ;
#18414=ORIENTED_EDGE ( 'NONE', *, *, #4030, .F. ) ;
#18416=ORIENTED_EDGE ( 'NONE', *, *, #14303, .F. ) ;
#18417=EDGE_LOOP ( 'NONE', ( #4883, #8656, #875, #16833, #17098 ) ) ;
#18425=FACE_OUTER_BOUND ( 'NONE', #28424, .T. ) ;
#18427=CARTESIAN_POINT ( 'NONE',  ( 8.903108651239925564, -22.82508830966962421, 190.0000000000000000 ) ) ;
#18441=CARTESIAN_POINT ( 'NONE',  ( -8.903108651239966420, -22.82508830966961000, 140.0000000000000000 ) ) ;
#18447=VERTEX_POINT ( 'NONE', #21964 ) ;
#18464=CARTESIAN_POINT ( 'NONE',  ( -6.394884621839999216E-14, -26.80000000000000071, 226.0999999999999943 ) ) ;
#18470=ORIENTED_EDGE ( 'NONE', *, *, #11756, .F. ) ;
#18474=CARTESIAN_POINT ( 'NONE',  ( 24.08872333959831380, -11.87645233066226069, 136.7828584119999960 ) ) ;
#18478=DIRECTION ( 'NONE',  ( 0.3090169943750400994, -0.9510565162951234441, 0.000000000000000000 ) ) ;
#18483=AXIS2_PLACEMENT_3D ( 'NONE', #11544, #20675, #1639 ) ;
#18486=CARTESIAN_POINT ( 'NONE',  ( 0.000000000000000000, 0.000000000000000000, 210.0000000000000284 ) ) ;
#18487=ORIENTED_EDGE ( 'NONE', *, *, #14841, .T. ) ;
#18507=CARTESIAN_POINT ( 'NONE',  ( 24.49999999589999788, -3.000285566359999846E-15, 190.0000000000000000 ) ) ;
#18510=VECTOR ( 'NONE', #23283, 1000.000000000000000 ) ;
#18511=DIRECTION ( 'NONE',  ( -0.3090169943750401549, -0.9510565162951233331, 0.000000000000000000 ) ) ;
#18526=CARTESIAN_POINT ( 'NONE',  ( -23.30309534863303256, -14.60301215427377031, 5.490554140840532504 ) ) ;
#18532=TOROIDAL_SURFACE ( 'NONE', #4967, 24.50000000000000000, 3.200000000000000178 ) ;
#18538=CARTESIAN_POINT ( 'NONE',  ( 0.000000000000000000, 0.000000000000000000, 87.93968498540000667 ) ) ;
#18544=FACE_OUTER_BOUND ( 'NONE', #16065, .T. ) ;
#18546=DIRECTION ( 'NONE',  ( 0.000000000000000000, 0.000000000000000000, 1.000000000000000000 ) ) ;
#18554=VECTOR ( 'NONE', #3057, 1000.000000000000000 ) ;
#18556=CARTESIAN_POINT ( 'NONE',  ( -1.100000000000000089, -26.77741585740000119, 5.000000000000000000 ) ) ;
#18564=EDGE_CURVE ( 'NONE', #25887, #17381, #4697, .T. ) ;
#18565=DIRECTION ( 'NONE',  ( -1.224606353819999829E-16, -1.000000000000000000, 0.000000000000000000 ) ) ;
#18567=CARTESIAN_POINT ( 'NONE',  ( -22.63992238019999803, -14.34133587289999845, 225.0000000000000000 ) ) ;
#18577=DIRECTION ( 'NONE',  ( 0.000000000000000000, 0.000000000000000000, 1.000000000000000000 ) ) ;
#18589=ADVANCED_FACE ( 'NONE', ( #2835 ), #798, .F. ) ;
#18592=CARTESIAN_POINT ( 'NONE',  ( -6.336630981016737607, -26.76091511895456776, 208.8270003598715050 ) ) ;
#18605=ORIENTED_EDGE ( 'NONE', *, *, #24494, .F. ) ;
#18606=CARTESIAN_POINT ( 'NONE',  ( 9.993285220779439371, -25.61999708228226069, 115.0000000000000000 ) ) ;
#18610=CARTESIAN_POINT ( 'NONE',  ( 20.19076655603537418, -17.71015691556361205, 186.7828584119999675 ) ) ;
#18611=EDGE_LOOP ( 'NONE', ( #6957, #16075, #11613, #24227 ) ) ;
#18616=CARTESIAN_POINT ( 'NONE',  ( 23.25354871329972895, -14.68148953537714441, 4.782075050810997041 ) ) ;
#18618=EDGE_CURVE ( 'NONE', #7124, #25355, #10236, .T. ) ;
#18620=APPLICATION_CONTEXT ( 'automotive_design' ) ;
#18631=DIRECTION ( 'NONE',  ( 0.000000000000000000, 0.000000000000000000, -1.000000000000000000 ) ) ;
#18637=CARTESIAN_POINT ( 'NONE',  ( -23.81569860410000317, -13.75000000000000000, 226.0999999999999943 ) ) ;
#18639=ORIENTED_EDGE ( 'NONE', *, *, #23286, .T. ) ;
#18642=FACE_OUTER_BOUND ( 'NONE', #18777, .T. ) ;
#18647=ORIENTED_EDGE ( 'NONE', *, *, #4639, .F. ) ;
#18648=CARTESIAN_POINT ( 'NONE',  ( 27.50000000000000000, -3.367667472999999580E-15, 36.71909809219999943 ) ) ;
#18656=SURFACE_STYLE_FILL_AREA ( #18356 ) ;
#18657=CARTESIAN_POINT ( 'NONE',  ( 27.92857142860000152, -3.116236426490000064E-16, 42.06031501460000044 ) ) ;
#18659=EDGE_CURVE ( 'NONE', #13152, #18447, #4084, .T. ) ;
#18664=CARTESIAN_POINT ( 'NONE',  ( -27.23548387060000309, 8.881784196999999612E-15, 191.6604601750000256 ) ) ;
#18679=CARTESIAN_POINT ( 'NONE',  ( -24.05715877267779490, -13.32261293328696539, 224.0051167719747696 ) ) ;
#18693=DIRECTION ( 'NONE',  ( 0.000000000000000000, 0.000000000000000000, 1.000000000000000000 ) ) ;
#18699=CARTESIAN_POINT ( 'NONE',  ( 7.105427357599999217E-15, 0.000000000000000000, 136.3944487250000179 ) ) ;
#18707=VECTOR ( 'NONE', #18631, 1000.000000000000000 ) ;
#18716=CARTESIAN_POINT ( 'NONE',  ( -27.69999999930000101, 3.392159599999999562E-15, 140.0000000000000000 ) ) ;
#18720=LINE ( 'NONE', #6306, #18083 ) ;
#18721=ORIENTED_EDGE ( 'NONE', *, *, #15572, .T. ) ;
#18723=ORIENTED_EDGE ( 'NONE', *, *, #6705, .T. ) ;
#18730=CARTESIAN_POINT ( 'NONE',  ( 27.69999999930000101, -3.392159599989999961E-15, 40.00000000000000000 ) ) ;
#18745=CARTESIAN_POINT ( 'NONE',  ( -23.48238834522544494, -12.91648733505556201, 224.0393715185676626 ) ) ;
#18746=DIRECTION ( 'NONE',  ( 1.000000000000000000, 0.000000000000000000, 0.000000000000000000 ) ) ;
#18751=CARTESIAN_POINT ( 'NONE',  ( 0.000000000000000000, 0.000000000000000000, 86.39444872359999295 ) ) ;
#18761=CARTESIAN_POINT ( 'NONE',  ( 26.80000000069999899, -3.281945028320000125E-15, 165.0000000000000000 ) ) ;
#18767=VERTEX_POINT ( 'NONE', #10511 ) ;
#18770=VECTOR ( 'NONE', #9741, 1000.000000000000000 ) ;
#18773=AXIS2_PLACEMENT_3D ( 'NONE', #18172, #6220, #13458 ) ;
#18777=EDGE_LOOP ( 'NONE', ( #8537, #11145, #2349, #28045 ) ) ;
#18780=CARTESIAN_POINT ( 'NONE',  ( 24.08627744698562267, -11.88207008772947049, 0.000000000000000000 ) ) ;
#18785=CARTESIAN_POINT ( 'NONE',  ( 0.000000000000000000, 0.000000000000000000, 115.0000000000000000 ) ) ;
#18793=EDGE_CURVE ( 'NONE', #23982, #4159, #19189, .T. ) ;
#18801=CARTESIAN_POINT ( 'NONE',  ( 24.49999999470000134, -3.000285566199999922E-15, 89.99999999930000172 ) ) ;
#18810=CIRCLE ( 'NONE', #23349, 26.80000000000000071 ) ;
#18811=DIRECTION ( 'NONE',  ( 1.000000000000000000, 0.000000000000000000, 0.000000000000000000 ) ) ;
#18814=FILL_AREA_STYLE_COLOUR ( '', #12045 ) ;
#18823=FACE_OUTER_BOUND ( 'NONE', #14171, .T. ) ;
#18838=ORIENTED_EDGE ( 'NONE', *, *, #14126, .T. ) ;
#18839=AXIS2_PLACEMENT_3D ( 'NONE', #23850, #9983, #31077 ) ;
#18841=CARTESIAN_POINT ( 'NONE',  ( -0.09666810103353495887, -27.50000000000000711, 223.9000000000000057 ) ) ;
#18856=EDGE_CURVE ( 'NONE', #11023, #20745, #6242, .T. ) ;
#18875=CYLINDRICAL_SURFACE ( 'NONE', #20314, 1.100000000000000089 ) ;
#18883=FACE_OUTER_BOUND ( 'NONE', #20213, .T. ) ;
#18886=ORIENTED_EDGE ( 'NONE', *, *, #2018, .F. ) ;
#18888=ORIENTED_EDGE ( 'NONE', *, *, #19533, .T. ) ;
#18903=DIRECTION ( 'NONE',  ( 0.000000000000000000, 0.000000000000000000, -1.000000000000000000 ) ) ;
#18912=ORIENTED_EDGE ( 'NONE', *, *, #21391, .T. ) ;
#18928=CARTESIAN_POINT ( 'NONE',  ( -9.993285220779425160, -25.61999708228226069, 115.0000000000000000 ) ) ;
#18948=DIRECTION ( 'NONE',  ( 1.000000000000000000, 0.000000000000000000, 0.000000000000000000 ) ) ;
#18951=EDGE_LOOP ( 'NONE', ( #5793, #9563, #19194, #1902, #559 ) ) ;
#18957=EDGE_CURVE ( 'NONE', #4180, #12069, #27642, .T. ) ;
#18961=AXIS2_PLACEMENT_3D ( 'NONE', #14304, #26415, #23911 ) ;
#18965=EDGE_LOOP ( 'NONE', ( #2875, #18487, #30069, #10134, #10627 ) ) ;
#18968=ORIENTED_EDGE ( 'NONE', *, *, #5805, .F. ) ;
#18971=CARTESIAN_POINT ( 'NONE',  ( 27.50000000000000000, -3.367667472999999580E-15, 43.28090191849999968 ) ) ;
#18973=CARTESIAN_POINT ( 'NONE',  ( 9.897162125286888212, -25.37356426548039678, 138.3395398250000028 ) ) ;
#18977=CARTESIAN_POINT ( 'NONE',  ( 0.9560301455467571374, -26.78297054432951896, 225.5489681738553713 ) ) ;
#18987=CYLINDRICAL_SURFACE ( 'NONE', #240, 27.50000000000000000 ) ;
#19005=ORIENTED_EDGE ( 'NONE', *, *, #6912, .T. ) ;
#19013=CARTESIAN_POINT ( 'NONE',  ( 27.50000000000000000, 1.776356839399999804E-15, 86.39444872449999480 ) ) ;
#19019=AXIS2_PLACEMENT_3D ( 'NONE', #28143, #300, #9569 ) ;
#19025=CARTESIAN_POINT ( 'NONE',  ( 27.76135144349999706, -3.399672736829999707E-15, 192.3385858899999903 ) ) ;
#19030=EDGE_CURVE ( 'NONE', #24695, #13818, #12642, .T. ) ;
#19037=CARTESIAN_POINT ( 'NONE',  ( -24.08872333959829959, -11.87645233066230332, 186.7828584124166866 ) ) ;
#19040=ORIENTED_EDGE ( 'NONE', *, *, #27545, .T. ) ;
#19047=PLANE ( 'NONE',  #2504 ) ;
#19049=DIRECTION ( 'NONE',  ( -1.224606353819999829E-16, -1.000000000000000000, 0.000000000000000000 ) ) ;
#19061=CARTESIAN_POINT ( 'NONE',  ( 14.94562240850000023, -8.628859120750000500, 5.000000000000000000 ) ) ;
#19063=DIRECTION ( 'NONE',  ( 0.000000000000000000, 0.000000000000000000, -1.000000000000000000 ) ) ;
#19068=DIRECTION ( 'NONE',  ( 0.3090169943750400994, -0.9510565162951234441, 0.000000000000000000 ) ) ;
#19077=AXIS2_PLACEMENT_3D ( 'NONE', #15797, #3675, #12820 ) ;
#19080=CARTESIAN_POINT ( 'NONE',  ( 23.26185891373408055, -14.66761890384653633, 5.286751411448414650 ) ) ;
#19088=DIRECTION ( 'NONE',  ( 0.3633921898465292122, 0.9316362575375348731, 3.469446951953613400E-15 ) ) ;
#19101=CARTESIAN_POINT ( 'NONE',  ( 27.06563796540000411, -3.314475222259999564E-15, 88.05973140640000452 ) ) ;
#19103=DIRECTION ( 'NONE',  ( 0.3633921898465291567, 0.9316362575375349842, 1.850371707708594444E-14 ) ) ;
#19105=CARTESIAN_POINT ( 'NONE',  ( 22.77466902168790241, -14.12660345740818713, 5.703642738130775491 ) ) ;
#19114=CIRCLE ( 'NONE', #35, 4.000000004070001225 ) ;
#19120=ORIENTED_EDGE ( 'NONE', *, *, #18957, .F. ) ;
#19123=ORIENTED_EDGE ( 'NONE', *, *, #3411, .T. ) ;
#19125=CARTESIAN_POINT ( 'NONE',  ( 27.23548387060000309, -1.776356839399999804E-15, 138.3395398250000028 ) ) ;
#19127=EDGE_CURVE ( 'NONE', #21856, #17533, #29740, .T. ) ;
#19128=DIRECTION ( 'NONE',  ( -1.000000000000000000, 5.665498452320000818E-16, 0.000000000000000000 ) ) ;
#19148=CIRCLE ( 'NONE', #21151, 3.000000000000001332 ) ;
#19151=CARTESIAN_POINT ( 'NONE',  ( -2.107992564109736566, -27.41908764619380889, 20.00000000000000355 ) ) ;
#19152=B_SPLINE_CURVE_WITH_KNOTS ( 'NONE', 5,
 ( #25864, #10745, #13255, #22873, #1315, #14519 ),
 .UNSPECIFIED., .F., .F.,
 ( 6, 6 ),
 ( 0.000000000000000000, 2.319814964899999943 ),
 .UNSPECIFIED. ) ;
#19156=CARTESIAN_POINT ( 'NONE',  ( 27.50000000000000000, -3.367667472999999580E-15, 43.60555127639999995 ) ) ;
#19157=EDGE_CURVE ( 'NONE', #17178, #10044, #2612, .T. ) ;
#19172=CARTESIAN_POINT ( 'NONE',  ( 27.63177356690000153, -3.383804547719999749E-15, 87.36052363810000543 ) ) ;
#19175=ORIENTED_EDGE ( 'NONE', *, *, #5213, .T. ) ;
#19184=CARTESIAN_POINT ( 'NONE',  ( 0.09707459473891824620, -26.79999999950000245, 223.8999999999999773 ) ) ;
#19189=CIRCLE ( 'NONE', #17160, 27.50000000000000000 ) ;
#19194=ORIENTED_EDGE ( 'NONE', *, *, #20932, .F. ) ;
#19199=ORIENTED_EDGE ( 'NONE', *, *, #9606, .T. ) ;
#19200=ORIENTED_EDGE ( 'NONE', *, *, #19773, .F. ) ;
#19203=CARTESIAN_POINT ( 'NONE',  ( -27.50000000000000000, 3.367667473009999970E-15, 230.0000000000000000 ) ) ;
#19204=LINE ( 'NONE', #14493, #20295 ) ;
#19217=EDGE_CURVE ( 'NONE', #16204, #25641, #2840, .T. ) ;
#19232=CARTESIAN_POINT ( 'NONE',  ( -23.20948082139999968, -13.40000000000000036, 226.0999999999999943 ) ) ;
#19236=EDGE_CURVE ( 'NONE', #5207, #15698, #21195, .T. ) ;
#19239=EDGE_LOOP ( 'NONE', ( #24811, #23231, #25867, #9359, #16371, #20003 ) ) ;
#19240=CARTESIAN_POINT ( 'NONE',  ( -23.24663841809999809, -14.69162354060000020, 5.000000000000000000 ) ) ;
#19241=FACE_OUTER_BOUND ( 'NONE', #27277, .T. ) ;
#19252=EDGE_CURVE ( 'NONE', #28706, #14673, #15647, .T. ) ;
#19256=VECTOR ( 'NONE', #7675, 1000.000000000000000 ) ;
#19266=EDGE_LOOP ( 'NONE', ( #14297, #538, #28785, #680 ) ) ;
#19270=EDGE_CURVE ( 'NONE', #21606, #4812, #9186, .T. ) ;
#19271=CARTESIAN_POINT ( 'NONE',  ( -1.421085471519999843E-14, -3.552713678799999608E-15, 136.3944487250000179 ) ) ;
#19279=ORIENTED_EDGE ( 'NONE', *, *, #9204, .F. ) ;
#19290=VECTOR ( 'NONE', #2778, 1000.000000000000114 ) ;
#19295=TOROIDAL_SURFACE ( 'NONE', #23323, 30.50000000000000000, 3.000000000000000000 ) ;
#19299=FACE_OUTER_BOUND ( 'NONE', #13666, .T. ) ;
#19300=VECTOR ( 'NONE', #16841, 1000.000000000000000 ) ;
#19302=CARTESIAN_POINT ( 'NONE',  ( -1.018916986751970954, -26.78112380549244520, 225.4205820666702493 ) ) ;
#19322=AXIS2_PLACEMENT_3D ( 'NONE', #15494, #29965, #3531 ) ;
#19331=( GEOMETRIC_REPRESENTATION_CONTEXT ( 3 ) GLOBAL_UNCERTAINTY_ASSIGNED_CONTEXT ( ( #20063 ) ) GLOBAL_UNIT_ASSIGNED_CONTEXT ( ( #5410, #24925, #27279 ) ) REPRESENTATION_CONTEXT ( 'NONE', 'WORKASPACE' ) );
#19348=CARTESIAN_POINT ( 'NONE',  ( 1.841797396446237967, -26.73663745407121795, 20.00000000000000355 ) ) ;
#19354=VERTEX_POINT ( 'NONE', #2846 ) ;
#19380=CARTESIAN_POINT ( 'NONE',  ( -2.947640775130000104E-14, -27.50000000000000000, 115.0000000000000000 ) ) ;
#19381=CARTESIAN_POINT ( 'NONE',  ( 3.163284386374760171, -27.32243547426061170, 20.04829674322551725 ) ) ;
#19415=CARTESIAN_POINT ( 'NONE',  ( 23.09885119083424598, -13.58970609041621636, 6.087620938929605430 ) ) ;
#19438=CARTESIAN_POINT ( 'NONE',  ( -2.947640775130000104E-14, -27.50000000000000000, 20.00000000000000355 ) ) ;
#19455=CARTESIAN_POINT ( 'NONE',  ( -0.2196051059861325316, -26.79904497468144342, 226.0876209393746592 ) ) ;
#19471=VERTEX_POINT ( 'NONE', #5972 ) ;
#19475=ORIENTED_EDGE ( 'NONE', *, *, #27917, .F. ) ;
#19480=AXIS2_PLACEMENT_3D ( 'NONE', #12735, #18693, #13354 ) ;
#19495=CARTESIAN_POINT ( 'NONE',  ( 27.50000000000000000, -3.367667472999999580E-15, 193.2809019210000088 ) ) ;
#19503=AXIS2_PLACEMENT_3D ( 'NONE', #1161, #3206, #3511 ) ;
#19504=CARTESIAN_POINT ( 'NONE',  ( -1.100000000000000089, -17.25771824079999917, 225.0000000000000000 ) ) ;
#19505=VERTEX_POINT ( 'NONE', #6127 ) ;
#19519=FACE_OUTER_BOUND ( 'NONE', #16522, .T. ) ;
#19533=EDGE_CURVE ( 'NONE', #7386, #11151, #5612, .T. ) ;
#19534=FACE_OUTER_BOUND ( 'NONE', #30771, .T. ) ;
#19538=CARTESIAN_POINT ( 'NONE',  ( 4.195523629574170243, -27.17925737118813956, 20.25802325405198800 ) ) ;
#19548=CARTESIAN_POINT ( 'NONE',  ( 0.000000000000000000, 0.000000000000000000, 138.3395398250000028 ) ) ;
#19556=AXIS2_PLACEMENT_3D ( 'NONE', #16966, #7978, #14620 ) ;
#19557=CARTESIAN_POINT ( 'NONE',  ( -8.903108651239966420, -22.82508830966961000, 190.0000000000000000 ) ) ;
#19559=EDGE_CURVE ( 'NONE', #23263, #21137, #29475, .T. ) ;
#19585=ADVANCED_FACE ( 'NONE', ( #9893 ), #4117, .F. ) ;
#19589=CARTESIAN_POINT ( 'NONE',  ( 8.903108651239925564, -22.82508830966962421, 90.00000000000000000 ) ) ;
#19597=CARTESIAN_POINT ( 'NONE',  ( -24.25955693048148731, -12.95188430978291905, 4.357489519555787005 ) ) ;
#19598=CARTESIAN_POINT ( 'NONE',  ( 0.6750190879921618148, -27.49190635773182834, 224.1195089973785741 ) ) ;
#19605=CARTESIAN_POINT ( 'NONE',  ( 23.52368442168704021, -12.84078897116981466, 224.0862411973129724 ) ) ;
#19616=CARTESIAN_POINT ( 'NONE',  ( -24.08956650204662608, -13.26503430059684518, 5.959546603950007793 ) ) ;
#19621=SHAPE_REPRESENTATION ( 'Cradle Body', ( #17722 ), #28868 ) ;
#19625=ADVANCED_FACE ( 'NONE', ( #5016 ), #7222, .F. ) ;
#19632=CARTESIAN_POINT ( 'NONE',  ( -1.421085471519999843E-14, -3.552713678799999608E-15, 187.9396849849999853 ) ) ;
#19641=CARTESIAN_POINT ( 'NONE',  ( 0.000000000000000000, 0.000000000000000000, 193.6055512739999926 ) ) ;
#19643=AXIS2_PLACEMENT_3D ( 'NONE', #4175, #1824, #11412 ) ;
#19646=CARTESIAN_POINT ( 'NONE',  ( 1.100000000000000311, -27.47799119300000470, 225.0964597111326952 ) ) ;
#19648=DIRECTION ( 'NONE',  ( 0.000000000000000000, -0.000000000000000000, 1.000000000000000000 ) ) ;
#19651=EDGE_CURVE ( 'NONE', #15698, #10713, #14685, .T. ) ;
#19659=EDGE_CURVE ( 'NONE', #26174, #25831, #22716, .T. ) ;
#19667=ORIENTED_EDGE ( 'NONE', *, *, #13702, .F. ) ;
#19676=DIRECTION ( 'NONE',  ( 0.000000000000000000, 0.000000000000000000, 1.000000000000000000 ) ) ;
#19689=AXIS2_PLACEMENT_3D ( 'NONE', #28891, #16926, #26535 ) ;
#19694=CIRCLE ( 'NONE', #10146, 3.200000004570001888 ) ;
#19702=ORIENTED_EDGE ( 'NONE', *, *, #10698, .T. ) ;
#19705=ORIENTED_EDGE ( 'NONE', *, *, #23945, .T. ) ;
#19706=EDGE_CURVE ( 'NONE', #28783, #21131, #11667, .T. ) ;
#19712=CIRCLE ( 'NONE', #23737, 2.999999999999999556 ) ;
#19713=CARTESIAN_POINT ( 'NONE',  ( 23.81569860410000317, -13.75000000000000000, 3.900000000369999942 ) ) ;
#19717=AXIS2_PLACEMENT_3D ( 'NONE', #8286, #17881, #27486 ) ;
#19724=DIRECTION ( 'NONE',  ( 1.000000000000000000, 0.000000000000000000, 0.000000000000000000 ) ) ;
#19740=VERTEX_POINT ( 'NONE', #1226 ) ;
#19750=CARTESIAN_POINT ( 'NONE',  ( -23.86403265525339634, -13.66628296766671546, 3.900000000001122569 ) ) ;
#19759=CARTESIAN_POINT ( 'NONE',  ( -27.92857142860000152, 3.552713678799999608E-15, 87.93968498540000667 ) ) ;
#19764=CARTESIAN_POINT ( 'NONE',  ( 0.000000000000000000, 0.000000000000000000, 42.06031501460000044 ) ) ;
#19768=CARTESIAN_POINT ( 'NONE',  ( 0.8790546033401771542, -27.48597397634632955, 4.334666192900195725 ) ) ;
#19772=CIRCLE ( 'NONE', #22769, 28.50000000000000000 ) ;
#19773=EDGE_CURVE ( 'NONE', #16461, #11358, #17275, .T. ) ;
#19774=CARTESIAN_POINT ( 'NONE',  ( -9.339631244007748023, -25.12005762863060454, 25.40686791475853568 ) ) ;
#19781=VERTEX_POINT ( 'NONE', #10205 ) ;
#19785=EDGE_CURVE ( 'NONE', #4261, #6141, #17430, .T. ) ;
#19786=ORIENTED_EDGE ( 'NONE', *, *, #24765, .T. ) ;
#19787=CIRCLE ( 'NONE', #14754, 28.50000000000000000 ) ;
#19803=CARTESIAN_POINT ( 'NONE',  ( 26.80000000069999899, -3.281945028320000125E-15, 18.39142920540000148 ) ) ;
#19805=ADVANCED_FACE ( 'NONE', ( #15381 ), #7636, .F. ) ;
#19808=CARTESIAN_POINT ( 'NONE',  ( -26.80000000069999899, 3.281945028329999726E-15, 142.8898184869999852 ) ) ;
#19814=CARTESIAN_POINT ( 'NONE',  ( 4.421808970600630495, -26.43392618132180871, 20.40072977778958219 ) ) ;
#19816=AXIS2_PLACEMENT_3D ( 'NONE', #19641, #10199, #24206 ) ;
#19818=VERTEX_POINT ( 'NONE', #7672 ) ;
#19832=CARTESIAN_POINT ( 'NONE',  ( -2.664535259099999568E-14, -26.80000000000000071, 115.0000000000000000 ) ) ;
#19834=CARTESIAN_POINT ( 'NONE',  ( -3.552713678799999608E-15, 0.000000000000000000, 93.21714158839999698 ) ) ;
#19836=DIRECTION ( 'NONE',  ( 0.000000000000000000, 0.000000000000000000, 1.000000000000000000 ) ) ;
#19842=AXIS2_PLACEMENT_3D ( 'NONE', #4286, #21271, #1613 ) ;
#19847=CARTESIAN_POINT ( 'NONE',  ( -23.81569860410000317, -13.75000000000000000, 3.900000000369999942 ) ) ;
#19863=ORIENTED_EDGE ( 'NONE', *, *, #12289, .F. ) ;
#19865=AXIS2_PLACEMENT_3D ( 'NONE', #15621, #28206, #23187 ) ;
#19872=VERTEX_POINT ( 'NONE', #20733 ) ;
#19879=CARTESIAN_POINT ( 'NONE',  ( -21.30888436558563370, -16.34772642260384146, 193.2171415879999756 ) ) ;
#19882=B_SPLINE_CURVE_WITH_KNOTS ( 'NONE', 3,
 ( #18374, #13492, #23109, #18526, #20900, #25777, #1548, #30499, #27969, #11453 ),
 .UNSPECIFIED., .F., .F.,
 ( 4, 2, 2, 2, 4 ),
 ( 0.000000000000000000, 0.2500000000000000000, 0.5000000000000000000, 0.7500000000000000000, 1.000000000000000000 ),
 .UNSPECIFIED. ) ;
#19896=ORIENTED_EDGE ( 'NONE', *, *, #1563, .T. ) ;
#19915=FACE_OUTER_BOUND ( 'NONE', #7001, .T. ) ;
#19926=CARTESIAN_POINT ( 'NONE',  ( -25.04491701902130174, -9.543388590360494916, 93.21714158838632613 ) ) ;
#19933=ORIENTED_EDGE ( 'NONE', *, *, #8806, .F. ) ;
#19935=EDGE_LOOP ( 'NONE', ( #16216, #29472, #14727, #2825 ) ) ;
#19937=DIRECTION ( 'NONE',  ( 0.000000000000000000, 0.000000000000000000, 1.000000000000000000 ) ) ;
#19942=DIRECTION ( 'NONE',  ( 1.000000000000000000, -1.224606353819999829E-16, 0.000000000000000000 ) ) ;
#19959=CARTESIAN_POINT ( 'NONE',  ( 24.25955693124982915, -12.95188430838311078, 225.6425104787478517 ) ) ;
#19980=DIRECTION ( 'NONE',  ( -1.000000000000000000, 1.224606353819999829E-16, 0.000000000000000000 ) ) ;
#19985=FACE_OUTER_BOUND ( 'NONE', #1038, .T. ) ;
#19990=AXIS2_PLACEMENT_3D ( 'NONE', #4775, #17029, #7432 ) ;
#19991=EDGE_CURVE ( 'NONE', #30789, #2523, #27667, .T. ) ;
#19995=CIRCLE ( 'NONE', #6426, 4.000000004070001225 ) ;
#19998=DIRECTION ( 'NONE',  ( 1.224606353819999829E-16, 1.000000000000000000, 0.000000000000000000 ) ) ;
#20003=ORIENTED_EDGE ( 'NONE', *, *, #8806, .T. ) ;
#20017=AXIS2_PLACEMENT_3D ( 'NONE', #27218, #4931, #20140 ) ;
#20018=CARTESIAN_POINT ( 'NONE',  ( 6.112033042629987811, -26.81582465834874540, 208.9768085133924558 ) ) ;
#20028=CARTESIAN_POINT ( 'NONE',  ( -23.36339467993373376, -14.50559736726076387, 224.3250316505409501 ) ) ;
#20040=AXIS2_PLACEMENT_3D ( 'NONE', #16007, #6086, #8284 ) ;
#20049=ADVANCED_FACE ( 'NONE', ( #29355 ), #24671, .F. ) ;
#20055=EDGE_CURVE ( 'NONE', #27919, #23263, #22600, .T. ) ;
#20057=ADVANCED_BREP_SHAPE_REPRESENTATION ( '', ( #688, #17722 ), #28868 ) ;
#20060=ADVANCED_FACE ( 'NONE', ( #589 ), #2061, .T. ) ;
#20063=UNCERTAINTY_MEASURE_WITH_UNIT (LENGTH_MEASURE( 1.000000000000000082E-05 ), #5410, 'distance_accuracy_value', 'NONE');
#20077=CARTESIAN_POINT ( 'NONE',  ( 22.65536946399887341, -14.31703147657543695, 224.7121835352572532 ) ) ;
#20078=ORIENTED_EDGE ( 'NONE', *, *, #6373, .F. ) ;
#20080=CARTESIAN_POINT ( 'NONE',  ( 27.50000000000000000, -3.367667472999999580E-15, 211.8027756369999679 ) ) ;
#20081=CARTESIAN_POINT ( 'NONE',  ( -26.93395403039999891, 3.298349123919999922E-15, 87.75675929320000535 ) ) ;
#20085=AXIS2_PLACEMENT_3D ( 'NONE', #15517, #19937, #25122 ) ;
#20086=AXIS2_PLACEMENT_3D ( 'NONE', #26597, #26746, #21889 ) ;
#20111=CARTESIAN_POINT ( 'NONE',  ( -23.73992238019999945, -12.43607998449999918, 225.0000000000000000 ) ) ;
#20112=CARTESIAN_POINT ( 'NONE',  ( 24.08872333959831380, -11.87645233066226069, 86.78285841130833944 ) ) ;
#20140=DIRECTION ( 'NONE',  ( 0.3633921898465273803, -0.9316362575375355393, 0.000000000000000000 ) ) ;
#20143=DIRECTION ( 'NONE',  ( 0.000000000000000000, 0.000000000000000000, 1.000000000000000000 ) ) ;
#20144=ADVANCED_FACE ( 'NONE', ( #10332 ), #7948, .T. ) ;
#20151=CARTESIAN_POINT ( 'NONE',  ( 18.95046173579999760, -18.95046173579999760, 115.0000000000000000 ) ) ;
#20155=DIRECTION ( 'NONE',  ( -1.000000000000000000, 5.665498452320000818E-16, 0.000000000000000000 ) ) ;
#20160=ORIENTED_EDGE ( 'NONE', *, *, #28825, .F. ) ;
#20161=DIRECTION ( 'NONE',  ( 0.000000000000000000, 0.000000000000000000, -1.000000000000000000 ) ) ;
#20164=B_SPLINE_CURVE_WITH_KNOTS ( 'NONE', 5,
 ( #15552, #14953, #25161, #24550, #12579, #22186 ),
 .UNSPECIFIED., .F., .F.,
 ( 6, 6 ),
 ( 0.000000000000000000, 2.300779731210000012 ),
 .UNSPECIFIED. ) ;
#20172=EDGE_CURVE ( 'NONE', #22078, #8738, #19148, .T. ) ;
#20195=VECTOR ( 'NONE', #20857, 1000.000000000000114 ) ;
#20196=FILL_AREA_STYLE ('',( #3353 ) ) ;
#20212=AXIS2_PLACEMENT_3D ( 'NONE', #29734, #20143, #5969 ) ;
#20213=EDGE_LOOP ( 'NONE', ( #25477, #3319, #17177, #15089, #3618 ) ) ;
#20220=EDGE_CURVE ( 'NONE', #24391, #8508, #13623, .T. ) ;
#20225=CARTESIAN_POINT ( 'NONE',  ( -24.90462872294776986, -9.900530325344881533, 93.21714158839293418 ) ) ;
#20227=ADVANCED_FACE ( 'NONE', ( #18642 ), #28558, .F. ) ;
#20229=DIRECTION ( 'NONE',  ( 0.000000000000000000, 0.000000000000000000, 1.000000000000000000 ) ) ;
#20231=VECTOR ( 'NONE', #21315, 1000.000000000000000 ) ;
#20237=ORIENTED_EDGE ( 'NONE', *, *, #4777, .F. ) ;
#20246=CARTESIAN_POINT ( 'NONE',  ( 27.54391550559999757, -3.373045393719999713E-15, 137.0437466829999948 ) ) ;
#20248=CARTESIAN_POINT ( 'NONE',  ( 23.52681767382016531, -12.83507605025694964, 4.090187774658970987 ) ) ;
#20253=CARTESIAN_POINT ( 'NONE',  ( -27.50000000000000000, 3.367667473009999970E-15, 186.3944487260000074 ) ) ;
#20262=B_SPLINE_CURVE_WITH_KNOTS ( 'NONE', 3,
 ( #1806, #11395, #27596, #17984, #4000, #16262, #25880, #3678, #20840, #6511, #30276, #28067, #6037, #13751 ),
 .UNSPECIFIED., .F., .F.,
 ( 4, 2, 2, 2, 2, 2, 4 ),
 ( 0.000000000000000000, 0.2500000000000006106, 0.3750000000000021094, 0.4375000000000021649, 0.5000000000000023315, 0.7500000000000011102, 1.000000000000000000 ),
 .UNSPECIFIED. ) ;
#20263=CARTESIAN_POINT ( 'NONE',  ( 8.964607010186844249, -25.25702356185616182, 24.41994893493238905 ) ) ;
#20271=ORIENTED_EDGE ( 'NONE', *, *, #3517, .F. ) ;
#20275=ORIENTED_EDGE ( 'NONE', *, *, #25652, .F. ) ;
#20280=CARTESIAN_POINT ( 'NONE',  ( -0.9245300002449383658, -27.48475604047732190, 4.402548359813233780 ) ) ;
#20290=AXIS2_PLACEMENT_3D ( 'NONE', #25183, #25032, #10560 ) ;
#20293=CIRCLE ( 'NONE', #24325, 27.92857142820000149 ) ;
#20294=CIRCLE ( 'NONE', #20831, 26.80000000000000071 ) ;
#20295=VECTOR ( 'NONE', #21576, 1000.000000000000000 ) ;
#20298=CARTESIAN_POINT ( 'NONE',  ( -27.50000000000000000, 3.367667473009999970E-15, 93.28090191849999258 ) ) ;
#20300=ORIENTED_EDGE ( 'NONE', *, *, #6056, .F. ) ;
#20305=DIRECTION ( 'NONE',  ( 0.000000000000000000, 0.000000000000000000, 1.000000000000000000 ) ) ;
#20308=ORIENTED_EDGE ( 'NONE', *, *, #224, .F. ) ;
#20309=CARTESIAN_POINT ( 'NONE',  ( -2.813083154009999692E-14, -26.79999999949999889, 3.899999999999999911 ) ) ;
#20310=ORIENTED_EDGE ( 'NONE', *, *, #30649, .T. ) ;
#20312=EDGE_LOOP ( 'NONE', ( #20525, #3236, #28639, #10739, #26821, #27017, #26545, #30698, #22990, #24228 ) ) ;
#20314=AXIS2_PLACEMENT_3D ( 'NONE', #16511, #4092, #11334 ) ;
#20322=CIRCLE ( 'NONE', #19842, 27.23548387100000312 ) ;
#20324=CARTESIAN_POINT ( 'NONE',  ( 9.993285220779432265, -25.61999708228224648, 202.5328830256821391 ) ) ;
#20331=DIRECTION ( 'NONE',  ( -1.000000000000000000, 0.000000000000000000, 0.000000000000000000 ) ) ;
#20334=CARTESIAN_POINT ( 'NONE',  ( -2.947640775130000104E-14, -27.50000000000000000, 115.0000000000000000 ) ) ;
#20337=DIRECTION ( 'NONE',  ( 1.000000000000000000, -1.224606353819999829E-16, 0.000000000000000000 ) ) ;
#20342=ORIENTED_EDGE ( 'NONE', *, *, #5098, .T. ) ;
#20367=VERTEX_POINT ( 'NONE', #87 ) ;
#20369=CARTESIAN_POINT ( 'NONE',  ( 0.1474953932389658495, -26.80000000000002203, 6.100000000000008527 ) ) ;
#20371=DIRECTION ( 'NONE',  ( 0.000000000000000000, 0.000000000000000000, -1.000000000000000000 ) ) ;
#20374=FACE_OUTER_BOUND ( 'NONE', #30445, .T. ) ;
#20375=CYLINDRICAL_SURFACE ( 'NONE', #3745, 26.80000000000002203 ) ;
#20377=CARTESIAN_POINT ( 'NONE',  ( -27.50000000000000000, 3.367667473009999970E-15, 230.0000000000000000 ) ) ;
#20382=VERTEX_POINT ( 'NONE', #9666 ) ;
#20390=EDGE_CURVE ( 'NONE', #22757, #31042, #26423, .T. ) ;
#20405=DIRECTION ( 'NONE',  ( 0.000000000000000000, 0.000000000000000000, 1.000000000000000000 ) ) ;
#20408=DIRECTION ( 'NONE',  ( 0.000000000000000000, 0.000000000000000000, -1.000000000000000000 ) ) ;
#20417=EDGE_CURVE ( 'NONE', #11023, #16979, #24912, .T. ) ;
#20418=CARTESIAN_POINT ( 'NONE',  ( 4.433903769297828035, -26.43189459824146326, 209.5952735306987336 ) ) ;
#20420=CARTESIAN_POINT ( 'NONE',  ( -24.76171951330573862, -10.25169584067250383, 43.21714158839993303 ) ) ;
#20421=CARTESIAN_POINT ( 'NONE',  ( 24.13062658790415682, -13.18986347251061808, 225.9130852754918806 ) ) ;
#20433=DIRECTION ( 'NONE',  ( 0.000000000000000000, 0.000000000000000000, 1.000000000000000000 ) ) ;
#20437=CARTESIAN_POINT ( 'NONE',  ( -1.100000000000000311, -27.47799119229999931, 4.902983112562558254 ) ) ;
#20468=VERTEX_POINT ( 'NONE', #2385 ) ;
#20470=EDGE_CURVE ( 'NONE', #21131, #27919, #1568, .T. ) ;
#20471=CARTESIAN_POINT ( 'NONE',  ( -27.92857142909999979, 3.420150602519999655E-15, 142.0603150149999863 ) ) ;
#20478=CARTESIAN_POINT ( 'NONE',  ( 8.095177325567849635, -26.28419651245282651, 207.3284286765387208 ) ) ;
#20479=CARTESIAN_POINT ( 'NONE',  ( 23.73992238019999945, -12.43607998449999918, 5.000000000000000000 ) ) ;
#20481=ORIENTED_EDGE ( 'NONE', *, *, #16011, .F. ) ;
#20485=CARTESIAN_POINT ( 'NONE',  ( -8.414407093329968390, -26.18160851622837981, 206.9056236797458155 ) ) ;
#20486=CIRCLE ( 'NONE', #13455, 27.50000000000000000 ) ;
#20487=CARTESIAN_POINT ( 'NONE',  ( -27.50000000000000000, 3.552713678799999608E-15, 93.60555127549999099 ) ) ;
#20490=CARTESIAN_POINT ( 'NONE',  ( 23.81569860410000317, -13.75000000000000000, 223.8999999999999773 ) ) ;
#20493=DIRECTION ( 'NONE',  ( -0.7071067811865475727, 0.7071067811865475727, 0.000000000000000000 ) ) ;
#20494=CARTESIAN_POINT ( 'NONE',  ( -27.50000000000000000, 3.367667473009999970E-15, 86.39444872359999295 ) ) ;
#20495=EDGE_LOOP ( 'NONE', ( #30235, #1947, #1794, #8233 ) ) ;
#20497=CARTESIAN_POINT ( 'NONE',  ( 9.897162125403639266, -25.37356426577972002, 91.66046017469999185 ) ) ;
#20509=AXIS2_PLACEMENT_3D ( 'NONE', #1442, #18577, #16372 ) ;
#20510=DIRECTION ( 'NONE',  ( -0.9316362575375349842, 0.3633921898465292122, -0.000000000000000000 ) ) ;
#20511=ORIENTED_EDGE ( 'NONE', *, *, #8887, .F. ) ;
#20525=ORIENTED_EDGE ( 'NONE', *, *, #7267, .F. ) ;
#20526=DIRECTION ( 'NONE',  ( -0.000000000000000000, -0.000000000000000000, -1.000000000000000000 ) ) ;
#20529=CARTESIAN_POINT ( 'NONE',  ( 7.105427357599999217E-15, 8.881784196999999612E-15, 43.60555127550000520 ) ) ;
#20530=CARTESIAN_POINT ( 'NONE',  ( 9.993285220779439371, -25.61999708228226069, 27.99999999999999645 ) ) ;
#20546=LINE ( 'NONE', #15361, #17695 ) ;
#20569=DIRECTION ( 'NONE',  ( -0.9316362575375349842, 0.3633921898465292122, -0.000000000000000000 ) ) ;
#20570=B_SPLINE_CURVE_WITH_KNOTS ( 'NONE', 3,
 ( #7907, #10440, #17958, #22558, #8363, #15771, #8059, #12949, #1003, #29935 ),
 .UNSPECIFIED., .F., .F.,
 ( 4, 2, 2, 2, 4 ),
 ( 0.000000000000000000, 0.2500000000000000000, 0.5000000000000000000, 0.7500000000000000000, 1.000000000000000000 ),
 .UNSPECIFIED. ) ;
#20574=TOROIDAL_SURFACE ( 'NONE', #19077, 30.50000000000000000, 3.000000000000000000 ) ;
#20575=CARTESIAN_POINT ( 'NONE',  ( 9.993285220779439371, -25.61999708228226069, 202.0000000000000000 ) ) ;
#20581=VERTEX_POINT ( 'NONE', #17002 ) ;
#20586=ORIENTED_EDGE ( 'NONE', *, *, #14582, .T. ) ;
#20592=EDGE_CURVE ( 'NONE', #8194, #12035, #27137, .T. ) ;
#20599=DIRECTION ( 'NONE',  ( 1.000000000000000000, -1.224606353819998843E-16, 0.000000000000000000 ) ) ;
#20600=EDGE_CURVE ( 'NONE', #29682, #16141, #5082, .T. ) ;
#20604=CARTESIAN_POINT ( 'NONE',  ( -1.100000000000000533, -26.77741585740000829, 5.097059005707468060 ) ) ;
#20609=CIRCLE ( 'NONE', #5535, 26.80000000000000071 ) ;
#20610=DIRECTION ( 'NONE',  ( 0.9316362575375356503, 0.3633921898465274913, 0.000000000000000000 ) ) ;
#20617=CARTESIAN_POINT ( 'NONE',  ( -23.09961856954875614, -13.58841269839368771, 223.9123094310619422 ) ) ;
#20619=CARTESIAN_POINT ( 'NONE',  ( 0.8178294365284820566, -26.78758452998259187, 4.262774516068433606 ) ) ;
#20621=TOROIDAL_SURFACE ( 'NONE', #3035, 24.50000000000000000, 3.200000000000000178 ) ;
#20622=CARTESIAN_POINT ( 'NONE',  ( -4.933588760076017543, -27.05494253741617428, 20.48841368488172776 ) ) ;
#20623=ORIENTED_EDGE ( 'NONE', *, *, #23789, .T. ) ;
#20624=EDGE_CURVE ( 'NONE', #17664, #23969, #4588, .T. ) ;
#20638=CARTESIAN_POINT ( 'NONE',  ( 23.68823177919582434, -12.53428999841347746, 5.486606152542477410 ) ) ;
#20643=CYLINDRICAL_SURFACE ( 'NONE', #17348, 26.80000000000002203 ) ;
#20651=CARTESIAN_POINT ( 'NONE',  ( 24.28117756992811493, -12.91036561250576220, 224.4438356455087273 ) ) ;
#20656=VERTEX_POINT ( 'NONE', #15925 ) ;
#20668=ORIENTED_EDGE ( 'NONE', *, *, #6189, .T. ) ;
#20674=LINE ( 'NONE', #15948, #17469 ) ;
#20675=DIRECTION ( 'NONE',  ( 0.9316362575375356503, 0.3633921898465274913, 0.000000000000000000 ) ) ;
#20682=VERTEX_POINT ( 'NONE', #25535 ) ;
#20688=LINE ( 'NONE', #10772, #8632 ) ;
#20689=DIRECTION ( 'NONE',  ( 0.000000000000000000, 0.000000000000000000, 1.000000000000000000 ) ) ;
#20717=( NAMED_UNIT ( * ) SI_UNIT ( $, .STERADIAN. ) SOLID_ANGLE_UNIT ( ) );
#20725=DIRECTION ( 'NONE',  ( 1.224606353819999829E-16, 1.000000000000000000, 0.000000000000000000 ) ) ;
#20727=DIRECTION ( 'NONE',  ( 1.000000000000000000, 0.000000000000000000, 0.000000000000000000 ) ) ;
#20728=B_SPLINE_CURVE_WITH_KNOTS ( 'NONE', 3,
 ( #21803, #16759, #26377, #9998, #4820, #19598, #29177, #16455, #12822, #7779 ),
 .UNSPECIFIED., .F., .F.,
 ( 4, 2, 2, 2, 4 ),
 ( 0.000000000000000000, 0.2500000000000000000, 0.5000000000000000000, 0.7500000000000000000, 1.000000000000000000 ),
 .UNSPECIFIED. ) ;
#20733=CARTESIAN_POINT ( 'NONE',  ( -27.23548387060000309, 8.881784196999999612E-15, 191.6604601750000256 ) ) ;
#20740=ORIENTED_EDGE ( 'NONE', *, *, #29031, .F. ) ;
#20745=VERTEX_POINT ( 'NONE', #20962 ) ;
#20747=ORIENTED_EDGE ( 'NONE', *, *, #21123, .T. ) ;
#20749=DIRECTION ( 'NONE',  ( 1.000000000000000000, 0.000000000000000000, 0.000000000000000000 ) ) ;
#20751=DIRECTION ( 'NONE',  ( 0.000000000000000000, 0.000000000000000000, 1.000000000000000000 ) ) ;
#20761=DIRECTION ( 'NONE',  ( 1.000000000000000000, 0.000000000000000000, 0.000000000000000000 ) ) ;
#20766=B_SPLINE_CURVE_WITH_KNOTS ( 'NONE', 5,
 ( #7600, #19101, #228, #5085, #14694, #24283 ),
 .UNSPECIFIED., .F., .F.,
 ( 6, 6 ),
 ( 0.000000000000000000, 2.319814892410000162 ),
 .UNSPECIFIED. ) ;
#20770=EDGE_CURVE ( 'NONE', #9833, #28814, #3842, .T. ) ;
#20771=VECTOR ( 'NONE', #21088, 1000.000000000000114 ) ;
#20779=AXIS2_PLACEMENT_3D ( 'NONE', #29261, #8156, #498 ) ;
#20781=FACE_OUTER_BOUND ( 'NONE', #2422, .T. ) ;
#20784=EDGE_CURVE ( 'NONE', #21744, #29682, #189, .T. ) ;
#20786=ORIENTED_EDGE ( 'NONE', *, *, #16433, .T. ) ;
#20788=ORIENTED_EDGE ( 'NONE', *, *, #17444, .F. ) ;
#20795=CARTESIAN_POINT ( 'NONE',  ( -26.62824275575433930, -3.502825096380762115, 0.000000000000000000 ) ) ;
#20803=CARTESIAN_POINT ( 'NONE',  ( -9.993285220779418054, -25.61999708228225714, 202.5329093469738666 ) ) ;
#20806=CARTESIAN_POINT ( 'NONE',  ( 0.000000000000000000, 0.000000000000000000, 210.0000000000000284 ) ) ;
#20825=AXIS2_PLACEMENT_3D ( 'NONE', #8404, #28238, #25740 ) ;
#20826=ORIENTED_EDGE ( 'NONE', *, *, #9506, .F. ) ;
#20829=AXIS2_PLACEMENT_3D ( 'NONE', #24560, #29267, #20727 ) ;
#20831=AXIS2_PLACEMENT_3D ( 'NONE', #14269, #4827, #2157 ) ;
#20834=CARTESIAN_POINT ( 'NONE',  ( 3.466821295769682159E-14, -2.890242878314739659E-13, 27.99999999999999645 ) ) ;
#20837=CARTESIAN_POINT ( 'NONE',  ( -2.664535259099999568E-14, -26.80000000000000071, 223.8999999999999773 ) ) ;
#20840=CARTESIAN_POINT ( 'NONE',  ( -23.60764285266575868, -12.68553248570766456, 5.737227008375342052 ) ) ;
#20843=CARTESIAN_POINT ( 'NONE',  ( -22.63992238019999803, -14.34133587289999845, 225.0000000000000000 ) ) ;
#20850=CARTESIAN_POINT ( 'NONE',  ( 0.000000000000000000, 3.552713678799999608E-15, 193.2171415880000040 ) ) ;
#20854=CIRCLE ( 'NONE', #25890, 27.50000000000000000 ) ;
#20856=VECTOR ( 'NONE', #16393, 1000.000000000000000 ) ;
#20857=DIRECTION ( 'NONE',  ( 0.8660254037843289066, -0.5000000000001899592, 0.000000000000000000 ) ) ;
#20875=CIRCLE ( 'NONE', #19865, 27.92857142860000152 ) ;
#20877=DIRECTION ( 'NONE',  ( -0.3633921898465292122, -0.9316362575375349842, 0.000000000000000000 ) ) ;
#20878=VERTEX_POINT ( 'NONE', #19847 ) ;
#20880=VERTEX_POINT ( 'NONE', #29428 ) ;
#20883=CARTESIAN_POINT ( 'NONE',  ( 27.50000000000000000, -3.367667472999999580E-15, 43.60555127639999995 ) ) ;
#20890=ORIENTED_EDGE ( 'NONE', *, *, #15081, .F. ) ;
#20892=CARTESIAN_POINT ( 'NONE',  ( -27.50000000000000000, 1.776356839399999804E-15, 43.60555127550000520 ) ) ;
#20900=CARTESIAN_POINT ( 'NONE',  ( -23.34643930348873653, -14.53345043297602679, 5.642510478632145166 ) ) ;
#20912=DIRECTION ( 'NONE',  ( 0.000000000000000000, 0.000000000000000000, -1.000000000000000000 ) ) ;
#20917=DIRECTION ( 'NONE',  ( 1.000000000000000000, 0.000000000000000000, 0.000000000000000000 ) ) ;
#20922=DIRECTION ( 'NONE',  ( 0.000000000000000000, 0.000000000000000000, 1.000000000000000000 ) ) ;
#20925=CARTESIAN_POINT ( 'NONE',  ( -0.9876156946213142662, -26.78228253924901026, 5.491373163700855820 ) ) ;
#20930=CARTESIAN_POINT ( 'NONE',  ( -23.73988890810277752, -12.43614388128984594, 4.854121447335470130 ) ) ;
#20932=EDGE_CURVE ( 'NONE', #19872, #19818, #8596, .T. ) ;
#20933=DIRECTION ( 'NONE',  ( 0.000000000000000000, 0.000000000000000000, -1.000000000000000000 ) ) ;
#20942=ORIENTED_EDGE ( 'NONE', *, *, #17326, .T. ) ;
#20954=EDGE_CURVE ( 'NONE', #24391, #22821, #11132, .T. ) ;
#20960=CARTESIAN_POINT ( 'NONE',  ( 23.53911279562209202, -12.81252279912947323, 225.8816713824184035 ) ) ;
#20962=CARTESIAN_POINT ( 'NONE',  ( 23.20948082139999968, -13.40000000000000036, 3.900000000369999942 ) ) ;
#20966=DIRECTION ( 'NONE',  ( 0.000000000000000000, 0.000000000000000000, 1.000000000000000000 ) ) ;
#20971=ORIENTED_EDGE ( 'NONE', *, *, #3987, .T. ) ;
#20983=DIRECTION ( 'NONE',  ( -1.000000000000000000, 5.665498452320000818E-16, 0.000000000000000000 ) ) ;
#20991=TOROIDAL_SURFACE ( 'NONE', #26511, 24.50000000000000000, 4.000000000000000000 ) ;
#20999=DIRECTION ( 'NONE',  ( -1.000000000000000000, 5.665498452320000818E-16, 0.000000000000000000 ) ) ;
#21011=AXIS2_PLACEMENT_3D ( 'NONE', #22419, #10604, #5871 ) ;
#21033=CARTESIAN_POINT ( 'NONE',  ( 9.738910687886868089, -24.96785170200598358, 115.0000000000000000 ) ) ;
#21039=CIRCLE ( 'NONE', #25049, 4.000000004070001225 ) ;
#21044=CARTESIAN_POINT ( 'NONE',  ( 9.993285220779506872, -25.61999708228222872, 43.60555127639999995 ) ) ;
#21049=CARTESIAN_POINT ( 'NONE',  ( -0.8805184773353784689, -27.48609199508887002, 225.6749683491974565 ) ) ;
#21052=CIRCLE ( 'NONE', #19019, 3.200000004570001888 ) ;
#21057=CARTESIAN_POINT ( 'NONE',  ( -24.25955693044071637, -12.95188430987226802, 224.3574895194784347 ) ) ;
#21061=TOROIDAL_SURFACE ( 'NONE', #20040, 24.50000000000000000, 3.200000000000000178 ) ;
#21062=EDGE_CURVE ( 'NONE', #25858, #5609, #15144, .T. ) ;
#21067=ORIENTED_EDGE ( 'NONE', *, *, #11511, .T. ) ;
#21069=ORIENTED_EDGE ( 'NONE', *, *, #2318, .T. ) ;
#21071=CARTESIAN_POINT ( 'NONE',  ( 1.065814103639999922E-14, 0.000000000000000000, 38.33953982530000104 ) ) ;
#21084=CIRCLE ( 'NONE', #29608, 3.000000000000001332 ) ;
#21088=DIRECTION ( 'NONE',  ( -0.8660254037843289066, -0.5000000000001899592, 0.000000000000000000 ) ) ;
#21097=CARTESIAN_POINT ( 'NONE',  ( 0.9242227292564770824, -26.78436817533707526, 4.402069900664497659 ) ) ;
#21098=VERTEX_POINT ( 'NONE', #470 ) ;
#21107=DIRECTION ( 'NONE',  ( 1.000000000000000000, 0.000000000000000000, 0.000000000000000000 ) ) ;
#21122=CARTESIAN_POINT ( 'NONE',  ( -26.80000000069999899, 3.281945028329999726E-15, 18.39142920540000148 ) ) ;
#21123=EDGE_CURVE ( 'NONE', #22430, #7318, #1588, .T. ) ;
#21125=CARTESIAN_POINT ( 'NONE',  ( -27.50000000000000000, 3.367667473009999970E-15, 65.00000000000000000 ) ) ;
#21131=VERTEX_POINT ( 'NONE', #7064 ) ;
#21132=DIRECTION ( 'NONE',  ( 0.3633921898465292122, 0.9316362575375348731, -6.938893903907226800E-15 ) ) ;
#21137=VERTEX_POINT ( 'NONE', #5244 ) ;
#21138=ORIENTED_EDGE ( 'NONE', *, *, #20954, .F. ) ;
#21149=ORIENTED_EDGE ( 'NONE', *, *, #255, .T. ) ;
#21151=AXIS2_PLACEMENT_3D ( 'NONE', #8567, #6378, #15824 ) ;
#21153=CARTESIAN_POINT ( 'NONE',  ( 27.92857142909999979, -3.420150602509999660E-15, 137.9396849850000137 ) ) ;
#21160=CARTESIAN_POINT ( 'NONE',  ( 8.986416953306171962, -25.99194954040538619, 23.96300465906694299 ) ) ;
#21162=DIRECTION ( 'NONE',  ( 0.000000000000000000, 0.000000000000000000, -1.000000000000000000 ) ) ;
#21164=DIRECTION ( 'NONE',  ( -0.000000000000000000, -0.000000000000000000, -1.000000000000000000 ) ) ;
#21165=ORIENTED_EDGE ( 'NONE', *, *, #21170, .F. ) ;
#21169=EDGE_CURVE ( 'NONE', #17667, #22455, #13989, .T. ) ;
#21170=EDGE_CURVE ( 'NONE', #18252, #3758, #27485, .T. ) ;
#21174=CARTESIAN_POINT ( 'NONE',  ( 27.63177356690000153, -3.383804547719999749E-15, 37.36052363810000543 ) ) ;
#21179=EDGE_CURVE ( 'NONE', #7809, #27823, #8330, .T. ) ;
#21182=ORIENTED_EDGE ( 'NONE', *, *, #9018, .T. ) ;
#21188=CARTESIAN_POINT ( 'NONE',  ( 26.93395387800000051, -3.298349105250000085E-15, 42.24324102359999955 ) ) ;
#21191=DIRECTION ( 'NONE',  ( 0.000000000000000000, -1.000000000000000000, 0.000000000000000000 ) ) ;
#21195=CIRCLE ( 'NONE', #30765, 27.92857142860000152 ) ;
#21206=CARTESIAN_POINT ( 'NONE',  ( -0.9131176269203642448, -27.48533474125000708, 224.3574895203637141 ) ) ;
#21211=VECTOR ( 'NONE', #29232, 1000.000000000000000 ) ;
#21219=CARTESIAN_POINT ( 'NONE',  ( 1.065814103639999922E-14, 0.000000000000000000, 36.78285841159999592 ) ) ;
#21222=DIRECTION ( 'NONE',  ( 0.000000000000000000, 0.000000000000000000, 1.000000000000000000 ) ) ;
#21242=CARTESIAN_POINT ( 'NONE',  ( 27.50000000000000000, 1.776356839399999804E-15, 186.3944487249999895 ) ) ;
#21243=ORIENTED_EDGE ( 'NONE', *, *, #17444, .T. ) ;
#21245=CARTESIAN_POINT ( 'NONE',  ( -7.105427357599999217E-15, -7.105427357599999217E-15, 36.78285841159999592 ) ) ;
#21263=CARTESIAN_POINT ( 'NONE',  ( -22.65536398236773508, -14.31703479018443304, 5.288095983115937315 ) ) ;
#21268=CYLINDRICAL_SURFACE ( 'NONE', #2260, 1.099999999999999867 ) ;
#21269=EDGE_CURVE ( 'NONE', #26433, #29406, #15098, .T. ) ;
#21271=DIRECTION ( 'NONE',  ( 0.000000000000000000, 0.000000000000000000, 1.000000000000000000 ) ) ;
#21277=ORIENTED_EDGE ( 'NONE', *, *, #27698, .F. ) ;
#21291=ORIENTED_EDGE ( 'NONE', *, *, #25827, .T. ) ;
#21295=VECTOR ( 'NONE', #20933, 1000.000000000000000 ) ;
#21298=ADVANCED_FACE ( 'NONE', ( #25461 ), #3715, .F. ) ;
#21315=DIRECTION ( 'NONE',  ( -0.000000000000000000, -0.000000000000000000, -1.000000000000000000 ) ) ;
#21322=CIRCLE ( 'NONE', #28828, 4.000000000000001776 ) ;
#21331=CARTESIAN_POINT ( 'NONE',  ( 27.50000000000000000, -3.367667472999999580E-15, 165.0000000000000000 ) ) ;
#21335=CARTESIAN_POINT ( 'NONE',  ( -26.80000000000000071, 9.769962616700000205E-15, 186.7828584120000244 ) ) ;
#21338=VECTOR ( 'NONE', #27385, 1000.000000000000000 ) ;
#21351=DIRECTION ( 'NONE',  ( -0.000000000000000000, -0.000000000000000000, -1.000000000000000000 ) ) ;
#21359=DIRECTION ( 'NONE',  ( -0.9316362575375349842, 0.3633921898465292122, -0.000000000000000000 ) ) ;
#21385=CARTESIAN_POINT ( 'NONE',  ( 27.92857142909999979, -3.420150602509999660E-15, 87.93968498519998889 ) ) ;
#21388=B_SPLINE_CURVE_WITH_KNOTS ( 'NONE', 5,
 ( #26888, #5327, #12561, #625, #19808, #10208 ),
 .UNSPECIFIED., .F., .F.,
 ( 6, 6 ),
 ( -2.319815200109999864, 0.000000000000000000 ),
 .UNSPECIFIED. ) ;
#21389=VERTEX_POINT ( 'NONE', #6560 ) ;
#21391=EDGE_CURVE ( 'NONE', #10044, #14421, #13260, .T. ) ;
#21397=CARTESIAN_POINT ( 'NONE',  ( 27.54391552369999729, -3.373045395939999845E-15, 192.9562530129999800 ) ) ;
#21401=CARTESIAN_POINT ( 'NONE',  ( -23.72659782641452608, -12.46160334549828619, 4.711904017072684248 ) ) ;
#21411=DIRECTION ( 'NONE',  ( -1.000000000000000000, 5.665498452320000818E-16, 0.000000000000000000 ) ) ;
#21418=VERTEX_POINT ( 'NONE', #11905 ) ;
#21430=DIRECTION ( 'NONE',  ( 1.000000000000000000, 0.000000000000000000, 0.000000000000000000 ) ) ;
#21431=CARTESIAN_POINT ( 'NONE',  ( -23.72659769747987824, -12.46160974968614887, 224.7121835346307535 ) ) ;
#21441=ORIENTED_EDGE ( 'NONE', *, *, #23945, .F. ) ;
#21442=CARTESIAN_POINT ( 'NONE',  ( 23.81569860410000317, -13.75000000000000000, 6.099999999630000502 ) ) ;
#21452=ADVANCED_FACE ( 'NONE', ( #26540, #31107 ), #18987, .T. ) ;
#21455=DIRECTION ( 'NONE',  ( 0.000000000000000000, 0.000000000000000000, -1.000000000000000000 ) ) ;
#21456=ORIENTED_EDGE ( 'NONE', *, *, #27913, .T. ) ;
#21459=CARTESIAN_POINT ( 'NONE',  ( -10.35667741062608371, -26.55163333981974816, 40.00000000000000000 ) ) ;
#21481=ORIENTED_EDGE ( 'NONE', *, *, #27081, .F. ) ;
#21485=CIRCLE ( 'NONE', #17449, 4.000000004070001225 ) ;
#21492=DIRECTION ( 'NONE',  ( -0.000000000000000000, -0.000000000000000000, -1.000000000000000000 ) ) ;
#21498=EDGE_LOOP ( 'NONE', ( #3770, #21566, #821, #27626 ) ) ;
#21499=CARTESIAN_POINT ( 'NONE',  ( 0.000000000000000000, 0.000000000000000000, 190.0000000000000000 ) ) ;
#21500=EDGE_CURVE ( 'NONE', #12226, #11846, #12773, .T. ) ;
#21509=CIRCLE ( 'NONE', #13983, 2.999999999999999556 ) ;
#21513=CARTESIAN_POINT ( 'NONE',  ( -26.80000000069999899, 3.281945028329999726E-15, 93.21714158910000947 ) ) ;
#21523=ORIENTED_EDGE ( 'NONE', *, *, #25901, .T. ) ;
#21524=CIRCLE ( 'NONE', #25552, 27.92857142860000152 ) ;
#21526=ORIENTED_EDGE ( 'NONE', *, *, #25745, .F. ) ;
#21527=AXIS2_PLACEMENT_3D ( 'NONE', #27597, #22581, #18316 ) ;
#21554=LINE ( 'NONE', #3, #15313 ) ;
#21566=ORIENTED_EDGE ( 'NONE', *, *, #23999, .T. ) ;
#21576=DIRECTION ( 'NONE',  ( 0.000000000000000000, 0.000000000000000000, 1.000000000000000000 ) ) ;
#21598=DIRECTION ( 'NONE',  ( -0.000000000000000000, -0.000000000000000000, -1.000000000000000000 ) ) ;
#21602=CARTESIAN_POINT ( 'NONE',  ( 23.74292845513278039, -13.87604159523734282, 6.099999999630012937 ) ) ;
#21604=ORIENTED_EDGE ( 'NONE', *, *, #8997, .T. ) ;
#21605=ORIENTED_EDGE ( 'NONE', *, *, #16694, .F. ) ;
#21606=VERTEX_POINT ( 'NONE', #1663 ) ;
#21608=ORIENTED_EDGE ( 'NONE', *, *, #19651, .T. ) ;
#21612=EDGE_LOOP ( 'NONE', ( #20160, #2462, #109, #16408 ) ) ;
#21614=LINE ( 'NONE', #4468, #14169 ) ;
#21623=CARTESIAN_POINT ( 'NONE',  ( -27.50000000000000000, 3.367667473009999970E-15, 143.2809019210000088 ) ) ;
#21632=FACE_OUTER_BOUND ( 'NONE', #19935, .T. ) ;
#21634=EDGE_CURVE ( 'NONE', #27430, #1290, #729, .T. ) ;
#21642=EDGE_LOOP ( 'NONE', ( #11117, #18912, #12845, #1083 ) ) ;
#21649=EDGE_LOOP ( 'NONE', ( #26197, #13658, #14710, #20271 ) ) ;
#21661=CARTESIAN_POINT ( 'NONE',  ( 1.071233845142131713, -26.77863813576653484, 225.2880959822963973 ) ) ;
#21664=DIRECTION ( 'NONE',  ( 1.000000000000000000, 0.000000000000000000, 0.000000000000000000 ) ) ;
#21667=CARTESIAN_POINT ( 'NONE',  ( -1.087555936180296001, -26.77834284442311130, 225.2180515729460240 ) ) ;
#21673=CARTESIAN_POINT ( 'NONE',  ( -18.95046173579999760, -18.95046173579999760, 115.0000000000000000 ) ) ;
#21675=ORIENTED_EDGE ( 'NONE', *, *, #27570, .T. ) ;
#21682=ORIENTED_EDGE ( 'NONE', *, *, #4497, .T. ) ;
#21686=DIRECTION ( 'NONE',  ( 0.000000000000000000, 0.000000000000000000, 1.000000000000000000 ) ) ;
#21693=DIRECTION ( 'NONE',  ( -1.000000000000000000, 5.665498452320000818E-16, 0.000000000000000000 ) ) ;
#21709=AXIS2_PLACEMENT_3D ( 'NONE', #28467, #23761, #16812 ) ;
#21714=CARTESIAN_POINT ( 'NONE',  ( 24.24391315721468487, -12.98049462758916661, 4.325031651118865561 ) ) ;
#21733=CARTESIAN_POINT ( 'NONE',  ( 10.82908725742651512, -27.76276047461856322, 193.2171415880000040 ) ) ;
#21744=VERTEX_POINT ( 'NONE', #28402 ) ;
#21747=CARTESIAN_POINT ( 'NONE',  ( -27.50000000000000000, 3.367667473009999970E-15, 211.8027756369999679 ) ) ;
#21752=CIRCLE ( 'NONE', #6670, 2.999999999999999556 ) ;
#21770=ADVANCED_FACE ( 'NONE', ( #2290 ), #16735, .T. ) ;
#21785=DIRECTION ( 'NONE',  ( 0.000000000000000000, -1.000000000000000000, 0.000000000000000000 ) ) ;
#21792=CIRCLE ( 'NONE', #25820, 3.199999983039998774 ) ;
#21795=EDGE_CURVE ( 'NONE', #7318, #4812, #15812, .T. ) ;
#21797=EDGE_LOOP ( 'NONE', ( #5643, #15018, #20971, #8939 ) ) ;
#21803=CARTESIAN_POINT ( 'NONE',  ( 1.100000000000000089, -27.47799119300000115, 225.0000000000000000 ) ) ;
#21805=CARTESIAN_POINT ( 'NONE',  ( 0.000000000000000000, 0.000000000000000000, 36.39444872359999295 ) ) ;
#21812=CIRCLE ( 'NONE', #17255, 2.999999999999999556 ) ;
#21817=CIRCLE ( 'NONE', #18773, 27.50000000000000000 ) ;
#21819=TOROIDAL_SURFACE ( 'NONE', #13772, 29.80000000000000071, 3.000000000000000000 ) ;
#21822=CARTESIAN_POINT ( 'NONE',  ( -6.394884621839999216E-14, -26.80000000000000071, 226.0999999999999943 ) ) ;
#21828=VERTEX_POINT ( 'NONE', #15013 ) ;
#21841=TOROIDAL_SURFACE ( 'NONE', #9240, 29.80000000000000071, 3.000000000000000000 ) ;
#21845=ORIENTED_EDGE ( 'NONE', *, *, #17326, .F. ) ;
#21851=CARTESIAN_POINT ( 'NONE',  ( 9.738910687886868089, -24.96785170200598358, 186.7828584120000244 ) ) ;
#21856=VERTEX_POINT ( 'NONE', #8062 ) ;
#21861=CARTESIAN_POINT ( 'NONE',  ( 0.9131176273315529945, -27.48533474125000353, 225.6425104791852618 ) ) ;
#21863=VECTOR ( 'NONE', #16627, 1000.000000000000000 ) ;
#21873=LINE ( 'NONE', #19504, #18770 ) ;
#21875=ORIENTED_EDGE ( 'NONE', *, *, #25863, .F. ) ;
#21884=EDGE_LOOP ( 'NONE', ( #27739, #11223, #4130, #27701 ) ) ;
#21889=DIRECTION ( 'NONE',  ( 1.000000000000000000, -1.224606353819999582E-16, 0.000000000000000000 ) ) ;
#21895=CARTESIAN_POINT ( 'NONE',  ( -22.69912944659995446, -14.24746549235085524, 5.486606152533540559 ) ) ;
#21905=CARTESIAN_POINT ( 'NONE',  ( 3.938336462418420059, -27.21777852796476793, 20.19589729288204083 ) ) ;
#21913=CARTESIAN_POINT ( 'NONE',  ( 0.000000000000000000, 0.000000000000000000, 140.0000000000000000 ) ) ;
#21917=DIRECTION ( 'NONE',  ( 0.000000000000000000, 0.000000000000000000, 1.000000000000000000 ) ) ;
#21923=ORIENTED_EDGE ( 'NONE', *, *, #8309, .T. ) ;
#21924=CARTESIAN_POINT ( 'NONE',  ( 26.80000000000000071, 7.105427357599999217E-15, 36.78285841090000474 ) ) ;
#21928=EDGE_LOOP ( 'NONE', ( #16639, #25791, #5104, #24466, #15615 ) ) ;
#21929=DIRECTION ( 'NONE',  ( -0.5000000000001894040, 0.8660254037843291286, 0.000000000000000000 ) ) ;
#21935=CARTESIAN_POINT ( 'NONE',  ( 0.000000000000000000, 0.000000000000000000, 115.0000000000000000 ) ) ;
#21952=ORIENTED_EDGE ( 'NONE', *, *, #17662, .T. ) ;
#21964=CARTESIAN_POINT ( 'NONE',  ( -26.80000000069999899, 3.281945028329999726E-15, 193.2171415869999862 ) ) ;
#21966=ADVANCED_FACE ( 'NONE', ( #17658 ), #24918, .F. ) ;
#21973=CARTESIAN_POINT ( 'NONE',  ( -14.39562240800000126, -9.581487064249998298, 225.0000000000000000 ) ) ;
#21981=AXIS2_PLACEMENT_3D ( 'NONE', #15331, #30116, #3358 ) ;
#21983=TOROIDAL_SURFACE ( 'NONE', #12421, 30.50000000000000000, 3.000000000000000000 ) ;
#21984=CARTESIAN_POINT ( 'NONE',  ( -24.28117756995407106, -12.91036561245694081, 5.556164354347067125 ) ) ;
#21992=B_SPLINE_CURVE_WITH_KNOTS ( 'NONE', 5,
 ( #9505, #28700, #17048, #26649, #7603, #5088 ),
 .UNSPECIFIED., .F., .F.,
 ( 6, 6 ),
 ( 0.000000000000000000, 2.319814960330000009 ),
 .UNSPECIFIED. ) ;
#21994=AXIS2_PLACEMENT_3D ( 'NONE', #27828, #5652, #8465 ) ;
#21995=FACE_OUTER_BOUND ( 'NONE', #9008, .T. ) ;
#22001=CIRCLE ( 'NONE', #5411, 3.200000000000002398 ) ;
#22011=CARTESIAN_POINT ( 'NONE',  ( -7.105427357599999217E-15, 7.105427357599999217E-15, 86.39444872449999480 ) ) ;
#22012=LINE ( 'NONE', #2650, #958 ) ;
#22015=DIRECTION ( 'NONE',  ( 0.000000000000000000, 0.000000000000000000, -1.000000000000000000 ) ) ;
#22019=ADVANCED_FACE ( 'NONE', ( #30422 ), #30397, .T. ) ;
#22021=EDGE_CURVE ( 'NONE', #17004, #11358, #22559, .T. ) ;
#22036=ORIENTED_EDGE ( 'NONE', *, *, #7405, .T. ) ;
#22044=VECTOR ( 'NONE', #6855, 1000.000000000000000 ) ;
#22049=AXIS2_PLACEMENT_3D ( 'NONE', #11805, #28638, #9435 ) ;
#22053=AXIS2_PLACEMENT_3D ( 'NONE', #21499, #11898, #31099 ) ;
#22066=EDGE_LOOP ( 'NONE', ( #11691, #12413, #10600, #30507 ) ) ;
#22070=ORIENTED_EDGE ( 'NONE', *, *, #29448, .F. ) ;
#22071=ORIENTED_EDGE ( 'NONE', *, *, #30225, .T. ) ;
#22077=CARTESIAN_POINT ( 'NONE',  ( -9.993285220779425160, -25.61999708228226069, 186.3944487260000074 ) ) ;
#22078=VERTEX_POINT ( 'NONE', #20497 ) ;
#22086=DIRECTION ( 'NONE',  ( -0.9316362575375349842, 0.3633921898465292122, -0.000000000000000000 ) ) ;
#22091=AXIS2_PLACEMENT_3D ( 'NONE', #16607, #7018, #26375 ) ;
#22093=CARTESIAN_POINT ( 'NONE',  ( 26.93395386830000149, -3.298349104060000254E-15, 192.2432411359999946 ) ) ;
#22105=DIRECTION ( 'NONE',  ( 0.9316362575375356503, 0.3633921898465274913, 0.000000000000000000 ) ) ;
#22109=DIRECTION ( 'NONE',  ( 0.000000000000000000, 0.000000000000000000, 1.000000000000000000 ) ) ;
#22110=AXIS2_PLACEMENT_3D ( 'NONE', #28954, #16528, #26139 ) ;
#22113=CARTESIAN_POINT ( 'NONE',  ( -15.49562240950000103, -7.676231176589999983, 5.000000000000000000 ) ) ;
#22116=DIRECTION ( 'NONE',  ( 1.000000000000000000, 0.000000000000000000, 0.000000000000000000 ) ) ;
#22133=CARTESIAN_POINT ( 'NONE',  ( -8.310304230308167561, -25.47941657935495741, 23.30551580194968153 ) ) ;
#22145=ORIENTED_EDGE ( 'NONE', *, *, #5389, .F. ) ;
#22149=DIRECTION ( 'NONE',  ( 0.000000000000000000, 0.000000000000000000, -1.000000000000000000 ) ) ;
#22163=CARTESIAN_POINT ( 'NONE',  ( 26.62724484483131349, -3.508068424019962883, 86.78285841101670428 ) ) ;
#22171=ORIENTED_EDGE ( 'NONE', *, *, #24267, .T. ) ;
#22174=CARTESIAN_POINT ( 'NONE',  ( 23.81569860410000317, -13.75000000000000000, 3.900000000369999942 ) ) ;
#22176=EDGE_LOOP ( 'NONE', ( #5401, #21952, #4923, #12071 ) ) ;
#22179=AXIS2_PLACEMENT_3D ( 'NONE', #1265, #10864, #30045 ) ;
#22185=CARTESIAN_POINT ( 'NONE',  ( -27.50000000000000000, 3.552713678799999608E-15, 193.6055512750000105 ) ) ;
#22186=CARTESIAN_POINT ( 'NONE',  ( -27.92857142860000152, 3.552713678799999608E-15, 87.93968498540000667 ) ) ;
#22189=DIRECTION ( 'NONE',  ( 1.000000000000000000, 0.000000000000000000, 0.000000000000000000 ) ) ;
#22207=B_SPLINE_CURVE_WITH_KNOTS ( 'NONE', 3,
 ( #24368, #19646, #312, #29081, #21861, #12554, #149, #5013, #29230, #7669 ),
 .UNSPECIFIED., .F., .F.,
 ( 4, 2, 2, 2, 4 ),
 ( 0.000000000000000000, 0.2500000000000000555, 0.5000000000000001110, 0.7500000000000002220, 1.000000000000000000 ),
 .UNSPECIFIED. ) ;
#22214=DIRECTION ( 'NONE',  ( 1.000000000000000000, 0.000000000000000000, 0.000000000000000000 ) ) ;
#22224=FACE_OUTER_BOUND ( 'NONE', #9913, .T. ) ;
#22237=DIRECTION ( 'NONE',  ( 0.000000000000000000, -0.000000000000000000, 1.000000000000000000 ) ) ;
#22238=CARTESIAN_POINT ( 'NONE',  ( 23.24663841809999809, -14.69162354060000020, 225.0000000000000000 ) ) ;
#22246=CIRCLE ( 'NONE', #16704, 27.23548387080000310 ) ;
#22251=EDGE_CURVE ( 'NONE', #12444, #15899, #9421, .T. ) ;
#22252=CARTESIAN_POINT ( 'NONE',  ( 24.25955693097017019, -12.95188430892189402, 5.642510479405106416 ) ) ;
#22253=( NAMED_UNIT ( * ) SI_UNIT ( $, .STERADIAN. ) SOLID_ANGLE_UNIT ( ) );
#22267=CARTESIAN_POINT ( 'NONE',  ( -26.80000000069999899, 3.281945028329999726E-15, 43.21714158909999526 ) ) ;
#22269=ORIENTED_EDGE ( 'NONE', *, *, #23096, .T. ) ;
#22270=CARTESIAN_POINT ( 'NONE',  ( 17.64448518804794830, -20.25643828355104148, 36.78285841153859792 ) ) ;
#22271=CARTESIAN_POINT ( 'NONE',  ( 23.70218820213038313, -12.50899637856321256, 224.5770195905794537 ) ) ;
#22279=CARTESIAN_POINT ( 'NONE',  ( 0.1477568879585779427, -27.50000000000000711, 3.900000000000001688 ) ) ;
#22284=ADVANCED_FACE ( 'NONE', ( #27651 ), #4269, .F. ) ;
#22286=CARTESIAN_POINT ( 'NONE',  ( -25.90058877277587612, -6.940365930346072965, 93.21714158835418118 ) ) ;
#22304=CARTESIAN_POINT ( 'NONE',  ( -26.62724484483129928, -3.508068424019927356, 143.2171415880000040 ) ) ;
#22309=VERTEX_POINT ( 'NONE', #10986 ) ;
#22313=DIRECTION ( 'NONE',  ( 1.000000000000000000, 0.000000000000000000, 0.000000000000000000 ) ) ;
#22320=CARTESIAN_POINT ( 'NONE',  ( 9.544994065185530729, -25.04267878452545304, 203.8307228059247507 ) ) ;
#22326=CIRCLE ( 'NONE', #30894, 3.199999983039998774 ) ;
#22327=CARTESIAN_POINT ( 'NONE',  ( -10.14902473071360411, -26.01926976408356396, 42.06031501460000044 ) ) ;
#22330=ORIENTED_EDGE ( 'NONE', *, *, #8095, .T. ) ;
#22331=CYLINDRICAL_SURFACE ( 'NONE', #23326, 26.80000000000002203 ) ;
#22347=DIRECTION ( 'NONE',  ( 0.000000000000000000, 0.000000000000000000, 1.000000000000000000 ) ) ;
#22363=DIRECTION ( 'NONE',  ( 0.9316362575375356503, 0.3633921898465274913, 0.000000000000000000 ) ) ;
#22365=CARTESIAN_POINT ( 'NONE',  ( -9.738910687886855655, -24.96785170200598714, 115.0000000000000000 ) ) ;
#22373=ORIENTED_EDGE ( 'NONE', *, *, #27076, .F. ) ;
#22385=CARTESIAN_POINT ( 'NONE',  ( 24.49999999470000134, -3.000285566199999922E-15, 40.00000000070000539 ) ) ;
#22390=AXIS2_PLACEMENT_3D ( 'NONE', #839, #12939, #27411 ) ;
#22395=FACE_OUTER_BOUND ( 'NONE', #10880, .T. ) ;
#22397=CARTESIAN_POINT ( 'NONE',  ( 23.67167941920536833, -13.99714051965694850, 226.0719093208177526 ) ) ;
#22411=EDGE_CURVE ( 'NONE', #23813, #15558, #4769, .T. ) ;
#22413=ORIENTED_EDGE ( 'NONE', *, *, #11105, .F. ) ;
#22419=CARTESIAN_POINT ( 'NONE',  ( -10.82908725742657374, -27.76276047461854546, 93.21714158839999698 ) ) ;
#22425=CARTESIAN_POINT ( 'NONE',  ( -27.76135144349999706, 3.399672736839999702E-15, 192.3385858899999903 ) ) ;
#22428=DIRECTION ( 'NONE',  ( 1.000000000000000000, -1.224606353819999829E-16, 0.000000000000000000 ) ) ;
#22430=VERTEX_POINT ( 'NONE', #19151 ) ;
#22436=DIRECTION ( 'NONE',  ( 0.000000000000000000, 0.000000000000000000, -1.000000000000000000 ) ) ;
#22437=CARTESIAN_POINT ( 'NONE',  ( -8.160452367545484975, -25.52912514472581051, 206.9265757142945006 ) ) ;
#22441=VERTEX_POINT ( 'NONE', #9863 ) ;
#22445=CARTESIAN_POINT ( 'NONE',  ( -9.254368700311671248, -25.15168151593200818, 25.15520747740333363 ) ) ;
#22455=VERTEX_POINT ( 'NONE', #28741 ) ;
#22457=EDGE_CURVE ( 'NONE', #8183, #27584, #20854, .T. ) ;
#22462=DIRECTION ( 'NONE',  ( 0.000000000000000000, 0.000000000000000000, 1.000000000000000000 ) ) ;
#22467=EDGE_CURVE ( 'NONE', #19740, #16896, #7278, .T. ) ;
#22472=AXIS2_PLACEMENT_3D ( 'NONE', #15335, #7929, #5730 ) ;
#22473=CARTESIAN_POINT ( 'NONE',  ( 25.43121960300669215, -8.635379644106567554, 86.78285841119168253 ) ) ;
#22474=CARTESIAN_POINT ( 'NONE',  ( -9.738910687886855655, -24.96785170200598714, 115.0000000000000000 ) ) ;
#22477=DIRECTION ( 'NONE',  ( 1.000000000000000000, 0.000000000000000000, 0.000000000000000000 ) ) ;
#22481=ORIENTED_EDGE ( 'NONE', *, *, #18564, .T. ) ;
#22490=TOROIDAL_SURFACE ( 'NONE', #29018, 24.50000000000000000, 3.200000000000000178 ) ;
#22517=CARTESIAN_POINT ( 'NONE',  ( 22.63992238019999803, -14.34133587289999845, 225.0000000000000000 ) ) ;
#22533=CIRCLE ( 'NONE', #25012, 26.80000000000000071 ) ;
#22552=CARTESIAN_POINT ( 'NONE',  ( 22.63992238019999803, -14.34133587289999845, 5.000000000000000000 ) ) ;
#22554=EDGE_CURVE ( 'NONE', #22455, #2523, #27459, .T. ) ;
#22558=CARTESIAN_POINT ( 'NONE',  ( 23.30309534879319600, -14.60301215399188735, 224.5094458585157327 ) ) ;
#22559=B_SPLINE_CURVE_WITH_KNOTS ( 'NONE', 3,
 ( #25542, #3825, #18286, #13575, #27893, #5859 ),
 .UNSPECIFIED., .F., .F.,
 ( 4, 2, 4 ),
 ( 0.000000000000000000, 0.2632370136849138675, 0.5264740273698277351 ),
 .UNSPECIFIED. ) ;
#22562=DIRECTION ( 'NONE',  ( 0.5000000000001898481, -0.8660254037843291286, 0.000000000000000000 ) ) ;
#22569=CARTESIAN_POINT ( 'NONE',  ( 24.13062658807300664, -13.18986347224536182, 5.913085275126884532 ) ) ;
#22570=( LENGTH_UNIT ( ) NAMED_UNIT ( * ) SI_UNIT ( .MILLI., .METRE. ) );
#22572=CARTESIAN_POINT ( 'NONE',  ( 0.000000000000000000, 0.000000000000000000, 138.3395398250000028 ) ) ;
#22581=DIRECTION ( 'NONE',  ( 0.000000000000000000, 0.000000000000000000, 1.000000000000000000 ) ) ;
#22584=ADVANCED_FACE ( 'NONE', ( #1042 ), #18007, .F. ) ;
#22591=DIRECTION ( 'NONE',  ( 0.000000000000000000, 0.000000000000000000, 1.000000000000000000 ) ) ;
#22594=CARTESIAN_POINT ( 'NONE',  ( -9.251510797979349832, -25.15273151106422489, 204.8526541494500179 ) ) ;
#22600=LINE ( 'NONE', #20080, #27182 ) ;
#22611=ORIENTED_EDGE ( 'NONE', *, *, #12289, .T. ) ;
#22616=CARTESIAN_POINT ( 'NONE',  ( -25.43121960300666728, -8.635379644106548014, 143.2171415880000040 ) ) ;
#22626=CARTESIAN_POINT ( 'NONE',  ( 23.70259205098650312, -12.50815390746196165, 4.579417934479508290 ) ) ;
#22628=CARTESIAN_POINT ( 'NONE',  ( 0.000000000000000000, 0.000000000000000000, 230.0000000000000000 ) ) ;
#22633=CARTESIAN_POINT ( 'NONE',  ( -18.95046173579999760, -18.95046173579999760, 43.21714158840000408 ) ) ;
#22634=CARTESIAN_POINT ( 'NONE',  ( 9.738910687886868089, -24.96785170200598358, 27.99999999999999645 ) ) ;
#22647=DIRECTION ( 'NONE',  ( -1.000000000000000000, 5.665498452320000818E-16, 0.000000000000000000 ) ) ;
#22657=ADVANCED_FACE ( 'NONE', ( #30926, #4805 ), #11877, .T. ) ;
#22668=CARTESIAN_POINT ( 'NONE',  ( -24.50000001620000134, 3.000285568850000245E-15, 140.0000000040000145 ) ) ;
#22674=DIRECTION ( 'NONE',  ( 1.000000000000000000, 0.000000000000000000, 0.000000000000000000 ) ) ;
#22681=FACE_OUTER_BOUND ( 'NONE', #13175, .T. ) ;
#22687=CARTESIAN_POINT ( 'NONE',  ( 26.80000000069999899, -3.281945028320000125E-15, 187.1101814799999943 ) ) ;
#22696=CARTESIAN_POINT ( 'NONE',  ( -27.50000000000000000, 3.367667473009999970E-15, 136.3944487260000074 ) ) ;
#22698=CARTESIAN_POINT ( 'NONE',  ( -23.81569860410000317, -13.75000000000000000, 223.8999999999999773 ) ) ;
#22700=CARTESIAN_POINT ( 'NONE',  ( 24.24391315728334817, -12.98049462746314120, 224.3250316511497147 ) ) ;
#22712=ORIENTED_EDGE ( 'NONE', *, *, #14737, .F. ) ;
#22714=ORIENTED_EDGE ( 'NONE', *, *, #2660, .F. ) ;
#22715=CARTESIAN_POINT ( 'NONE',  ( 23.86403265466892876, -13.66628296867904346, 6.099999999998879652 ) ) ;
#22716=CIRCLE ( 'NONE', #17185, 27.92857142860000152 ) ;
#22722=DIRECTION ( 'NONE',  ( 1.000000000000000000, -1.224606353819999829E-16, 0.000000000000000000 ) ) ;
#22723=B_SPLINE_CURVE_WITH_KNOTS ( 'NONE', 3,
 ( #1057, #3559, #24660, #3094, #5766, #10963, #3251, #12857, #7967, #5917, #5611, #29528 ),
 .UNSPECIFIED., .F., .F.,
 ( 4, 2, 2, 2, 2, 4 ),
 ( 0.000000000000000000, 0.2499999999999658051, 0.3749999999999714673, 0.4999999999999771294, 0.7499999999999885647, 1.000000000000000000 ),
 .UNSPECIFIED. ) ;
#22733=ORIENTED_EDGE ( 'NONE', *, *, #15893, .T. ) ;
#22742=CARTESIAN_POINT ( 'NONE',  ( 22.86552662882814246, -13.97920826333698230, 224.1183286168485722 ) ) ;
#22749=EDGE_CURVE ( 'NONE', #17448, #24430, #20875, .T. ) ;
#22753=TOROIDAL_SURFACE ( 'NONE', #2170, 29.80000000000000071, 3.000000000000000000 ) ;
#22757=VERTEX_POINT ( 'NONE', #15938 ) ;
#22763=LINE ( 'NONE', #3561, #30905 ) ;
#22764=CARTESIAN_POINT ( 'NONE',  ( 9.738910687886868089, -24.96785170200598358, 27.99999999999999645 ) ) ;
#22767=LINE ( 'NONE', #8591, #24046 ) ;
#22769=AXIS2_PLACEMENT_3D ( 'NONE', #12024, #23537, #14236 ) ;
#22775=AXIS2_PLACEMENT_3D ( 'NONE', #7982, #6090, #25302 ) ;
#22780=DIRECTION ( 'NONE',  ( 0.3633921898465272138, -0.9316362575375356503, -1.850371707708593498E-14 ) ) ;
#22782=CARTESIAN_POINT ( 'NONE',  ( -25.38111185550165416, -8.615767840674489975, 43.21714158837188080 ) ) ;
#22789=EDGE_CURVE ( 'NONE', #21137, #3582, #30424, .T. ) ;
#22793=ORIENTED_EDGE ( 'NONE', *, *, #5945, .F. ) ;
#22794=CIRCLE ( 'NONE', #192, 28.50000000000000000 ) ;
#22818=CARTESIAN_POINT ( 'NONE',  ( 22.96035733374347743, -13.82212301974795565, 225.9951937274967690 ) ) ;
#22820=CARTESIAN_POINT ( 'NONE',  ( -27.92857142909999979, 3.420150602519999655E-15, 92.06031501479999690 ) ) ;
#22821=VERTEX_POINT ( 'NONE', #16246 ) ;
#22830=CARTESIAN_POINT ( 'NONE',  ( -8.416763499243886670, -26.18199973230928990, 23.07543701367895039 ) ) ;
#22832=ORIENTED_EDGE ( 'NONE', *, *, #24628, .F. ) ;
#22836=CIRCLE ( 'NONE', #7758, 27.23548387100000312 ) ;
#22838=CARTESIAN_POINT ( 'NONE',  ( 8.903108651239925564, -22.82508830966962421, 190.0000000000000000 ) ) ;
#22843=AXIS2_PLACEMENT_3D ( 'NONE', #30875, #19063, #18746 ) ;
#22848=EDGE_CURVE ( 'NONE', #10260, #15775, #19152, .T. ) ;
#22854=CARTESIAN_POINT ( 'NONE',  ( -0.8360625281005691356, -27.48733646094163063, 5.718668015287994955 ) ) ;
#22873=CARTESIAN_POINT ( 'NONE',  ( 26.84464185210000053, -3.287411897800000213E-15, 137.4375040469999760 ) ) ;
#22880=CARTESIAN_POINT ( 'NONE',  ( 0.000000000000000000, 0.000000000000000000, 90.00000000000000000 ) ) ;
#22881=ORIENTED_EDGE ( 'NONE', *, *, #5949, .T. ) ;
#22898=CARTESIAN_POINT ( 'NONE',  ( 27.50000000000000000, -3.367667472999999580E-15, 230.0000000000000000 ) ) ;
#22899=CARTESIAN_POINT ( 'NONE',  ( 0.000000000000000000, 0.000000000000000000, 115.0000000000000000 ) ) ;
#22900=EDGE_CURVE ( 'NONE', #13409, #16204, #6285, .T. ) ;
#22913=EDGE_CURVE ( 'NONE', #13351, #19505, #9389, .T. ) ;
#22914=DIRECTION ( 'NONE',  ( -0.9316362575375349842, 0.3633921898465292122, -0.000000000000000000 ) ) ;
#22922=EDGE_CURVE ( 'NONE', #24004, #16204, #4765, .T. ) ;
#22933=ORIENTED_EDGE ( 'NONE', *, *, #12057, .F. ) ;
#22935=CARTESIAN_POINT ( 'NONE',  ( 27.92857142909999979, -3.420150602509999660E-15, 137.9396849850000137 ) ) ;
#22965=FACE_OUTER_BOUND ( 'NONE', #22066, .T. ) ;
#22971=CARTESIAN_POINT ( 'NONE',  ( -26.80000000069999899, 3.281945028329999726E-15, 211.6085707940000020 ) ) ;
#22982=ORIENTED_EDGE ( 'NONE', *, *, #22411, .T. ) ;
#22990=ORIENTED_EDGE ( 'NONE', *, *, #18153, .F. ) ;
#22997=VERTEX_POINT ( 'NONE', #2858 ) ;
#22999=VERTEX_POINT ( 'NONE', #12448 ) ;
#23004=CARTESIAN_POINT ( 'NONE',  ( 5.656593618302459880, -26.91642256435905622, 209.2180597379770290 ) ) ;
#23006=LINE ( 'NONE', #25202, #3438 ) ;
#23007=ORIENTED_EDGE ( 'NONE', *, *, #18618, .T. ) ;
#23014=EDGE_CURVE ( 'NONE', #8508, #10260, #30915, .T. ) ;
#23023=CARTESIAN_POINT ( 'NONE',  ( -3.552713678799999608E-15, -3.552713678799999608E-15, 143.2171415880000040 ) ) ;
#23037=TOROIDAL_SURFACE ( 'NONE', #23542, 30.50000000000000000, 3.000000000000000000 ) ;
#23038=CARTESIAN_POINT ( 'NONE',  ( -26.80000000000002203, -1.754055898254307966, 186.7828584129167098 ) ) ;
#23042=TOROIDAL_SURFACE ( 'NONE', #22053, 24.50000000000000000, 4.000000000000000000 ) ;
#23050=ORIENTED_EDGE ( 'NONE', *, *, #5279, .T. ) ;
#23074=CARTESIAN_POINT ( 'NONE',  ( -24.34663841809999951, -12.78636765230000094, 225.0000000000000000 ) ) ;
#23077=DIRECTION ( 'NONE',  ( 0.3633921898465289901, 0.9316362575375348731, -8.673617379884029161E-15 ) ) ;
#23082=ORIENTED_EDGE ( 'NONE', *, *, #28825, .T. ) ;
#23084=TOROIDAL_SURFACE ( 'NONE', #27095, 24.50000000000000000, 4.000000000000000000 ) ;
#23092=FACE_OUTER_BOUND ( 'NONE', #27769, .T. ) ;
#23096=EDGE_CURVE ( 'NONE', #8364, #21606, #17173, .T. ) ;
#23103=CARTESIAN_POINT ( 'NONE',  ( -0.9598841924169057016, -27.48329941561060252, 225.5561643546540722 ) ) ;
#23106=VECTOR ( 'NONE', #30152, 1000.000000000000000 ) ;
#23107=EDGE_CURVE ( 'NONE', #1493, #20367, #7227, .T. ) ;
#23109=CARTESIAN_POINT ( 'NONE',  ( -23.25354871329894024, -14.68148953537939860, 5.217924949212490837 ) ) ;
#23124=DIRECTION ( 'NONE',  ( 1.224606353819999829E-16, 1.000000000000000000, 0.000000000000000000 ) ) ;
#23132=FACE_OUTER_BOUND ( 'NONE', #21642, .T. ) ;
#23141=CARTESIAN_POINT ( 'NONE',  ( 22.70120178298296310, -14.24511786442693939, 225.4947892891584047 ) ) ;
#23142=CIRCLE ( 'NONE', #3024, 26.80000000000000071 ) ;
#23162=DIRECTION ( 'NONE',  ( -0.9316362575375349842, 0.3633921898465292122, -0.000000000000000000 ) ) ;
#23164=CARTESIAN_POINT ( 'NONE',  ( -27.06563796000000366, 3.314475221609999872E-15, 138.0597313979999967 ) ) ;
#23174=DIRECTION ( 'NONE',  ( 1.000000000000000000, 0.000000000000000000, 0.000000000000000000 ) ) ;
#23187=DIRECTION ( 'NONE',  ( 1.000000000000000000, 0.000000000000000000, 0.000000000000000000 ) ) ;
#23188=CARTESIAN_POINT ( 'NONE',  ( 3.466821295769682159E-14, -2.890242878314739659E-13, 277.5163816122566800 ) ) ;
#23192=CARTESIAN_POINT ( 'NONE',  ( -25.43121960300668150, -8.635379644106590646, 186.7828584125833515 ) ) ;
#23196=EDGE_CURVE ( 'NONE', #28212, #13351, #8968, .T. ) ;
#23201=B_SPLINE_CURVE_WITH_KNOTS ( 'NONE', 3,
 ( #25537, #1000, #25217, #20651, #22700, #27888, #8361, #11208, #4127, #3974 ),
 .UNSPECIFIED., .F., .F.,
 ( 4, 2, 2, 2, 4 ),
 ( 0.000000000000000000, 0.2500000000000000000, 0.5000000000000000000, 0.7500000000000000000, 1.000000000000000000 ),
 .UNSPECIFIED. ) ;
#23208=DIRECTION ( 'NONE',  ( 1.000000000000000000, 0.000000000000000000, 0.000000000000000000 ) ) ;
#23219=ORIENTED_EDGE ( 'NONE', *, *, #7848, .T. ) ;
#23222=EDGE_CURVE ( 'NONE', #17862, #24922, #11325, .T. ) ;
#23231=ORIENTED_EDGE ( 'NONE', *, *, #16565, .T. ) ;
#23239=PRESENTATION_STYLE_ASSIGNMENT (( #13948 ) ) ;
#23243=CARTESIAN_POINT ( 'NONE',  ( 1.065814103639999922E-14, -1.065814103639999922E-14, 143.6055512749999821 ) ) ;
#23251=CARTESIAN_POINT ( 'NONE',  ( 23.45268582460785112, -12.96920632855593425, 4.006804827044976314 ) ) ;
#23263=VERTEX_POINT ( 'NONE', #25666 ) ;
#23277=CARTESIAN_POINT ( 'NONE',  ( 0.000000000000000000, 0.000000000000000000, 188.3395398250000028 ) ) ;
#23278=DIRECTION ( 'NONE',  ( 0.000000000000000000, 0.000000000000000000, 1.000000000000000000 ) ) ;
#23283=DIRECTION ( 'NONE',  ( -0.000000000000000000, -0.000000000000000000, -1.000000000000000000 ) ) ;
#23286=EDGE_CURVE ( 'NONE', #7351, #22999, #30777, .T. ) ;
#23295=AXIS2_PLACEMENT_3D ( 'NONE', #26270, #317, #24071 ) ;
#23299=DIRECTION ( 'NONE',  ( 0.8660254037843289066, -0.5000000000001899592, 0.000000000000000000 ) ) ;
#23302=ORIENTED_EDGE ( 'NONE', *, *, #26362, .F. ) ;
#23315=DIRECTION ( 'NONE',  ( 0.3633921898465291567, 0.9316362575375349842, -6.938893903907229167E-15 ) ) ;
#23318=CARTESIAN_POINT ( 'NONE',  ( 23.20948082139999968, -13.40000000000000036, 6.099999999630000502 ) ) ;
#23319=AXIS2_PLACEMENT_3D ( 'NONE', #9073, #1540, #23417 ) ;
#23321=CIRCLE ( 'NONE', #1708, 3.199999983039998774 ) ;
#23322=ORIENTED_EDGE ( 'NONE', *, *, #23196, .F. ) ;
#23323=AXIS2_PLACEMENT_3D ( 'NONE', #19271, #399, #14243 ) ;
#23326=AXIS2_PLACEMENT_3D ( 'NONE', #17893, #8141, #783 ) ;
#23327=DIRECTION ( 'NONE',  ( 1.000000000000000000, -1.224606353820000075E-16, 0.000000000000000000 ) ) ;
#23330=CARTESIAN_POINT ( 'NONE',  ( -23.35113490818136839, -13.15228900125540434, 223.9278743037135655 ) ) ;
#23343=ORIENTED_EDGE ( 'NONE', *, *, #19252, .T. ) ;
#23348=DIRECTION ( 'NONE',  ( -0.9316362575375356503, -0.3633921898465275468, 0.000000000000000000 ) ) ;
#23349=AXIS2_PLACEMENT_3D ( 'NONE', #23023, #11060, #3340 ) ;
#23354=CIRCLE ( 'NONE', #6758, 3.000000000000001332 ) ;
#23357=VECTOR ( 'NONE', #22591, 1000.000000000000000 ) ;
#23360=CARTESIAN_POINT ( 'NONE',  ( 23.81569860410000317, -13.75000000000000000, 3.900000000369999942 ) ) ;
#23364=CARTESIAN_POINT ( 'NONE',  ( -0.5612683859346103699, -26.79446734600721314, 224.0425474258357212 ) ) ;
#23372=DIRECTION ( 'NONE',  ( 1.000000000000000000, 0.000000000000000000, 0.000000000000000000 ) ) ;
#23374=CIRCLE ( 'NONE', #9794, 27.50000000000000000 ) ;
#23377=CARTESIAN_POINT ( 'NONE',  ( 9.993285220779439371, -25.61999708228226069, 36.39444872359999295 ) ) ;
#23378=DIRECTION ( 'NONE',  ( 0.000000000000000000, 0.000000000000000000, -1.000000000000000000 ) ) ;
#23392=TOROIDAL_SURFACE ( 'NONE', #7291, 24.50000000000000000, 3.200000000000000178 ) ;
#23413=ORIENTED_EDGE ( 'NONE', *, *, #7926, .F. ) ;
#23415=CARTESIAN_POINT ( 'NONE',  ( 0.8784916434280891639, -26.78562594471228664, 225.6660761023112229 ) ) ;
#23417=DIRECTION ( 'NONE',  ( 1.000000000000000000, 0.000000000000000000, 0.000000000000000000 ) ) ;
#23419=CARTESIAN_POINT ( 'NONE',  ( -10.14902473071360411, -26.01926976408356396, 92.06031501460000754 ) ) ;
#23429=CARTESIAN_POINT ( 'NONE',  ( -24.34663841809999951, -12.78636765230000094, 225.0000000000000000 ) ) ;
#23435=ORIENTED_EDGE ( 'NONE', *, *, #27360, .T. ) ;
#23438=DIRECTION ( 'NONE',  ( 0.000000000000000000, 0.000000000000000000, 1.000000000000000000 ) ) ;
#23446=CARTESIAN_POINT ( 'NONE',  ( 27.54391552379999908, -3.373045395939999845E-15, 92.95625301640001226 ) ) ;
#23453=CARTESIAN_POINT ( 'NONE',  ( -0.8466629511608627645, -26.78674366427728160, 5.703642739696129560 ) ) ;
#23461=LINE ( 'NONE', #11337, #21295 ) ;
#23462=ORIENTED_EDGE ( 'NONE', *, *, #13667, .T. ) ;
#23472=B_SPLINE_CURVE_WITH_KNOTS ( 'NONE', 3,
 ( #28052, #18610, #23507, #6181, #30104, #28207, #8371, #3660, #15939, #13581 ),
 .UNSPECIFIED., .F., .F.,
 ( 4, 2, 2, 2, 4 ),
 ( 0.000000000000000000, 0.2499999999999998890, 0.4999999999999997780, 0.7499999999999998890, 1.000000000000000000 ),
 .UNSPECIFIED. ) ;
#23489=EDGE_CURVE ( 'NONE', #13152, #3686, #14835, .T. ) ;
#23495=AXIS2_PLACEMENT_3D ( 'NONE', #13674, #23278, #25485 ) ;
#23505=ORIENTED_EDGE ( 'NONE', *, *, #25652, .T. ) ;
#23507=CARTESIAN_POINT ( 'NONE',  ( 21.30888436558567633, -16.34772642260384856, 186.7828584119999960 ) ) ;
#23509=ORIENTED_EDGE ( 'NONE', *, *, #4559, .T. ) ;
#23524=ORIENTED_EDGE ( 'NONE', *, *, #6043, .T. ) ;
#23528=CARTESIAN_POINT ( 'NONE',  ( 25.43291179139270142, -8.631520107455976643, -0.000000000000000000 ) ) ;
#23534=CARTESIAN_POINT ( 'NONE',  ( 23.13573312470881405, -13.52773475764968225, 3.899999999999999911 ) ) ;
#23536=CIRCLE ( 'NONE', #16974, 3.200000000000002398 ) ;
#23537=DIRECTION ( 'NONE',  ( 0.000000000000000000, 0.000000000000000000, 1.000000000000000000 ) ) ;
#23540=DIRECTION ( 'NONE',  ( 0.000000000000000000, -0.000000000000000000, 1.000000000000000000 ) ) ;
#23542=AXIS2_PLACEMENT_3D ( 'NONE', #7617, #9524, #4954 ) ;
#23553=VERTEX_POINT ( 'NONE', #9376 ) ;
#23556=EDGE_CURVE ( 'NONE', #21828, #28697, #15782, .T. ) ;
#23561=DIRECTION ( 'NONE',  ( 0.000000000000000000, 0.000000000000000000, 1.000000000000000000 ) ) ;
#23566=CIRCLE ( 'NONE', #30079, 4.000000004070001225 ) ;
#23568=CARTESIAN_POINT ( 'NONE',  ( 0.000000000000000000, 0.000000000000000000, 90.00000000000000000 ) ) ;
#23569=VERTEX_POINT ( 'NONE', #20490 ) ;
#23581=CARTESIAN_POINT ( 'NONE',  ( 27.15000000039999861, -3.324806250660000050E-15, 230.0000000000000000 ) ) ;
#23591=DIRECTION ( 'NONE',  ( -1.000000000000000000, 5.665498452320000818E-16, 0.000000000000000000 ) ) ;
#23593=EDGE_LOOP ( 'NONE', ( #14238, #29982, #24258, #30083 ) ) ;
#23595=CARTESIAN_POINT ( 'NONE',  ( -9.897162125403687227, -25.37356426577970581, 91.66046017469999185 ) ) ;
#23604=CARTESIAN_POINT ( 'NONE',  ( 0.000000000000000000, 0.000000000000000000, 230.0000000000000000 ) ) ;
#23615=EDGE_CURVE ( 'NONE', #9708, #9436, #28338, .T. ) ;
#23617=ORIENTED_EDGE ( 'NONE', *, *, #17586, .F. ) ;
#23632=CARTESIAN_POINT ( 'NONE',  ( -7.105427357599999217E-15, -7.105427357599999217E-15, 186.7828584120000244 ) ) ;
#23641=DIRECTION ( 'NONE',  ( 0.9316362575375356503, 0.3633921898465274913, 0.000000000000000000 ) ) ;
#23651=DIRECTION ( 'NONE',  ( -0.9316362575375349842, 0.3633921898465292122, -0.000000000000000000 ) ) ;
#23658=ORIENTED_EDGE ( 'NONE', *, *, #26147, .T. ) ;
#23681=DIRECTION ( 'NONE',  ( 0.000000000000000000, 0.000000000000000000, -1.000000000000000000 ) ) ;
#23694=B_SPLINE_CURVE_WITH_KNOTS ( 'NONE', 3,
 ( #17780, #17930, #30064, #3316, #18091, #29751, #822, #5833, #15281, #8034, #1120, #20309 ),
 .UNSPECIFIED., .F., .F.,
 ( 4, 2, 2, 2, 2, 4 ),
 ( 0.000000000000000000, 0.2500000000000002776, 0.3750000000000002776, 0.5000000000000003331, 0.7500000000000001110, 1.000000000000000000 ),
 .UNSPECIFIED. ) ;
#23698=CARTESIAN_POINT ( 'NONE',  ( 27.23548387060000309, -1.776356839399999804E-15, 188.3395398250000028 ) ) ;
#23713=CARTESIAN_POINT ( 'NONE',  ( 26.80000000000000071, -1.776356839399999804E-15, 43.21714158840000408 ) ) ;
#23715=ORIENTED_EDGE ( 'NONE', *, *, #13033, .F. ) ;
#23716=CARTESIAN_POINT ( 'NONE',  ( -26.80000000069999899, 3.281945028329999726E-15, 193.2171415869999862 ) ) ;
#23723=CARTESIAN_POINT ( 'NONE',  ( 0.000000000000000000, 0.000000000000000000, 188.3395398250000028 ) ) ;
#23737=AXIS2_PLACEMENT_3D ( 'NONE', #28228, #9503, #19103 ) ;
#23750=DIRECTION ( 'NONE',  ( 0.000000000000000000, 0.000000000000000000, -1.000000000000000000 ) ) ;
#23761=DIRECTION ( 'NONE',  ( 0.000000000000000000, 0.000000000000000000, 1.000000000000000000 ) ) ;
#23764=EDGE_CURVE ( 'NONE', #7351, #9833, #12364, .T. ) ;
#23789=EDGE_CURVE ( 'NONE', #17696, #15285, #28096, .T. ) ;
#23792=DIRECTION ( 'NONE',  ( 0.7071067811865475727, -0.7071067811865475727, 0.000000000000000000 ) ) ;
#23794=CIRCLE ( 'NONE', #26379, 2.999999999999999556 ) ;
#23801=CARTESIAN_POINT ( 'NONE',  ( 0.000000000000000000, 0.000000000000000000, 40.00000000000000000 ) ) ;
#23813=VERTEX_POINT ( 'NONE', #24488 ) ;
#23816=CARTESIAN_POINT ( 'NONE',  ( 26.93395403039999891, -3.298349123909999533E-15, 37.75675929319999824 ) ) ;
#23819=VECTOR ( 'NONE', #30212, 1000.000000000000000 ) ;
#23849=AXIS2_PLACEMENT_3D ( 'NONE', #580, #12203, #29342 ) ;
#23850=CARTESIAN_POINT ( 'NONE',  ( 0.000000000000000000, 0.000000000000000000, 115.0000000000000000 ) ) ;
#23858=ORIENTED_EDGE ( 'NONE', *, *, #19773, .T. ) ;
#23870=B_SPLINE_CURVE_WITH_KNOTS ( 'NONE', 5,
 ( #11643, #14161, #6450, #25968, #28165, #21242 ),
 .UNSPECIFIED., .F., .F.,
 ( 6, 6 ),
 ( -2.300779717630000221, 0.000000000000000000 ),
 .UNSPECIFIED. ) ;
#23874=FACE_OUTER_BOUND ( 'NONE', #24132, .T. ) ;
#23875=CARTESIAN_POINT ( 'NONE',  ( 0.8355090511298449707, -26.78702287612135891, 225.7193154187195603 ) ) ;
#23886=EDGE_CURVE ( 'NONE', #4374, #10417, #1069, .T. ) ;
#23888=CARTESIAN_POINT ( 'NONE',  ( -23.88846875299723393, -13.62395840478711762, 6.099999999630012937 ) ) ;
#23895=EDGE_LOOP ( 'NONE', ( #27869, #11143, #18888, #28013 ) ) ;
#23911=DIRECTION ( 'NONE',  ( 1.000000000000000000, -5.551115123130002122E-16, 0.000000000000000000 ) ) ;
#23926=CARTESIAN_POINT ( 'NONE',  ( -26.80000000000000071, 9.769962616700000205E-15, 36.78285841159999592 ) ) ;
#23931=ORIENTED_EDGE ( 'NONE', *, *, #1982, .F. ) ;
#23934=VERTEX_POINT ( 'NONE', #17689 ) ;
#23939=EDGE_CURVE ( 'NONE', #23813, #3101, #10825, .T. ) ;
#23945=EDGE_CURVE ( 'NONE', #8194, #9526, #27768, .T. ) ;
#23946=EDGE_CURVE ( 'NONE', #9708, #13263, #30866, .T. ) ;
#23957=CARTESIAN_POINT ( 'NONE',  ( 1.841797396446237967, -26.73663745407121795, 20.00000000000000355 ) ) ;
#23969=VERTEX_POINT ( 'NONE', #6212 ) ;
#23982=VERTEX_POINT ( 'NONE', #10784 ) ;
#23988=CARTESIAN_POINT ( 'NONE',  ( 0.9245300016271229548, -27.48475604047800047, 5.597451638069735225 ) ) ;
#23994=FACE_OUTER_BOUND ( 'NONE', #2748, .T. ) ;
#23995=DIRECTION ( 'NONE',  ( 0.3633921898465291567, 0.9316362575375349842, 1.850371707708594444E-14 ) ) ;
#23999=EDGE_CURVE ( 'NONE', #22441, #11915, #30720, .T. ) ;
#24000=DIRECTION ( 'NONE',  ( 0.000000000000000000, 0.000000000000000000, -1.000000000000000000 ) ) ;
#24004=VERTEX_POINT ( 'NONE', #13297 ) ;
#24021=ORIENTED_EDGE ( 'NONE', *, *, #14841, .F. ) ;
#24040=EDGE_LOOP ( 'NONE', ( #7651, #26941, #25512, #14986 ) ) ;
#24046=VECTOR ( 'NONE', #20408, 1000.000000000000000 ) ;
#24049=EDGE_CURVE ( 'NONE', #28478, #24307, #1730, .T. ) ;
#24071=DIRECTION ( 'NONE',  ( 0.3633921898465272138, -0.9316362575375356503, 0.000000000000000000 ) ) ;
#24076=ORIENTED_EDGE ( 'NONE', *, *, #27582, .T. ) ;
#24086=VERTEX_POINT ( 'NONE', #11716 ) ;
#24087=CYLINDRICAL_SURFACE ( 'NONE', #24531, 8.000000000000000000 ) ;
#24104=CARTESIAN_POINT ( 'NONE',  ( -23.48807013395677856, -14.30280389748388359, 225.9130852761126107 ) ) ;
#24105=CARTESIAN_POINT ( 'NONE',  ( 6.112318018889860483, -26.81313817375426112, 21.03870473235707550 ) ) ;
#24107=CARTESIAN_POINT ( 'NONE',  ( -9.993285220779545952, -25.61999708228220740, 193.6055512750000105 ) ) ;
#24109=DIRECTION ( 'NONE',  ( 0.000000000000000000, 0.000000000000000000, -1.000000000000000000 ) ) ;
#24116=VERTEX_POINT ( 'NONE', #11871 ) ;
#24117=DIRECTION ( 'NONE',  ( 0.000000000000000000, 0.000000000000000000, 1.000000000000000000 ) ) ;
#24120=ORIENTED_EDGE ( 'NONE', *, *, #15461, .F. ) ;
#24121=EDGE_LOOP ( 'NONE', ( #16263, #17631, #25598, #7277 ) ) ;
#24132=EDGE_LOOP ( 'NONE', ( #2670, #19005, #26641, #12218 ) ) ;
#24137=CARTESIAN_POINT ( 'NONE',  ( -2.962149026499999369E-14, -27.50000000069999828, 6.100000000000000533 ) ) ;
#24138=DIRECTION ( 'NONE',  ( 0.3633921898465291567, 0.9316362575375348731, -0.000000000000000000 ) ) ;
#24168=CARTESIAN_POINT ( 'NONE',  ( -27.06563794070000029, 3.314475219249999806E-15, 191.9402686260000053 ) ) ;
#24178=CARTESIAN_POINT ( 'NONE',  ( -0.6479069133012533843, -26.79235980095155512, 225.9098122281707788 ) ) ;
#24193=DIRECTION ( 'NONE',  ( -0.9316362575375349842, 0.3633921898465292122, -0.000000000000000000 ) ) ;
#24206=DIRECTION ( 'NONE',  ( 1.000000000000000000, 0.000000000000000000, 0.000000000000000000 ) ) ;
#24210=LINE ( 'NONE', #26720, #17517 ) ;
#24227=ORIENTED_EDGE ( 'NONE', *, *, #21634, .T. ) ;
#24228=ORIENTED_EDGE ( 'NONE', *, *, #19127, .F. ) ;
#24238=CARTESIAN_POINT ( 'NONE',  ( -22.78048776543632670, -14.11708351994821165, 5.719315394042070011 ) ) ;
#24245=CARTESIAN_POINT ( 'NONE',  ( 0.000000000000000000, 0.000000000000000000, 142.0603150149999863 ) ) ;
#24253=AXIS2_PLACEMENT_3D ( 'NONE', #30997, #26277, #26128 ) ;
#24258=ORIENTED_EDGE ( 'NONE', *, *, #11856, .F. ) ;
#24267=EDGE_CURVE ( 'NONE', #23969, #25641, #24839, .T. ) ;
#24270=DIRECTION ( 'NONE',  ( 0.3090169943750400994, -0.9510565162951234441, 0.000000000000000000 ) ) ;
#24274=CARTESIAN_POINT ( 'NONE',  ( -14.94562240850000023, -8.628859120750000500, 5.000000000000000000 ) ) ;
#24283=CARTESIAN_POINT ( 'NONE',  ( 26.80000000069999899, -3.281945028320000125E-15, 86.78285841090000474 ) ) ;
#24288=EDGE_CURVE ( 'NONE', #5682, #23569, #20570, .T. ) ;
#24290=DIRECTION ( 'NONE',  ( 0.3633921898465291567, 0.9316362575375349842, 0.000000000000000000 ) ) ;
#24298=AXIS2_PLACEMENT_3D ( 'NONE', #22668, #19998, #1431 ) ;
#24303=AXIS2_PLACEMENT_3D ( 'NONE', #11073, #20510, #16670 ) ;
#24307=VERTEX_POINT ( 'NONE', #13247 ) ;
#24311=EDGE_CURVE ( 'NONE', #27823, #18767, #1756, .T. ) ;
#24321=VERTEX_POINT ( 'NONE', #13408 ) ;
#24323=CARTESIAN_POINT ( 'NONE',  ( 23.73463268742296961, -12.44713172126245126, 224.7819332099832081 ) ) ;
#24324=AXIS2_PLACEMENT_3D ( 'NONE', #16160, #18037, #25774 ) ;
#24325=AXIS2_PLACEMENT_3D ( 'NONE', #15731, #25345, #969 ) ;
#24355=FACE_BOUND ( 'NONE', #26818, .T. ) ;
#24363=VERTEX_POINT ( 'NONE', #15312 ) ;
#24368=CARTESIAN_POINT ( 'NONE',  ( 1.100000000000000089, -27.47799119300000115, 225.0000000000000000 ) ) ;
#24371=DIRECTION ( 'NONE',  ( 0.9316362575375356503, 0.3633921898465274913, 0.000000000000000000 ) ) ;
#24376=CARTESIAN_POINT ( 'NONE',  ( -2.664535259099999568E-14, -26.80000000000000071, 223.8999999999999773 ) ) ;
#24389=VERTEX_POINT ( 'NONE', #20494 ) ;
#24391=VERTEX_POINT ( 'NONE', #18123 ) ;
#24409=EDGE_CURVE ( 'NONE', #7124, #1598, #18810, .T. ) ;
#24419=ORIENTED_EDGE ( 'NONE', *, *, #14790, .F. ) ;
#24421=CARTESIAN_POINT ( 'NONE',  ( -23.81569860410000317, -13.75000000000000000, 6.099999999630000502 ) ) ;
#24427=VERTEX_POINT ( 'NONE', #27418 ) ;
#24430=VERTEX_POINT ( 'NONE', #12794 ) ;
#24433=DIRECTION ( 'NONE',  ( 0.3633921898465289901, 0.9316362575375348731, 0.000000000000000000 ) ) ;
#24441=ORIENTED_EDGE ( 'NONE', *, *, #4504, .T. ) ;
#24446=DIRECTION ( 'NONE',  ( 0.9316362575375356503, 0.3633921898465274913, 0.000000000000000000 ) ) ;
#24450=ADVANCED_FACE ( 'NONE', ( #4445 ), #17306, .F. ) ;
#24459=EDGE_CURVE ( 'NONE', #4649, #19818, #27347, .T. ) ;
#24461=ORIENTED_EDGE ( 'NONE', *, *, #2133, .T. ) ;
#24466=ORIENTED_EDGE ( 'NONE', *, *, #23489, .F. ) ;
#24474=CARTESIAN_POINT ( 'NONE',  ( -22.63992238019999803, -14.34133587289999845, 225.0000000000000000 ) ) ;
#24479=ORIENTED_EDGE ( 'NONE', *, *, #12709, .F. ) ;
#24480=FACE_OUTER_BOUND ( 'NONE', #14833, .T. ) ;
#24485=CARTESIAN_POINT ( 'NONE',  ( -2.895630725101765890, -26.64812433595227503, 209.9519070181412701 ) ) ;
#24488=CARTESIAN_POINT ( 'NONE',  ( 27.50000000000000000, -3.367667472999999580E-15, 143.6055512739999926 ) ) ;
#24490=CARTESIAN_POINT ( 'NONE',  ( 0.000000000000000000, 0.000000000000000000, 190.0000000000000000 ) ) ;
#24494=EDGE_CURVE ( 'NONE', #20880, #17294, #14804, .T. ) ;
#24504=CIRCLE ( 'NONE', #13302, 26.80000000000000071 ) ;
#24513=AXIS2_PLACEMENT_3D ( 'NONE', #23632, #2381, #16221 ) ;
#24524=CARTESIAN_POINT ( 'NONE',  ( -27.54391550559999757, 3.373045393730000103E-15, 187.0437466829999948 ) ) ;
#24528=CARTESIAN_POINT ( 'NONE',  ( 0.9876156986561913653, -26.78228253905960798, 224.5086268448359874 ) ) ;
#24531=AXIS2_PLACEMENT_3D ( 'NONE', #9915, #4570, #11655 ) ;
#24534=ORIENTED_EDGE ( 'NONE', *, *, #6301, .T. ) ;
#24536=AXIS2_PLACEMENT_3D ( 'NONE', #5495, #12734, #24549 ) ;
#24548=DIRECTION ( 'NONE',  ( 0.000000000000000000, 0.000000000000000000, -1.000000000000000000 ) ) ;
#24549=DIRECTION ( 'NONE',  ( 0.7071067811865475727, 0.7071067811865475727, 0.000000000000000000 ) ) ;
#24550=CARTESIAN_POINT ( 'NONE',  ( -27.63177356679999974, 3.383804547729999744E-15, 87.36052363810000543 ) ) ;
#24560=CARTESIAN_POINT ( 'NONE',  ( 0.000000000000000000, 0.000000000000000000, 142.0603150149999863 ) ) ;
#24578=DIRECTION ( 'NONE',  ( 0.000000000000000000, 0.000000000000000000, -1.000000000000000000 ) ) ;
#24579=ORIENTED_EDGE ( 'NONE', *, *, #10234, .T. ) ;
#24588=EDGE_LOOP ( 'NONE', ( #30307, #21608, #23082, #4304 ) ) ;
#24595=EDGE_CURVE ( 'NONE', #22078, #1634, #22836, .T. ) ;
#24596=CARTESIAN_POINT ( 'NONE',  ( 27.06563795990000187, -3.314475221579999886E-15, 41.94026860139999258 ) ) ;
#24604=CIRCLE ( 'NONE', #11037, 28.50000000000000000 ) ;
#24605=DIRECTION ( 'NONE',  ( -0.9316362575375349842, 0.3633921898465292122, -0.000000000000000000 ) ) ;
#24613=EDGE_CURVE ( 'NONE', #30479, #25858, #30890, .T. ) ;
#24618=DIRECTION ( 'NONE',  ( 0.3633921898465289901, 0.9316362575375348731, 2.168404344971007290E-15 ) ) ;
#24621=DIRECTION ( 'NONE',  ( -0.3090169943750401549, -0.9510565162951233331, 0.000000000000000000 ) ) ;
#24624=CARTESIAN_POINT ( 'NONE',  ( 18.95046173579999760, -18.95046173579999760, 115.0000000000000000 ) ) ;
#24628=EDGE_CURVE ( 'NONE', #7590, #26174, #28365, .T. ) ;
#24630=ORIENTED_EDGE ( 'NONE', *, *, #17325, .F. ) ;
#24631=CARTESIAN_POINT ( 'NONE',  ( 9.738910687886868089, -24.96785170200598358, 36.78285841123148003 ) ) ;
#24638=CIRCLE ( 'NONE', #13954, 27.50000000000000000 ) ;
#24646=CARTESIAN_POINT ( 'NONE',  ( -19.81582138730396636, -18.05844329259051051, 93.21714158843887787 ) ) ;
#24650=DIRECTION ( 'NONE',  ( 1.000000000000000000, 0.000000000000000000, 0.000000000000000000 ) ) ;
#24657=VERTEX_POINT ( 'NONE', #5057 ) ;
#24660=CARTESIAN_POINT ( 'NONE',  ( -23.73463268736954035, -12.44713172136066248, 225.2180667906550298 ) ) ;
#24661=DIRECTION ( 'NONE',  ( 0.000000000000000000, 0.000000000000000000, -1.000000000000000000 ) ) ;
#24662=B_SPLINE_CURVE_WITH_KNOTS ( 'NONE', 3,
 ( #9178, #16267, #13917, #14076, #18780, #23528, #6202, #11557, #15804, #28389 ),
 .UNSPECIFIED., .F., .F.,
 ( 4, 2, 2, 2, 4 ),
 ( 0.000000000000000000, 0.2500000000000001665, 0.5000000000000001110, 0.7500000000000000000, 1.000000000000000000 ),
 .UNSPECIFIED. ) ;
#24671=TOROIDAL_SURFACE ( 'NONE', #8078, 24.50000000000000000, 3.200000000000000178 ) ;
#24673=CARTESIAN_POINT ( 'NONE',  ( 23.73992238019999945, -12.43607998449999918, 5.000000000000000000 ) ) ;
#24675=CARTESIAN_POINT ( 'NONE',  ( -27.63177356800000339, 3.383804547869999678E-15, 187.3605236429999934 ) ) ;
#24676=DIRECTION ( 'NONE',  ( 1.000000000000000000, 0.000000000000000000, 0.000000000000000000 ) ) ;
#24683=CARTESIAN_POINT ( 'NONE',  ( 9.481612630793602392, -25.06681236668577384, 25.90123088588473976 ) ) ;
#24692=VECTOR ( 'NONE', #28661, 1000.000000000000000 ) ;
#24695=VERTEX_POINT ( 'NONE', #9469 ) ;
#24699=CARTESIAN_POINT ( 'NONE',  ( -1.841797396446221091, -26.73663745407121795, 210.0000000000000284 ) ) ;
#24700=CARTESIAN_POINT ( 'NONE',  ( 10.14902473063354194, -26.01926976387845158, 192.0603150150000147 ) ) ;
#24727=CARTESIAN_POINT ( 'NONE',  ( -9.506387914194311506, -25.80482363264563972, 25.14863730271530073 ) ) ;
#24731=DIRECTION ( 'NONE',  ( 0.000000000000000000, 0.000000000000000000, 1.000000000000000000 ) ) ;
#24737=EDGE_CURVE ( 'NONE', #27983, #22821, #10557, .T. ) ;
#24743=CARTESIAN_POINT ( 'NONE',  ( 7.554893095320836416, -26.44255681430371041, 207.8813784578385935 ) ) ;
#24745=CARTESIAN_POINT ( 'NONE',  ( 8.903108651239925564, -22.82508830966962421, 140.0000000000000000 ) ) ;
#24748=AXIS2_PLACEMENT_3D ( 'NONE', #10638, #20229, #29823 ) ;
#24750=CARTESIAN_POINT ( 'NONE',  ( 23.47117976016943430, -14.33053685725933235, 225.8804910026547077 ) ) ;
#24759=CIRCLE ( 'NONE', #30283, 2.999999999999999556 ) ;
#24765=EDGE_CURVE ( 'NONE', #13324, #13818, #29533, .T. ) ;
#24768=PRESENTATION_STYLE_ASSIGNMENT (( #15020 ) ) ;
#24783=CARTESIAN_POINT ( 'NONE',  ( -27.06563795990000187, 3.314475221589999487E-15, 91.94026860140000679 ) ) ;
#24788=DIRECTION ( 'NONE',  ( 0.000000000000000000, 0.000000000000000000, 1.000000000000000000 ) ) ;
#24794=CARTESIAN_POINT ( 'NONE',  ( -1.100000000000000089, -26.77741585740000119, 225.0000000000000000 ) ) ;
#24795=EDGE_CURVE ( 'NONE', #12078, #16428, #23374, .T. ) ;
#24799=CARTESIAN_POINT ( 'NONE',  ( -2.898287520842993015, -26.64792758275492446, 20.04810862688719553 ) ) ;
#24805=FACE_OUTER_BOUND ( 'NONE', #7538, .T. ) ;
#24809=ORIENTED_EDGE ( 'NONE', *, *, #14060, .F. ) ;
#24811=ORIENTED_EDGE ( 'NONE', *, *, #20600, .T. ) ;
#24817=CARTESIAN_POINT ( 'NONE',  ( -26.80000000069999899, 3.281945028329999726E-15, 143.2171415869999862 ) ) ;
#24819=VECTOR ( 'NONE', #7994, 1000.000000000000000 ) ;
#24831=CARTESIAN_POINT ( 'NONE',  ( 3.466821295769682159E-14, -2.890242878314739659E-13, 202.0000000000000000 ) ) ;
#24835=CARTESIAN_POINT ( 'NONE',  ( -26.80000000000000071, 1.065814103639999922E-14, 86.78285841159998881 ) ) ;
#24839=CIRCLE ( 'NONE', #11274, 3.199999983039998774 ) ;
#24840=AXIS2_PLACEMENT_3D ( 'NONE', #6806, #16402, #28670 ) ;
#24842=CARTESIAN_POINT ( 'NONE',  ( 24.34131725956216030, -12.79741914639830647, 225.2179249505068981 ) ) ;
#24844=VECTOR ( 'NONE', #21351, 1000.000000000000000 ) ;
#24854=ORIENTED_EDGE ( 'NONE', *, *, #380, .T. ) ;
#24862=CARTESIAN_POINT ( 'NONE',  ( -1.421085471519999843E-14, -1.065814103639999922E-14, 136.7828584120000244 ) ) ;
#24866=CARTESIAN_POINT ( 'NONE',  ( -27.92857142909999979, 3.420150602519999655E-15, 42.06031501480000401 ) ) ;
#24868=VECTOR ( 'NONE', #17549, 1000.000000000000000 ) ;
#24875=CARTESIAN_POINT ( 'NONE',  ( 22.63992238021891978, -14.34133587286723532, 225.0964353485933600 ) ) ;
#24880=ORIENTED_EDGE ( 'NONE', *, *, #27532, .T. ) ;
#24882=DIRECTION ( 'NONE',  ( -0.8660254037843290176, 0.5000000000001899592, 0.000000000000000000 ) ) ;
#24883=ORIENTED_EDGE ( 'NONE', *, *, #21795, .T. ) ;
#24888=CARTESIAN_POINT ( 'NONE',  ( -5.656593618302445670, -26.91642256435905978, 20.78194026202293543 ) ) ;
#24890=VERTEX_POINT ( 'NONE', #6761 ) ;
#24894=CARTESIAN_POINT ( 'NONE',  ( -9.897162125400482680, -25.37356426577147417, 88.33953982530000815 ) ) ;
#24896=DIRECTION ( 'NONE',  ( -0.3090169943750401549, -0.9510565162951233331, 0.000000000000000000 ) ) ;
#24897=DIRECTION ( 'NONE',  ( 1.000000000000000000, -1.224606353819999582E-16, 0.000000000000000000 ) ) ;
#24909=CARTESIAN_POINT ( 'NONE',  ( -27.50000000000000000, 3.367667473009999970E-15, 136.7190980919999959 ) ) ;
#24911=DIRECTION ( 'NONE',  ( 1.000000000000000000, -1.224606353820000075E-16, 0.000000000000000000 ) ) ;
#24912=B_SPLINE_CURVE_WITH_KNOTS ( 'NONE', 3,
 ( #20479, #11356, #28025, #20638, #4114, #6320, #13713, #3960, #8667, #8986, #11195, #23318 ),
 .UNSPECIFIED., .F., .F.,
 ( 4, 2, 2, 2, 2, 4 ),
 ( 0.000000000000000000, 0.2500000000000037192, 0.3750000000000043299, 0.5000000000000049960, 0.7500000000000024425, 1.000000000000000000 ),
 .UNSPECIFIED. ) ;
#24914=CYLINDRICAL_SURFACE ( 'NONE', #2208, 26.80000000000002203 ) ;
#24918=CYLINDRICAL_SURFACE ( 'NONE', #26376, 1.099999999999998979 ) ;
#24922=VERTEX_POINT ( 'NONE', #11488 ) ;
#24925=( NAMED_UNIT ( * ) PLANE_ANGLE_UNIT ( ) SI_UNIT ( $, .RADIAN. ) );
#24937=CARTESIAN_POINT ( 'NONE',  ( -27.06563795990000187, 3.314475221589999487E-15, 41.94026860139999258 ) ) ;
#24938=CARTESIAN_POINT ( 'NONE',  ( -26.80000000069999899, 3.281945028329999726E-15, 93.21714158910000947 ) ) ;
#24947=CARTESIAN_POINT ( 'NONE',  ( 22.75759212980393187, -14.15424219578301113, 224.3233986261513451 ) ) ;
#24948=ORIENTED_EDGE ( 'NONE', *, *, #12589, .T. ) ;
#24951=ADVANCED_FACE ( 'NONE', ( #9269 ), #18875, .F. ) ;
#24953=CARTESIAN_POINT ( 'NONE',  ( -6.076762841307600915, -26.10292173851732400, 21.17116608273227740 ) ) ;
#24977=CARTESIAN_POINT ( 'NONE',  ( 23.68794489801944181, -12.53584098811867698, 4.508626838105977086 ) ) ;
#24986=CARTESIAN_POINT ( 'NONE',  ( -21.27344192715450433, -16.32329153680506195, 43.21714158846668141 ) ) ;
#24987=CARTESIAN_POINT ( 'NONE',  ( 3.918707624292984804, -26.51317744985242797, 20.25387219759830160 ) ) ;
#24993=CARTESIAN_POINT ( 'NONE',  ( 10.14902473063354549, -26.01926976387845869, 142.0603150149999863 ) ) ;
#24997=AXIS2_PLACEMENT_3D ( 'NONE', #1408, #8462, #27985 ) ;
#25008=DIRECTION ( 'NONE',  ( 1.000000000000000000, 0.000000000000000000, 0.000000000000000000 ) ) ;
#25010=FACE_OUTER_BOUND ( 'NONE', #16568, .T. ) ;
#25012=AXIS2_PLACEMENT_3D ( 'NONE', #18358, #3719, #25125 ) ;
#25017=DIRECTION ( 'NONE',  ( 0.000000000000000000, 0.000000000000000000, 1.000000000000000000 ) ) ;
#25022=CIRCLE ( 'NONE', #20509, 27.23548387060000309 ) ;
#25032=DIRECTION ( 'NONE',  ( -0.9316362575375349842, 0.3633921898465292122, -0.000000000000000000 ) ) ;
#25034=CARTESIAN_POINT ( 'NONE',  ( -22.77614505619871110, -14.12431931101418492, 224.2880739206591727 ) ) ;
#25037=CARTESIAN_POINT ( 'NONE',  ( -7.554893095320830199, -26.44255681430371396, 22.11862154216139942 ) ) ;
#25038=ORIENTED_EDGE ( 'NONE', *, *, #4217, .T. ) ;
#25049=AXIS2_PLACEMENT_3D ( 'NONE', #16462, #26076, #16922 ) ;
#25050=CARTESIAN_POINT ( 'NONE',  ( 9.736208184377293406, -25.71890933281309444, 204.0979242502758666 ) ) ;
#25052=ORIENTED_EDGE ( 'NONE', *, *, #10234, .F. ) ;
#25070=ORIENTED_EDGE ( 'NONE', *, *, #22251, .T. ) ;
#25078=VERTEX_POINT ( 'NONE', #14775 ) ;
#25088=CARTESIAN_POINT ( 'NONE',  ( -27.50000000000000000, 3.367667473009999970E-15, 193.2809019210000088 ) ) ;
#25094=CARTESIAN_POINT ( 'NONE',  ( -27.23548387100000312, 8.881784196999999612E-15, 41.66046017469999896 ) ) ;
#25101=CARTESIAN_POINT ( 'NONE',  ( -9.543143524407900813, -25.04338540923419743, 203.8394562065719811 ) ) ;
#25104=CARTESIAN_POINT ( 'NONE',  ( 22.63992238019999803, -14.34133587289999845, 225.0000000000000000 ) ) ;
#25109=CARTESIAN_POINT ( 'NONE',  ( -4.433903769297805830, -26.43189459824145615, 20.40472646930128775 ) ) ;
#25122=DIRECTION ( 'NONE',  ( 1.000000000000000000, 0.000000000000000000, 0.000000000000000000 ) ) ;
#25124=CARTESIAN_POINT ( 'NONE',  ( 9.993285220779439371, -25.61999708228226069, 186.3944487260000074 ) ) ;
#25125=DIRECTION ( 'NONE',  ( 1.000000000000000000, 0.000000000000000000, 0.000000000000000000 ) ) ;
#25127=CARTESIAN_POINT ( 'NONE',  ( 0.000000000000000000, 0.000000000000000000, 210.0000000000000284 ) ) ;
#25140=PRODUCT_DEFINITION_SHAPE ( 'NONE', 'NONE',  #5604 ) ;
#25141=CARTESIAN_POINT ( 'NONE',  ( -2.947640775130000104E-14, -27.50000000000000000, 210.0000000000000284 ) ) ;
#25154=EDGE_CURVE ( 'NONE', #12078, #13677, #21554, .T. ) ;
#25158=DIRECTION ( 'NONE',  ( 0.000000000000000000, 0.000000000000000000, -1.000000000000000000 ) ) ;
#25161=CARTESIAN_POINT ( 'NONE',  ( -27.54391550599999761, 3.373045393779999685E-15, 87.04374668509998969 ) ) ;
#25163=CARTESIAN_POINT ( 'NONE',  ( -0.4949169567396824454, -27.49533956265154799, 4.006901989143670129 ) ) ;
#25174=CARTESIAN_POINT ( 'NONE',  ( 0.000000000000000000, 3.552713678799999608E-15, 191.6604601750000256 ) ) ;
#25178=DIRECTION ( 'NONE',  ( -1.000000000000000000, 5.665498452320000818E-16, 0.000000000000000000 ) ) ;
#25180=ORIENTED_EDGE ( 'NONE', *, *, #19270, .T. ) ;
#25183=CARTESIAN_POINT ( 'NONE',  ( -8.903108651239966420, -22.82508830966961000, 140.0000000000000000 ) ) ;
#25189=CARTESIAN_POINT ( 'NONE',  ( -9.736208184377284525, -25.71890933281309444, 25.90207574972422577 ) ) ;
#25190=ORIENTED_EDGE ( 'NONE', *, *, #25937, .F. ) ;
#25191=ORIENTED_EDGE ( 'NONE', *, *, #26202, .T. ) ;
#25195=DIRECTION ( 'NONE',  ( 1.000000000000000000, 0.000000000000000000, 0.000000000000000000 ) ) ;
#25201=CARTESIAN_POINT ( 'NONE',  ( 9.219833965033643608, -25.90918750570072859, 205.5784319129419657 ) ) ;
#25202=CARTESIAN_POINT ( 'NONE',  ( -27.15000000039999861, 3.324806250669999651E-15, 0.000000000000000000 ) ) ;
#25211=CARTESIAN_POINT ( 'NONE',  ( -27.63177356790000161, 3.383804547869999678E-15, 137.3605236429999934 ) ) ;
#25217=CARTESIAN_POINT ( 'NONE',  ( 24.33346004066275370, -12.81155130655225705, 224.7132485887567839 ) ) ;
#25235=SURFACE_STYLE_FILL_AREA ( #20196 ) ;
#25237=CARTESIAN_POINT ( 'NONE',  ( 9.993285220779503319, -25.61999708228222872, 193.6055512739999926 ) ) ;
#25259=CARTESIAN_POINT ( 'NONE',  ( 0.000000000000000000, 0.000000000000000000, 40.00000000000000000 ) ) ;
#25262=CARTESIAN_POINT ( 'NONE',  ( 23.06578384731929532, -13.64653153667426544, 223.9278743037292543 ) ) ;
#25271=DIRECTION ( 'NONE',  ( 0.000000000000000000, 0.000000000000000000, 1.000000000000000000 ) ) ;
#25274=ORIENTED_EDGE ( 'NONE', *, *, #27749, .T. ) ;
#25282=LINE ( 'NONE', #4036, #998 ) ;
#25285=CARTESIAN_POINT ( 'NONE',  ( 26.80000000000000071, 7.105427357599999217E-15, 36.78285841090000474 ) ) ;
#25290=DIRECTION ( 'NONE',  ( 0.3633921898465272138, -0.9316362575375356503, -4.625929269271483744E-15 ) ) ;
#25302=DIRECTION ( 'NONE',  ( 1.000000000000000000, 0.000000000000000000, 0.000000000000000000 ) ) ;
#25303=CARTESIAN_POINT ( 'NONE',  ( 6.726015838937449587, -25.94607852067420595, 208.3934793376300547 ) ) ;
#25322=CARTESIAN_POINT ( 'NONE',  ( -0.8471243407022264194, -27.48706736360457015, 4.296916151638034975 ) ) ;
#25338=CIRCLE ( 'NONE', #19322, 3.000000000000001332 ) ;
#25342=ORIENTED_EDGE ( 'NONE', *, *, #23946, .F. ) ;
#25345=DIRECTION ( 'NONE',  ( 0.000000000000000000, 0.000000000000000000, -1.000000000000000000 ) ) ;
#25347=ORIENTED_EDGE ( 'NONE', *, *, #20417, .T. ) ;
#25355=VERTEX_POINT ( 'NONE', #12067 ) ;
#25363=CARTESIAN_POINT ( 'NONE',  ( 0.000000000000000000, 0.000000000000000000, 115.0000000000000000 ) ) ;
#25366=FACE_OUTER_BOUND ( 'NONE', #4949, .T. ) ;
#25367=CARTESIAN_POINT ( 'NONE',  ( 2.107992564109752998, -27.41908764619381245, 210.0000000000000284 ) ) ;
#25374=CARTESIAN_POINT ( 'NONE',  ( -3.938336462418404516, -27.21777852796477504, 209.8041027071180338 ) ) ;
#25383=CARTESIAN_POINT ( 'NONE',  ( 0.000000000000000000, 0.000000000000000000, 115.0000000000000000 ) ) ;
#25385=VERTEX_POINT ( 'NONE', #26543 ) ;
#25397=VERTEX_POINT ( 'NONE', #12215 ) ;
#25408=EDGE_CURVE ( 'NONE', #25870, #11151, #9552, .T. ) ;
#25410=FACE_OUTER_BOUND ( 'NONE', #24040, .T. ) ;
#25429=CARTESIAN_POINT ( 'NONE',  ( 22.92720033239275068, -13.87810118103447543, 224.0393715186460213 ) ) ;
#25441=ORIENTED_EDGE ( 'NONE', *, *, #16079, .F. ) ;
#25461=FACE_OUTER_BOUND ( 'NONE', #2525, .T. ) ;
#25472=VERTEX_POINT ( 'NONE', #15776 ) ;
#25475=SHAPE_DEFINITION_REPRESENTATION ( #25140, #19621 ) ;
#25477=ORIENTED_EDGE ( 'NONE', *, *, #10860, .T. ) ;
#25481=TOROIDAL_SURFACE ( 'NONE', #11907, 30.50000000000000000, 3.000000000000000000 ) ;
#25485=DIRECTION ( 'NONE',  ( 1.000000000000000000, 0.000000000000000000, 0.000000000000000000 ) ) ;
#25498=CARTESIAN_POINT ( 'NONE',  ( -23.48532358956344623, -12.91116100318319937, 4.042547419098327488 ) ) ;
#25503=CARTESIAN_POINT ( 'NONE',  ( 10.14902473071355793, -26.01926976408357817, 92.06031501460000754 ) ) ;
#25505=AXIS2_PLACEMENT_3D ( 'NONE', #9250, #21222, #16343 ) ;
#25506=CARTESIAN_POINT ( 'NONE',  ( -23.20948082139999968, -13.40000000000000036, 223.8999999999999773 ) ) ;
#25509=ORIENTED_EDGE ( 'NONE', *, *, #30008, .T. ) ;
#25511=DIRECTION ( 'NONE',  ( 0.3633921898465273803, -0.9316362575375355393, 0.000000000000000000 ) ) ;
#25512=ORIENTED_EDGE ( 'NONE', *, *, #6981, .T. ) ;
#25513=ORIENTED_EDGE ( 'NONE', *, *, #18281, .F. ) ;
#25515=EDGE_LOOP ( 'NONE', ( #6553, #23050, #3380, #9282, #21243 ) ) ;
#25529=CARTESIAN_POINT ( 'NONE',  ( -9.509259942401930843, -25.80376675868339120, 204.8434573210849692 ) ) ;
#25535=CARTESIAN_POINT ( 'NONE',  ( -1.841797396446221979, -26.73663745407121795, 20.00000000000000355 ) ) ;
#25537=CARTESIAN_POINT ( 'NONE',  ( 24.34663841809999951, -12.78636765230000094, 225.0000000000000000 ) ) ;
#25542=CARTESIAN_POINT ( 'NONE',  ( -18.95046173579999760, -18.95046173579999760, 36.78285841159999592 ) ) ;
#25546=VERTEX_POINT ( 'NONE', #2251 ) ;
#25551=ORIENTED_EDGE ( 'NONE', *, *, #28292, .T. ) ;
#25552=AXIS2_PLACEMENT_3D ( 'NONE', #9286, #7244, #16837 ) ;
#25565=EDGE_CURVE ( 'NONE', #28783, #15300, #4911, .T. ) ;
#25567=CIRCLE ( 'NONE', #2454, 2.999999999999999556 ) ;
#25569=CARTESIAN_POINT ( 'NONE',  ( 21.30888436558567633, -16.34772642260384856, 136.7828584119999960 ) ) ;
#25570=FACE_OUTER_BOUND ( 'NONE', #18951, .T. ) ;
#25573=CARTESIAN_POINT ( 'NONE',  ( -22.68367506360150188, -14.27296989836904828, 4.579417935583666832 ) ) ;
#25576=CARTESIAN_POINT ( 'NONE',  ( 22.78048776663572639, -14.11708351801274297, 4.280684603339811822 ) ) ;
#25577=CARTESIAN_POINT ( 'NONE',  ( -2.947640775130000104E-14, -27.50000000000000000, 0.000000000000000000 ) ) ;
#25578=CIRCLE ( 'NONE', #19556, 3.200000000000002398 ) ;
#25581=ORIENTED_EDGE ( 'NONE', *, *, #21634, .F. ) ;
#25596=VERTEX_POINT ( 'NONE', #24421 ) ;
#25598=ORIENTED_EDGE ( 'NONE', *, *, #5167, .F. ) ;
#25609=DIRECTION ( 'NONE',  ( 0.9316362575375356503, 0.3633921898465274913, 0.000000000000000000 ) ) ;
#25612=ORIENTED_EDGE ( 'NONE', *, *, #16742, .F. ) ;
#25614=CARTESIAN_POINT ( 'NONE',  ( 27.50000000000000000, -1.776356839399999804E-15, 136.3944487250000179 ) ) ;
#25625=AXIS2_PLACEMENT_3D ( 'NONE', #28575, #7170, #18811 ) ;
#25631=CARTESIAN_POINT ( 'NONE',  ( -2.947640775130000104E-14, -27.50000000000000000, 115.0000000000000000 ) ) ;
#25635=ORIENTED_EDGE ( 'NONE', *, *, #10860, .F. ) ;
#25637=VERTEX_POINT ( 'NONE', #515 ) ;
#25641=VERTEX_POINT ( 'NONE', #7872 ) ;
#25651=CARTESIAN_POINT ( 'NONE',  ( 26.80000000069999899, -3.281945028320000125E-15, 136.7828584130000138 ) ) ;
#25652=EDGE_CURVE ( 'NONE', #17294, #2824, #15576, .T. ) ;
#25666=CARTESIAN_POINT ( 'NONE',  ( 27.50000000000000000, -3.367667472999999580E-15, 193.6055512739999926 ) ) ;
#25671=ORIENTED_EDGE ( 'NONE', *, *, #26012, .T. ) ;
#25679=DIRECTION ( 'NONE',  ( 1.224606353819999829E-16, 1.000000000000000000, 0.000000000000000000 ) ) ;
#25680=CYLINDRICAL_SURFACE ( 'NONE', #15953, 27.50000000000000000 ) ;
#25683=EDGE_CURVE ( 'NONE', #25887, #27542, #4219, .T. ) ;
#25698=DIRECTION ( 'NONE',  ( 0.000000000000000000, 0.000000000000000000, 1.000000000000000000 ) ) ;
#25711=ADVANCED_FACE ( 'NONE', ( #29594 ), #9218, .F. ) ;
#25718=CARTESIAN_POINT ( 'NONE',  ( 23.24663841809999809, -14.69162354060000020, 5.000000000000000000 ) ) ;
#25721=CARTESIAN_POINT ( 'NONE',  ( -0.8784916636842051707, -26.78562594404069230, 224.3339239247088699 ) ) ;
#25727=CARTESIAN_POINT ( 'NONE',  ( 9.993285220779439371, -25.61999708228226069, 115.0000000000000000 ) ) ;
#25740=DIRECTION ( 'NONE',  ( 1.000000000000000000, 0.000000000000000000, 0.000000000000000000 ) ) ;
#25745=EDGE_CURVE ( 'NONE', #12912, #17381, #29834, .T. ) ;
#25750=DIRECTION ( 'NONE',  ( -0.9316362575375349842, 0.3633921898465292122, -0.000000000000000000 ) ) ;
#25766=ORIENTED_EDGE ( 'NONE', *, *, #6167, .F. ) ;
#25774=DIRECTION ( 'NONE',  ( 0.3633921898465292122, 0.9316362575375348731, -6.938893903907226800E-15 ) ) ;
#25777=CARTESIAN_POINT ( 'NONE',  ( -23.48807013383927256, -14.30280389769410831, 5.913085275914951922 ) ) ;
#25781=EDGE_CURVE ( 'NONE', #28478, #2098, #970, .T. ) ;
#25791=ORIENTED_EDGE ( 'NONE', *, *, #3028, .T. ) ;
#25792=ADVANCED_FACE ( 'NONE', ( #30057 ), #8488, .F. ) ;
#25799=FACE_OUTER_BOUND ( 'NONE', #8265, .T. ) ;
#25804=ORIENTED_EDGE ( 'NONE', *, *, #20055, .T. ) ;
#25805=CARTESIAN_POINT ( 'NONE',  ( 0.000000000000000000, 0.000000000000000000, 115.0000000000000000 ) ) ;
#25812=CARTESIAN_POINT ( 'NONE',  ( -8.903108651239966420, -22.82508830966961000, 190.0000000000000000 ) ) ;
#25814=CARTESIAN_POINT ( 'NONE',  ( -23.28322851814834493, -13.27226524233089933, 3.900000000000000799 ) ) ;
#25819=ORIENTED_EDGE ( 'NONE', *, *, #7371, .T. ) ;
#25820=AXIS2_PLACEMENT_3D ( 'NONE', #7804, #10488, #17698 ) ;
#25824=EDGE_LOOP ( 'NONE', ( #25342, #11022, #26916, #25513 ) ) ;
#25827=EDGE_CURVE ( 'NONE', #23982, #8812, #23461, .T. ) ;
#25831=VERTEX_POINT ( 'NONE', #1587 ) ;
#25858=VERTEX_POINT ( 'NONE', #25503 ) ;
#25863=EDGE_CURVE ( 'NONE', #26900, #26548, #23321, .T. ) ;
#25864=CARTESIAN_POINT ( 'NONE',  ( 27.23548387060000309, -1.776356839399999804E-15, 138.3395398250000028 ) ) ;
#25866=AXIS2_PLACEMENT_3D ( 'NONE', #30572, #20966, #11677 ) ;
#25867=ORIENTED_EDGE ( 'NONE', *, *, #7156, .F. ) ;
#25870=VERTEX_POINT ( 'NONE', #3941 ) ;
#25880=CARTESIAN_POINT ( 'NONE',  ( -23.64677485492346065, -12.61282739001573994, 5.633487048013353871 ) ) ;
#25884=CARTESIAN_POINT ( 'NONE',  ( -3.552713678799999608E-15, 0.000000000000000000, 93.21714158839999698 ) ) ;
#25887=VERTEX_POINT ( 'NONE', #18716 ) ;
#25890=AXIS2_PLACEMENT_3D ( 'NONE', #4985, #2784, #28598 ) ;
#25893=DIRECTION ( 'NONE',  ( 0.3633921898465291567, 0.9316362575375349842, 0.000000000000000000 ) ) ;
#25899=DIRECTION ( 'NONE',  ( -0.7071067811865475727, -0.7071067811865475727, 0.000000000000000000 ) ) ;
#25901=EDGE_CURVE ( 'NONE', #20382, #12383, #23870, .T. ) ;
#25910=DIRECTION ( 'NONE',  ( 0.3633921898465272138, -0.9316362575375356503, -9.251858538542967489E-15 ) ) ;
#25928=CARTESIAN_POINT ( 'NONE',  ( -0.1455402981285491004, -27.49999999999999289, 226.1000000000000227 ) ) ;
#25937=EDGE_CURVE ( 'NONE', #21389, #11492, #19787, .T. ) ;
#25948=EDGE_CURVE ( 'NONE', #12574, #5207, #10243, .T. ) ;
#25963=CARTESIAN_POINT ( 'NONE',  ( 9.993285220779439371, -25.61999708228226069, 136.3944487260000074 ) ) ;
#25965=CARTESIAN_POINT ( 'NONE',  ( 9.738910687886868089, -24.96785170200598358, 86.78285841159998881 ) ) ;
#25968=CARTESIAN_POINT ( 'NONE',  ( 27.54391550559999757, -3.373045393719999713E-15, 187.0437466829999948 ) ) ;
#25977=ORIENTED_EDGE ( 'NONE', *, *, #31035, .F. ) ;
#25981=EDGE_LOOP ( 'NONE', ( #10115, #22036, #12201, #14676 ) ) ;
#25995=CARTESIAN_POINT ( 'NONE',  ( 0.000000000000000000, 0.000000000000000000, 115.0000000000000000 ) ) ;
#26003=DIRECTION ( 'NONE',  ( 1.000000000000000000, 0.000000000000000000, 0.000000000000000000 ) ) ;
#26008=EDGE_LOOP ( 'NONE', ( #2488, #23505, #17561, #8326, #29683 ) ) ;
#26012=EDGE_CURVE ( 'NONE', #2408, #18020, #10316, .T. ) ;
#26026=VECTOR ( 'NONE', #30626, 1000.000000000000000 ) ;
#26048=ORIENTED_EDGE ( 'NONE', *, *, #19651, .F. ) ;
#26051=AXIS2_PLACEMENT_3D ( 'NONE', #3837, #13423, #16253 ) ;
#26059=ORIENTED_EDGE ( 'NONE', *, *, #18618, .F. ) ;
#26063=EDGE_CURVE ( 'NONE', #4374, #26433, #21873, .T. ) ;
#26064=ORIENTED_EDGE ( 'NONE', *, *, #9901, .F. ) ;
#26065=FACE_OUTER_BOUND ( 'NONE', #30848, .T. ) ;
#26066=TOROIDAL_SURFACE ( 'NONE', #12484, 24.50000000000000000, 3.200000000000000178 ) ;
#26072=CARTESIAN_POINT ( 'NONE',  ( 26.80000000069999899, -3.281945028320000125E-15, 42.88981852279999885 ) ) ;
#26076=DIRECTION ( 'NONE',  ( -1.224606353819999829E-16, -1.000000000000000000, 0.000000000000000000 ) ) ;
#26090=EDGE_LOOP ( 'NONE', ( #6613, #12006, #17025, #16672 ) ) ;
#26091=CARTESIAN_POINT ( 'NONE',  ( -23.81569860410000317, -13.75000000000000000, 223.8999999999999773 ) ) ;
#26113=AXIS2_PLACEMENT_3D ( 'NONE', #9964, #26639, #29298 ) ;
#26123=EDGE_CURVE ( 'NONE', #28953, #5952, #210, .T. ) ;
#26125=CARTESIAN_POINT ( 'NONE',  ( 24.49999999589999788, -3.000285566359999846E-15, 40.00000000000000000 ) ) ;
#26128=DIRECTION ( 'NONE',  ( 0.3090169943750400994, -0.9510565162951234441, 0.000000000000000000 ) ) ;
#26135=CIRCLE ( 'NONE', #20086, 3.200000004570001888 ) ;
#26136=ORIENTED_EDGE ( 'NONE', *, *, #26242, .F. ) ;
#26139=DIRECTION ( 'NONE',  ( 1.000000000000000000, -1.224606353819999582E-16, 0.000000000000000000 ) ) ;
#26145=CARTESIAN_POINT ( 'NONE',  ( -23.13573312441312879, -13.52773475816182369, 6.100000000000007638 ) ) ;
#26147=EDGE_CURVE ( 'NONE', #28386, #8364, #14442, .T. ) ;
#26157=DIRECTION ( 'NONE',  ( 0.3633921898465291567, 0.9316362575375349842, 0.000000000000000000 ) ) ;
#26159=CIRCLE ( 'NONE', #28668, 27.92857142860000152 ) ;
#26163=EDGE_LOOP ( 'NONE', ( #21138, #15624, #18053, #29959, #942 ) ) ;
#26164=CARTESIAN_POINT ( 'NONE',  ( 23.53263993737497017, -14.22965940669009655, 5.959546603885336857 ) ) ;
#26174=VERTEX_POINT ( 'NONE', #22327 ) ;
#26187=CARTESIAN_POINT ( 'NONE',  ( 1.100000000000000089, -27.47799119230000287, 5.000000000000000000 ) ) ;
#26189=LINE ( 'NONE', #13758, #18707 ) ;
#26193=CARTESIAN_POINT ( 'NONE',  ( -10.82908725742657374, -27.76276047461854546, 143.2171415880000040 ) ) ;
#26197=ORIENTED_EDGE ( 'NONE', *, *, #5058, .F. ) ;
#26202=EDGE_CURVE ( 'NONE', #14673, #5141, #17816, .T. ) ;
#26238=ORIENTED_EDGE ( 'NONE', *, *, #15780, .T. ) ;
#26242=EDGE_CURVE ( 'NONE', #15285, #17294, #15864, .T. ) ;
#26246=TOROIDAL_SURFACE ( 'NONE', #16685, 24.50000000000000000, 4.000000000000000000 ) ;
#26248=VERTEX_POINT ( 'NONE', #30658 ) ;
#26251=ORIENTED_EDGE ( 'NONE', *, *, #20172, .F. ) ;
#26270=CARTESIAN_POINT ( 'NONE',  ( 11.08346179031908640, -28.41490585489483678, 93.60555127549999099 ) ) ;
#26277=DIRECTION ( 'NONE',  ( 0.000000000000000000, 0.000000000000000000, -1.000000000000000000 ) ) ;
#26279=CARTESIAN_POINT ( 'NONE',  ( -21.30888436558564791, -16.34772642260388409, 186.7828584121667177 ) ) ;
#26281=ORIENTED_EDGE ( 'NONE', *, *, #7883, .T. ) ;
#26300=FACE_OUTER_BOUND ( 'NONE', #3154, .T. ) ;
#26301=CARTESIAN_POINT ( 'NONE',  ( 23.73992238019999945, -12.43607998449999918, 225.0000000000000000 ) ) ;
#26311=DIRECTION ( 'NONE',  ( 1.000000000000000000, -1.224606353820000075E-16, 0.000000000000000000 ) ) ;
#26329=AXIS2_PLACEMENT_3D ( 'NONE', #27388, #24882, #5982 ) ;
#26343=DIRECTION ( 'NONE',  ( -0.3090169943750401549, -0.9510565162951233331, 0.000000000000000000 ) ) ;
#26354=ORIENTED_EDGE ( 'NONE', *, *, #13862, .T. ) ;
#26362=EDGE_CURVE ( 'NONE', #24890, #25397, #10693, .T. ) ;
#26363=ORIENTED_EDGE ( 'NONE', *, *, #22789, .T. ) ;
#26366=ORIENTED_EDGE ( 'NONE', *, *, #16214, .F. ) ;
#26369=ORIENTED_EDGE ( 'NONE', *, *, #26063, .F. ) ;
#26372=EDGE_CURVE ( 'NONE', #26433, #21744, #8796, .T. ) ;
#26375=DIRECTION ( 'NONE',  ( 1.000000000000000000, 0.000000000000000000, 0.000000000000000000 ) ) ;
#26376=AXIS2_PLACEMENT_3D ( 'NONE', #8210, #27271, #22562 ) ;
#26377=CARTESIAN_POINT ( 'NONE',  ( 1.071601127087828287, -27.47917021045937958, 224.7132485889944746 ) ) ;
#26379=AXIS2_PLACEMENT_3D ( 'NONE', #4288, #1929, #30247 ) ;
#26399=AXIS2_PLACEMENT_3D ( 'NONE', #19548, #21917, #22214 ) ;
#26407=ORIENTED_EDGE ( 'NONE', *, *, #27163, .F. ) ;
#26415=DIRECTION ( 'NONE',  ( -5.551115123130000150E-16, -1.000000000000000000, 0.000000000000000000 ) ) ;
#26419=DIRECTION ( 'NONE',  ( 0.000000000000000000, 0.000000000000000000, 1.000000000000000000 ) ) ;
#26423=B_SPLINE_CURVE_WITH_KNOTS ( 'NONE', 3,
 ( #30233, #6625, #20795, #18263, #28183, #11510, #1294, #1454, #13230, #30405 ),
 .UNSPECIFIED., .F., .F.,
 ( 4, 2, 2, 2, 4 ),
 ( 0.000000000000000000, 0.2500000000000000555, 0.5000000000000000000, 0.7499999999999998890, 1.000000000000000000 ),
 .UNSPECIFIED. ) ;
#26425=ADVANCED_FACE ( 'NONE', ( #14440 ), #11259, .F. ) ;
#26433=VERTEX_POINT ( 'NONE', #9555 ) ;
#26439=ORIENTED_EDGE ( 'NONE', *, *, #9712, .F. ) ;
#26444=ORIENTED_EDGE ( 'NONE', *, *, #27509, .T. ) ;
#26446=CARTESIAN_POINT ( 'NONE',  ( 3.552713678799999608E-15, -3.552713678799999608E-15, 186.7828584120000244 ) ) ;
#26458=EDGE_CURVE ( 'NONE', #7727, #12643, #21812, .T. ) ;
#26461=CARTESIAN_POINT ( 'NONE',  ( -23.56630063319272139, -14.17280417015954619, 225.9948832298492221 ) ) ;
#26469=ORIENTED_EDGE ( 'NONE', *, *, #23556, .T. ) ;
#26470=CARTESIAN_POINT ( 'NONE',  ( 23.36339467984016594, -14.50559736741132433, 5.674968348874030788 ) ) ;
#26496=CARTESIAN_POINT ( 'NONE',  ( 23.20948082139999968, -13.40000000000000036, 6.099999999630000502 ) ) ;
#26499=PLANE ( 'NONE',  #2694 ) ;
#26505=FACE_OUTER_BOUND ( 'NONE', #26695, .T. ) ;
#26511=AXIS2_PLACEMENT_3D ( 'NONE', #9409, #5148, #21693 ) ;
#26533=CIRCLE ( 'NONE', #19503, 4.000000000000000888 ) ;
#26535=DIRECTION ( 'NONE',  ( 1.000000000000000000, 0.000000000000000000, 0.000000000000000000 ) ) ;
#26539=CARTESIAN_POINT ( 'NONE',  ( -0.9003584917538117738, -26.78512143702961268, 225.6334870514607189 ) ) ;
#26540=FACE_BOUND ( 'NONE', #2625, .T. ) ;
#26543=CARTESIAN_POINT ( 'NONE',  ( -27.50000000000000000, 0.000000000000000000, 143.6055512749999821 ) ) ;
#26545=ORIENTED_EDGE ( 'NONE', *, *, #30762, .F. ) ;
#26548=VERTEX_POINT ( 'NONE', #2786 ) ;
#26552=ORIENTED_EDGE ( 'NONE', *, *, #20592, .F. ) ;
#26568=EDGE_CURVE ( 'NONE', #10260, #23969, #21792, .T. ) ;
#26579=CARTESIAN_POINT ( 'NONE',  ( 0.8178280466645336810, -26.78758467633450735, 224.2627730065052560 ) ) ;
#26581=CIRCLE ( 'NONE', #13000, 27.69999999999999929 ) ;
#26583=CARTESIAN_POINT ( 'NONE',  ( 2.895630725101784542, -26.64812433595226437, 20.04809298185875832 ) ) ;
#26588=CARTESIAN_POINT ( 'NONE',  ( 23.88846875300728456, -13.62395840476969688, 3.900000000370010156 ) ) ;
#26597=CARTESIAN_POINT ( 'NONE',  ( -24.49999999470000134, 3.000285566209999917E-15, 39.99999999930000172 ) ) ;
#26612=CARTESIAN_POINT ( 'NONE',  ( 4.941595660341814522, -27.05346828916501423, 20.49141012103500259 ) ) ;
#26616=CARTESIAN_POINT ( 'NONE',  ( 0.000000000000000000, 0.000000000000000000, 92.06031501460000754 ) ) ;
#26621=ORIENTED_EDGE ( 'NONE', *, *, #24267, .F. ) ;
#26623=CARTESIAN_POINT ( 'NONE',  ( 23.47117976014261131, -14.33053685730250493, 5.880491002250007426 ) ) ;
#26629=EDGE_CURVE ( 'NONE', #11773, #11717, #6218, .T. ) ;
#26638=FACE_OUTER_BOUND ( 'NONE', #15783, .T. ) ;
#26639=DIRECTION ( 'NONE',  ( 0.000000000000000000, 0.000000000000000000, 1.000000000000000000 ) ) ;
#26641=ORIENTED_EDGE ( 'NONE', *, *, #6549, .T. ) ;
#26643=CIRCLE ( 'NONE', #30074, 3.200000004570001888 ) ;
#26646=CARTESIAN_POINT ( 'NONE',  ( 0.2195862974910302301, -27.49906791309039633, 6.087643466945557691 ) ) ;
#26647=DIRECTION ( 'NONE',  ( 1.224606353819999829E-16, 1.000000000000000000, 0.000000000000000000 ) ) ;
#26649=CARTESIAN_POINT ( 'NONE',  ( 26.93395387809999875, -3.298349105250000085E-15, 92.24324102360000666 ) ) ;
#26652=CARTESIAN_POINT ( 'NONE',  ( -27.23548387180000319, 3.335274659879999868E-15, 88.33953982590000464 ) ) ;
#26660=ORIENTED_EDGE ( 'NONE', *, *, #10289, .T. ) ;
#26678=CARTESIAN_POINT ( 'NONE',  ( 13.11056599509670129, -23.44705117439652042, 36.78285841135431156 ) ) ;
#26680=CARTESIAN_POINT ( 'NONE',  ( 23.31771987772114940, -13.21065015143701693, 223.9123094306712005 ) ) ;
#26685=CARTESIAN_POINT ( 'NONE',  ( -9.897162125297922941, -25.37356426550855204, 141.6604601749999972 ) ) ;
#26692=DIRECTION ( 'NONE',  ( 0.3633921898465273803, -0.9316362575375355393, 0.000000000000000000 ) ) ;
#26695=EDGE_LOOP ( 'NONE', ( #6026, #21, #21605, #13212 ) ) ;
#26702=DIRECTION ( 'NONE',  ( 0.3633921898465291567, 0.9316362575375349842, 0.000000000000000000 ) ) ;
#26703=EDGE_LOOP ( 'NONE', ( #5986, #15906, #25180, #1282, #4917, #1751, #20623, #489, #13629, #4774 ) ) ;
#26705=ORIENTED_EDGE ( 'NONE', *, *, #25901, .F. ) ;
#26710=AXIS2_PLACEMENT_3D ( 'NONE', #25174, #3301, #12906 ) ;
#26712=CARTESIAN_POINT ( 'NONE',  ( 27.54391550599999761, -3.373045393770000084E-15, 87.04374668499998791 ) ) ;
#26720=CARTESIAN_POINT ( 'NONE',  ( 1.100000000000000089, -17.25771824079999917, 225.0000000000000000 ) ) ;
#26730=AXIS2_PLACEMENT_3D ( 'NONE', #27482, #2160, #14117 ) ;
#26739=EDGE_CURVE ( 'NONE', #16404, #4771, #27822, .T. ) ;
#26746=DIRECTION ( 'NONE',  ( 1.224606353819999829E-16, 1.000000000000000000, 0.000000000000000000 ) ) ;
#26772=ORIENTED_EDGE ( 'NONE', *, *, #9018, .F. ) ;
#26774=DIRECTION ( 'NONE',  ( -0.8660254037843290176, 0.5000000000001899592, 0.000000000000000000 ) ) ;
#26778=EDGE_LOOP ( 'NONE', ( #5081, #10482, #160, #24479 ) ) ;
#26792=TOROIDAL_SURFACE ( 'NONE', #30326, 24.50000000000000000, 4.000000000000000000 ) ;
#26796=EDGE_CURVE ( 'NONE', #12383, #11948, #21817, .T. ) ;
#26797=CARTESIAN_POINT ( 'NONE',  ( -27.50000000000000000, 0.000000000000000000, 143.6055512749999821 ) ) ;
#26817=AXIS2_PLACEMENT_3D ( 'NONE', #13304, #22914, #4178 ) ;
#26818=EDGE_LOOP ( 'NONE', ( #29538, #10110, #12850, #7582 ) ) ;
#26819=DIRECTION ( 'NONE',  ( 1.000000000000000000, 0.000000000000000000, 0.000000000000000000 ) ) ;
#26821=ORIENTED_EDGE ( 'NONE', *, *, #29581, .F. ) ;
#26843=CARTESIAN_POINT ( 'NONE',  ( -1.033595436889999888E-13, -27.50000000069999828, 3.899999999999999911 ) ) ;
#26850=CARTESIAN_POINT ( 'NONE',  ( 0.000000000000000000, 0.000000000000000000, 143.6055512739999926 ) ) ;
#26863=CIRCLE ( 'NONE', #10221, 3.000000000000001332 ) ;
#26888=CARTESIAN_POINT ( 'NONE',  ( -27.23548387060000309, 7.105427357599999217E-15, 141.6604601749999972 ) ) ;
#26893=ORIENTED_EDGE ( 'NONE', *, *, #29617, .F. ) ;
#26895=CIRCLE ( 'NONE', #16852, 3.199999983039998774 ) ;
#26900=VERTEX_POINT ( 'NONE', #23698 ) ;
#26908=CARTESIAN_POINT ( 'NONE',  ( -9.993285220779425160, -25.61999708228226069, 115.0000000000000000 ) ) ;
#26912=DIRECTION ( 'NONE',  ( 0.000000000000000000, 0.000000000000000000, -1.000000000000000000 ) ) ;
#26916=ORIENTED_EDGE ( 'NONE', *, *, #6593, .F. ) ;
#26922=EDGE_CURVE ( 'NONE', #7809, #25385, #5100, .T. ) ;
#26928=B_SPLINE_CURVE_WITH_KNOTS ( 'NONE', 3,
 ( #22517, #24875, #29897, #8638, #23141, #15723, #8323, #3304, #22818, #3937, #30377, #11019 ),
 .UNSPECIFIED., .F., .F.,
 ( 4, 2, 2, 2, 2, 4 ),
 ( 0.000000000000000000, 0.2499999999999976685, 0.3749999999999970579, 0.4999999999999964473, 0.7499999999999982236, 1.000000000000000000 ),
 .UNSPECIFIED. ) ;
#26941=ORIENTED_EDGE ( 'NONE', *, *, #28269, .F. ) ;
#26943=ORIENTED_EDGE ( 'NONE', *, *, #9375, .F. ) ;
#26945=EDGE_CURVE ( 'NONE', #27983, #24427, #13236, .T. ) ;
#26946=DIRECTION ( 'NONE',  ( 0.000000000000000000, 1.000000000000000000, 0.000000000000000000 ) ) ;
#26948=ORIENTED_EDGE ( 'NONE', *, *, #5279, .F. ) ;
#26949=DIRECTION ( 'NONE',  ( 1.000000000000000000, 0.000000000000000000, 0.000000000000000000 ) ) ;
#26961=CARTESIAN_POINT ( 'NONE',  ( 26.80000000069999899, -3.281945028320000125E-15, 192.8898184869999852 ) ) ;
#26962=EDGE_CURVE ( 'NONE', #29126, #19505, #3899, .T. ) ;
#26979=CARTESIAN_POINT ( 'NONE',  ( -10.14902473063359167, -26.01926976387843027, 192.0603150150000147 ) ) ;
#26982=DIRECTION ( 'NONE',  ( 0.000000000000000000, 0.000000000000000000, -1.000000000000000000 ) ) ;
#26984=ADVANCED_FACE ( 'NONE', ( #3990 ), #8730, .T. ) ;
#26985=CARTESIAN_POINT ( 'NONE',  ( 23.20948082139999968, -13.40000000000000036, 226.0999999999999943 ) ) ;
#26990=EDGE_LOOP ( 'NONE', ( #15512, #16587, #26705, #28368 ) ) ;
#26996=CARTESIAN_POINT ( 'NONE',  ( -1.841797396446221091, -26.73663745407121795, 210.0000000000000284 ) ) ;
#26999=CARTESIAN_POINT ( 'NONE',  ( 0.6812178525677142771, -27.49175526060846408, 4.123857012729932769 ) ) ;
#27003=AXIS2_PLACEMENT_3D ( 'NONE', #5922, #607, #12545 ) ;
#27004=CARTESIAN_POINT ( 'NONE',  ( -5.159343048259773745, -26.29982486972314604, 20.68509006311345644 ) ) ;
#27016=ADVANCED_FACE ( 'NONE', ( #11385 ), #6713, .T. ) ;
#27017=ORIENTED_EDGE ( 'NONE', *, *, #27674, .T. ) ;
#27021=CARTESIAN_POINT ( 'NONE',  ( -20.19076655603533155, -17.71015691556361205, 143.2171415880000040 ) ) ;
#27022=AXIS2_PLACEMENT_3D ( 'NONE', #22572, #15628, #10303 ) ;
#27023=B_SPLINE_CURVE_WITH_KNOTS ( 'NONE', 5,
 ( #13834, #6588, #23446, #3765, #13993, #30673 ),
 .UNSPECIFIED., .F., .F.,
 ( 6, 6 ),
 ( -2.300779653509999800, 0.000000000000000000 ),
 .UNSPECIFIED. ) ;
#27025=FACE_OUTER_BOUND ( 'NONE', #4880, .T. ) ;
#27038=CARTESIAN_POINT ( 'NONE',  ( -27.92857142860000152, 1.776356839399999804E-15, 37.93968498539999956 ) ) ;
#27041=DIRECTION ( 'NONE',  ( -0.8090169943751909232, 0.5877852522921378498, 0.000000000000000000 ) ) ;
#27047=CIRCLE ( 'NONE', #30589, 26.80000000000000071 ) ;
#27058=FACE_BOUND ( 'NONE', #10447, .T. ) ;
#27060=CIRCLE ( 'NONE', #17986, 27.92857142860000152 ) ;
#27064=CARTESIAN_POINT ( 'NONE',  ( -27.63177371549999961, 3.383804565940000193E-15, 42.63947604850000772 ) ) ;
#27065=CIRCLE ( 'NONE', #22049, 26.80000000000000071 ) ;
#27076=EDGE_CURVE ( 'NONE', #10071, #25355, #17375, .T. ) ;
#27081=EDGE_CURVE ( 'NONE', #27427, #22997, #13771, .T. ) ;
#27085=ORIENTED_EDGE ( 'NONE', *, *, #668, .F. ) ;
#27095=AXIS2_PLACEMENT_3D ( 'NONE', #25259, #3691, #13293 ) ;
#27102=CARTESIAN_POINT ( 'NONE',  ( 4.933588760076037971, -27.05494253741616362, 209.5115863151182793 ) ) ;
#27103=EDGE_CURVE ( 'NONE', #29126, #2375, #9531, .T. ) ;
#27108=CARTESIAN_POINT ( 'NONE',  ( -26.79999999999999361, -1.754055898254257118, 193.2171415879999756 ) ) ;
#27113=MECHANICAL_DESIGN_GEOMETRIC_PRESENTATION_REPRESENTATION('',(#6515),#29625);
#27137=B_SPLINE_CURVE_WITH_KNOTS ( 'NONE', 3,
 ( #6939, #5044, #21263, #21895, #14653, #4578, #24238, #2683, #9925, #12278, #26145, #342 ),
 .UNSPECIFIED., .F., .F.,
 ( 4, 2, 2, 2, 2, 4 ),
 ( 0.000000000000000000, 0.2500000000000012212, 0.3750000000000017208, 0.5000000000000022204, 0.7500000000000011102, 1.000000000000000000 ),
 .UNSPECIFIED. ) ;
#27140=CARTESIAN_POINT ( 'NONE',  ( 9.897162125286889989, -25.37356426548040389, 188.3395398250000028 ) ) ;
#27144=CARTESIAN_POINT ( 'NONE',  ( -24.49999999589999788, 3.000285566369999841E-15, 90.00000000000000000 ) ) ;
#27151=CARTESIAN_POINT ( 'NONE',  ( -23.24663841809999809, -14.69162354060000020, 5.000000000000000000 ) ) ;
#27152=CIRCLE ( 'NONE', #29664, 27.23548387080000310 ) ;
#27158=DIRECTION ( 'NONE',  ( 0.000000000000000000, 0.000000000000000000, 1.000000000000000000 ) ) ;
#27159=CARTESIAN_POINT ( 'NONE',  ( -8.158046243928263053, -25.52871334855630892, 23.09233687717909334 ) ) ;
#27160=CARTESIAN_POINT ( 'NONE',  ( 0.000000000000000000, 0.000000000000000000, 115.0000000000000000 ) ) ;
#27163=EDGE_CURVE ( 'NONE', #10568, #19354, #3122, .T. ) ;
#27168=ORIENTED_EDGE ( 'NONE', *, *, #8132, .T. ) ;
#27182=VECTOR ( 'NONE', #17851, 1000.000000000000000 ) ;
#27195=CARTESIAN_POINT ( 'NONE',  ( -24.76521256262104842, -10.24325429074770000, 43.21714158839976250 ) ) ;
#27197=CARTESIAN_POINT ( 'NONE',  ( 7.838355892653583012, -25.63086664713628693, 22.66947412054902244 ) ) ;
#27211=CARTESIAN_POINT ( 'NONE',  ( 0.000000000000000000, 0.000000000000000000, 137.9396849850000137 ) ) ;
#27217=DIRECTION ( 'NONE',  ( 0.000000000000000000, 0.000000000000000000, 1.000000000000000000 ) ) ;
#27218=CARTESIAN_POINT ( 'NONE',  ( 8.903108651239925564, -22.82508830966962421, 190.0000000000000000 ) ) ;
#27230=ADVANCED_FACE ( 'NONE', ( #29865, #18051 ), #22331, .F. ) ;
#27234=ORIENTED_EDGE ( 'NONE', *, *, #26568, .T. ) ;
#27236=DIRECTION ( 'NONE',  ( 0.000000000000000000, 0.000000000000000000, 1.000000000000000000 ) ) ;
#27237=EDGE_LOOP ( 'NONE', ( #27814, #7012, #28991, #4415 ) ) ;
#27246=DIRECTION ( 'NONE',  ( 0.000000000000000000, 0.000000000000000000, 1.000000000000000000 ) ) ;
#27268=VERTEX_POINT ( 'NONE', #24993 ) ;
#27271=DIRECTION ( 'NONE',  ( 0.8660254037843290176, 0.5000000000001899592, 1.018673689593249976E-32 ) ) ;
#27277=EDGE_LOOP ( 'NONE', ( #30186, #14071, #5527, #13821, #7512 ) ) ;
#27279=( NAMED_UNIT ( * ) SI_UNIT ( $, .STERADIAN. ) SOLID_ANGLE_UNIT ( ) );
#27284=DIRECTION ( 'NONE',  ( 1.224606353819999829E-16, 1.000000000000000000, 0.000000000000000000 ) ) ;
#27288=CARTESIAN_POINT ( 'NONE',  ( -27.54391552369999729, 3.373045395949999841E-15, 192.9562530129999800 ) ) ;
#27311=CARTESIAN_POINT ( 'NONE',  ( -24.76259292740833828, -10.24958551592170508, 93.21714158839989750 ) ) ;
#27329=DIRECTION ( 'NONE',  ( 0.8090169943751909232, 0.5877852522921378498, 0.000000000000000000 ) ) ;
#27330=AXIS2_PLACEMENT_3D ( 'NONE', #11881, #14095, #11724 ) ;
#27333=DIRECTION ( 'NONE',  ( 0.000000000000000000, 0.000000000000000000, -1.000000000000000000 ) ) ;
#27334=ORIENTED_EDGE ( 'NONE', *, *, #29983, .T. ) ;
#27346=CARTESIAN_POINT ( 'NONE',  ( -25.15951549259922260, -9.235088186050575132, 43.21714158838125996 ) ) ;
#27347=CIRCLE ( 'NONE', #11300, 2.999999999999999556 ) ;
#27350=CARTESIAN_POINT ( 'NONE',  ( 5.395560604220515977, -26.25584002662961680, 20.78043813435757414 ) ) ;
#27351=ORIENTED_EDGE ( 'NONE', *, *, #6167, .T. ) ;
#27360=EDGE_CURVE ( 'NONE', #23263, #9397, #2238, .T. ) ;
#27369=CARTESIAN_POINT ( 'NONE',  ( -18.95046173579999760, -18.95046173579999760, 115.0000000000000000 ) ) ;
#27375=AXIS2_PLACEMENT_3D ( 'NONE', #13931, #23540, #9192 ) ;
#27385=DIRECTION ( 'NONE',  ( 0.000000000000000000, 0.000000000000000000, 1.000000000000000000 ) ) ;
#27388=CARTESIAN_POINT ( 'NONE',  ( 14.94562240850000023, -8.628859120750000500, 5.000000000000000000 ) ) ;
#27393=CARTESIAN_POINT ( 'NONE',  ( -3.928578988383292003, -27.21916582938555251, 20.19379707351126285 ) ) ;
#27395=ORIENTED_EDGE ( 'NONE', *, *, #24737, .F. ) ;
#27399=CARTESIAN_POINT ( 'NONE',  ( 0.000000000000000000, 0.000000000000000000, 190.0000000000000000 ) ) ;
#27403=EDGE_CURVE ( 'NONE', #11023, #29126, #12241, .T. ) ;
#27406=CARTESIAN_POINT ( 'NONE',  ( 8.982833346883268177, -25.99322455654492003, 206.0440937483093649 ) ) ;
#27411=DIRECTION ( 'NONE',  ( 1.000000000000000000, 0.000000000000000000, 0.000000000000000000 ) ) ;
#27418=CARTESIAN_POINT ( 'NONE',  ( 26.80000000000000071, -3.552713678799999608E-15, 93.21714158839999698 ) ) ;
#27427=VERTEX_POINT ( 'NONE', #12864 ) ;
#27428=ORIENTED_EDGE ( 'NONE', *, *, #13702, .T. ) ;
#27430=VERTEX_POINT ( 'NONE', #17269 ) ;
#27432=ORIENTED_EDGE ( 'NONE', *, *, #11856, .T. ) ;
#27458=CARTESIAN_POINT ( 'NONE',  ( -26.62724484483074150, -3.508068424025498455, 93.21714158835001740 ) ) ;
#27459=LINE ( 'NONE', #3081, #24868 ) ;
#27473=CARTESIAN_POINT ( 'NONE',  ( -18.95046173579999760, -18.95046173579999760, 136.7828584120000244 ) ) ;
#27482=CARTESIAN_POINT ( 'NONE',  ( 7.105427357599999217E-15, 3.552713678799999608E-15, 93.60555127549999099 ) ) ;
#27483=CARTESIAN_POINT ( 'NONE',  ( 0.000000000000000000, 0.000000000000000000, 190.0000000000000000 ) ) ;
#27484=AXIS2_PLACEMENT_3D ( 'NONE', #11823, #10082, #7401 ) ;
#27485=LINE ( 'NONE', #24831, #17644 ) ;
#27486=DIRECTION ( 'NONE',  ( -1.000000000000000000, 5.665498452320000818E-16, 0.000000000000000000 ) ) ;
#27489=CARTESIAN_POINT ( 'NONE',  ( 2.373622499810743136, -26.70000180411620505, 210.0000000000000284 ) ) ;
#27494=B_SPLINE_CURVE_WITH_KNOTS ( 'NONE', 5,
 ( #17838, #24783, #15340, #10931, #5735, #24938 ),
 .UNSPECIFIED., .F., .F.,
 ( 6, 6 ),
 ( -2.319814960320000008, 0.000000000000000000 ),
 .UNSPECIFIED. ) ;
#27495=ORIENTED_EDGE ( 'NONE', *, *, #4104, .F. ) ;
#27501=ORIENTED_EDGE ( 'NONE', *, *, #19030, .T. ) ;
#27509=EDGE_CURVE ( 'NONE', #4659, #8882, #6901, .T. ) ;
#27512=CARTESIAN_POINT ( 'NONE',  ( -24.49999999589999788, 3.000285566369999841E-15, 40.00000000000000000 ) ) ;
#27522=CYLINDRICAL_SURFACE ( 'NONE', #20212, 27.50000000000000000 ) ;
#27531=TOROIDAL_SURFACE ( 'NONE', #5414, 29.80000000000000071, 3.000000000000000000 ) ;
#27532=EDGE_CURVE ( 'NONE', #17862, #6732, #12779, .T. ) ;
#27542=VERTEX_POINT ( 'NONE', #6082 ) ;
#27543=CARTESIAN_POINT ( 'NONE',  ( -3.160606383828813204, -27.32265456628853784, 20.04828141274519027 ) ) ;
#27545=EDGE_CURVE ( 'NONE', #25546, #21137, #30376, .T. ) ;
#27547=AXIS2_PLACEMENT_3D ( 'NONE', #8790, #16034, #3294 ) ;
#27565=CARTESIAN_POINT ( 'NONE',  ( -23.74292845506526461, -13.87604159535428927, 223.8999999999999773 ) ) ;
#27570=EDGE_CURVE ( 'NONE', #1526, #20656, #6241, .T. ) ;
#27574=ORIENTED_EDGE ( 'NONE', *, *, #23939, .T. ) ;
#27582=EDGE_CURVE ( 'NONE', #18237, #20880, #3889, .T. ) ;
#27583=ORIENTED_EDGE ( 'NONE', *, *, #15967, .T. ) ;
#27584=VERTEX_POINT ( 'NONE', #20892 ) ;
#27593=TOROIDAL_SURFACE ( 'NONE', #5980, 29.80000000000000071, 3.000000000000000000 ) ;
#27595=DIRECTION ( 'NONE',  ( 0.000000000000000000, 0.000000000000000000, 1.000000000000000000 ) ) ;
#27596=CARTESIAN_POINT ( 'NONE',  ( -23.73450314257943816, -12.44732035342869203, 5.218051572315431486 ) ) ;
#27597=CARTESIAN_POINT ( 'NONE',  ( 0.000000000000000000, 0.000000000000000000, 115.0000000000000000 ) ) ;
#27599=AXIS2_PLACEMENT_3D ( 'NONE', #15172, #27595, #3361 ) ;
#27605=CARTESIAN_POINT ( 'NONE',  ( -22.63992238021891978, -14.34133587286723710, 4.902940995466560814 ) ) ;
#27614=DIRECTION ( 'NONE',  ( 0.000000000000000000, 0.000000000000000000, 1.000000000000000000 ) ) ;
#27616=CARTESIAN_POINT ( 'NONE',  ( -24.28117756982639364, -12.91036561269763716, 225.5561643545236734 ) ) ;
#27620=DIRECTION ( 'NONE',  ( 1.000000000000000000, 0.000000000000000000, 0.000000000000000000 ) ) ;
#27622=ORIENTED_EDGE ( 'NONE', *, *, #2660, .T. ) ;
#27626=ORIENTED_EDGE ( 'NONE', *, *, #16774, .T. ) ;
#27631=DIRECTION ( 'NONE',  ( 0.000000000000000000, 0.000000000000000000, -1.000000000000000000 ) ) ;
#27637=DIRECTION ( 'NONE',  ( 1.000000000000000000, -1.224606353819999829E-16, 0.000000000000000000 ) ) ;
#27642=LINE ( 'NONE', #8917, #28732 ) ;
#27651=FACE_OUTER_BOUND ( 'NONE', #28599, .T. ) ;
#27653=VERTEX_POINT ( 'NONE', #21044 ) ;
#27663=VERTEX_POINT ( 'NONE', #30948 ) ;
#27667=CIRCLE ( 'NONE', #9600, 26.80000000000000071 ) ;
#27674=EDGE_CURVE ( 'NONE', #17360, #10417, #5342, .T. ) ;
#27683=CARTESIAN_POINT ( 'NONE',  ( 8.903108651239925564, -22.82508830966962421, 90.00000000000000000 ) ) ;
#27686=EDGE_CURVE ( 'NONE', #6309, #1290, #2005, .T. ) ;
#27690=ORIENTED_EDGE ( 'NONE', *, *, #12377, .T. ) ;
#27693=CARTESIAN_POINT ( 'NONE',  ( 0.4946794151854280730, -26.79522481891638108, 4.006804116327493226 ) ) ;
#27695=CARTESIAN_POINT ( 'NONE',  ( 27.23548387180000319, -3.335274659869999873E-15, 91.66046017409999536 ) ) ;
#27696=EDGE_LOOP ( 'NONE', ( #9157, #2995, #13036, #22373, #14887 ) ) ;
#27698=EDGE_CURVE ( 'NONE', #25870, #24116, #20294, .T. ) ;
#27701=ORIENTED_EDGE ( 'NONE', *, *, #27753, .T. ) ;
#27714=CARTESIAN_POINT ( 'NONE',  ( -7.379546049855178147, -26.49401563815923666, 208.0614364002278478 ) ) ;
#27718=CARTESIAN_POINT ( 'NONE',  ( -27.76135143710000008, 3.399672736049999681E-15, 137.6614141009999912 ) ) ;
#27727=ORIENTED_EDGE ( 'NONE', *, *, #15174, .F. ) ;
#27739=ORIENTED_EDGE ( 'NONE', *, *, #3987, .F. ) ;
#27745=CARTESIAN_POINT ( 'NONE',  ( 2.107992564109752998, -27.41908764619381245, 210.0000000000000284 ) ) ;
#27747=FACE_OUTER_BOUND ( 'NONE', #30340, .T. ) ;
#27748=CARTESIAN_POINT ( 'NONE',  ( -0.1474953975175301857, -26.80000000000002203, 223.9000000000000057 ) ) ;
#27749=EDGE_CURVE ( 'NONE', #28706, #11915, #2343, .T. ) ;
#27753=EDGE_CURVE ( 'NONE', #5262, #30396, #15789, .T. ) ;
#27755=CARTESIAN_POINT ( 'NONE',  ( 0.000000000000000000, 0.000000000000000000, 90.00000000000000000 ) ) ;
#27759=CIRCLE ( 'NONE', #3140, 27.92857142860000152 ) ;
#27760=ORIENTED_EDGE ( 'NONE', *, *, #1163, .T. ) ;
#27768=LINE ( 'NONE', #6055, #208 ) ;
#27769=EDGE_LOOP ( 'NONE', ( #29521, #13465, #12925, #22982 ) ) ;
#27781=ORIENTED_EDGE ( 'NONE', *, *, #29279, .T. ) ;
#27794=EDGE_CURVE ( 'NONE', #17040, #4771, #15295, .T. ) ;
#27798=CIRCLE ( 'NONE', #18239, 3.200000000000002398 ) ;
#27804=TOROIDAL_SURFACE ( 'NONE', #7691, 24.50000000000000000, 4.000000000000000000 ) ;
#27814=ORIENTED_EDGE ( 'NONE', *, *, #27913, .F. ) ;
#27822=CIRCLE ( 'NONE', #26817, 2.999999999999999556 ) ;
#27823=VERTEX_POINT ( 'NONE', #12665 ) ;
#27828=CARTESIAN_POINT ( 'NONE',  ( 0.000000000000000000, 0.000000000000000000, 90.00000000000000000 ) ) ;
#27829=PLANE ( 'NONE',  #12076 ) ;
#27836=AXIS2_PLACEMENT_3D ( 'NONE', #11901, #14116, #30793 ) ;
#27859=CARTESIAN_POINT ( 'NONE',  ( -2.107992564109736566, -27.41908764619380889, 20.00000000000000355 ) ) ;
#27869=ORIENTED_EDGE ( 'NONE', *, *, #29999, .F. ) ;
#27871=CIRCLE ( 'NONE', #5256, 4.000000000000001776 ) ;
#27872=CARTESIAN_POINT ( 'NONE',  ( 0.000000000000000000, 0.000000000000000000, 115.0000000000000000 ) ) ;
#27873=CARTESIAN_POINT ( 'NONE',  ( -26.84464185210000053, 3.287411897809999814E-15, 137.4375040469999760 ) ) ;
#27878=EDGE_CURVE ( 'NONE', #8194, #24363, #12868, .T. ) ;
#27881=CARTESIAN_POINT ( 'NONE',  ( -6.984668861240823645, -26.60192251835760757, 208.3914686747987162 ) ) ;
#27882=AXIS2_PLACEMENT_3D ( 'NONE', #21805, #264, #10002 ) ;
#27884=CARTESIAN_POINT ( 'NONE',  ( -27.54391550559999757, 3.373045393730000103E-15, 137.0437466829999948 ) ) ;
#27888=CARTESIAN_POINT ( 'NONE',  ( 24.14619884819310158, -13.16136950074017875, 224.1195089971002972 ) ) ;
#27891=ORIENTED_EDGE ( 'NONE', *, *, #5949, .F. ) ;
#27893=CARTESIAN_POINT ( 'NONE',  ( -11.45957740435848926, -24.29669185712474899, 36.78285841129289224 ) ) ;
#27901=ORIENTED_EDGE ( 'NONE', *, *, #29615, .F. ) ;
#27902=ORIENTED_EDGE ( 'NONE', *, *, #19217, .T. ) ;
#27905=B_SPLINE_CURVE_WITH_KNOTS ( 'NONE', 5,
 ( #29003, #2426, #14855, #28841, #21623, #26797 ),
 .UNSPECIFIED., .F., .F.,
 ( 6, 6 ),
 ( 0.000000000000000000, 2.300779637660000265 ),
 .UNSPECIFIED. ) ;
#27909=VECTOR ( 'NONE', #30086, 1000.000000000000000 ) ;
#27913=EDGE_CURVE ( 'NONE', #16428, #24430, #25338, .T. ) ;
#27917=EDGE_CURVE ( 'NONE', #30789, #17667, #6048, .T. ) ;
#27919=VERTEX_POINT ( 'NONE', #22898 ) ;
#27922=CARTESIAN_POINT ( 'NONE',  ( -27.15000000039999861, 3.324806250669999651E-15, 230.0000000000000000 ) ) ;
#27931=CARTESIAN_POINT ( 'NONE',  ( -23.67167941903505479, -13.99714051993850461, 3.928090679417475695 ) ) ;
#27934=DIRECTION ( 'NONE',  ( -0.8660254037843289066, -0.5000000000001899592, 0.000000000000000000 ) ) ;
#27939=ADVANCED_FACE ( 'NONE', ( #20374 ), #1502, .F. ) ;
#27948=CARTESIAN_POINT ( 'NONE',  ( -1.100000000000000089, -27.47799119230000287, 5.000000000000000000 ) ) ;
#27951=ORIENTED_EDGE ( 'NONE', *, *, #15559, .F. ) ;
#27953=CARTESIAN_POINT ( 'NONE',  ( -26.80000000069999899, 3.281945028329999726E-15, 165.0000000000000000 ) ) ;
#27969=CARTESIAN_POINT ( 'NONE',  ( -23.76736455408141069, -13.83371703036772615, 6.100000000001124079 ) ) ;
#27973=CARTESIAN_POINT ( 'NONE',  ( -0.6425564543738772061, -27.49266737062499999, 224.0869147246957027 ) ) ;
#27975=ADVANCED_FACE ( 'NONE', ( #13759 ), #21841, .T. ) ;
#27983=VERTEX_POINT ( 'NONE', #4325 ) ;
#27985=DIRECTION ( 'NONE',  ( -0.8090169943751909232, 0.5877852522921378498, 0.000000000000000000 ) ) ;
#27986=AXIS2_PLACEMENT_3D ( 'NONE', #29026, #17068, #12498 ) ;
#27987=DIRECTION ( 'NONE',  ( 0.3633921898465291567, 0.9316362575375349842, 5.551115123125783333E-14 ) ) ;
#28002=B_SPLINE_CURVE_WITH_KNOTS ( 'NONE', 3,
 ( #3491, #15609, #10436, #13242, #20028, #29467, #7903, #29932, #27565, #22698 ),
 .UNSPECIFIED., .F., .F.,
 ( 4, 2, 2, 2, 4 ),
 ( 0.000000000000000000, 0.2500000000000000000, 0.5000000000000000000, 0.7500000000000000000, 1.000000000000000000 ),
 .UNSPECIFIED. ) ;
#28009=AXIS2_PLACEMENT_3D ( 'NONE', #25127, #22462, #10194 ) ;
#28013=ORIENTED_EDGE ( 'NONE', *, *, #25408, .F. ) ;
#28016=ORIENTED_EDGE ( 'NONE', *, *, #1596, .F. ) ;
#28022=DIRECTION ( 'NONE',  ( 0.000000000000000000, 0.000000000000000000, 1.000000000000000000 ) ) ;
#28025=CARTESIAN_POINT ( 'NONE',  ( 23.72659782635170700, -12.46160334561661109, 5.288095983042272685 ) ) ;
#28032=CARTESIAN_POINT ( 'NONE',  ( -9.594426947539474781, -25.77213547066687127, 204.5919004740421485 ) ) ;
#28036=CARTESIAN_POINT ( 'NONE',  ( 0.000000000000000000, 0.000000000000000000, 140.0000000000000000 ) ) ;
#28045=ORIENTED_EDGE ( 'NONE', *, *, #7194, .T. ) ;
#28048=CARTESIAN_POINT ( 'NONE',  ( -26.80000000000000071, 1.065814103639999922E-14, 86.78285841159998881 ) ) ;
#28052=CARTESIAN_POINT ( 'NONE',  ( 18.95046173579999760, -18.95046173579999760, 186.7828584120000244 ) ) ;
#28062=DIRECTION ( 'NONE',  ( 0.3633921898465291567, 0.9316362575375348731, -0.000000000000000000 ) ) ;
#28067=CARTESIAN_POINT ( 'NONE',  ( -23.31845629847328993, -13.20933888637554254, 6.087620939417903720 ) ) ;
#28072=CARTESIAN_POINT ( 'NONE',  ( 26.80000000069999899, -3.281945028320000125E-15, 136.7828584130000138 ) ) ;
#28078=EDGE_CURVE ( 'NONE', #27427, #25385, #30896, .T. ) ;
#28080=CARTESIAN_POINT ( 'NONE',  ( 22.75778669649943353, -14.15360906249806128, 4.333923913290392171 ) ) ;
#28096=B_SPLINE_CURVE_WITH_KNOTS ( 'NONE', 3,
 ( #3074, #12672, #5439, #7946, #276, #19768, #12369, #26999, #29047, #7796, #22279, #26843 ),
 .UNSPECIFIED., .F., .F.,
 ( 4, 2, 2, 2, 2, 4 ),
 ( 0.000000000000000000, 0.2500000000000012768, 0.3750000000000011657, 0.5000000000000011102, 0.7500000000000005551, 1.000000000000000000 ),
 .UNSPECIFIED. ) ;
#28100=CARTESIAN_POINT ( 'NONE',  ( -24.49999999589999788, 3.000285566369999841E-15, 190.0000000000000000 ) ) ;
#28105=ORIENTED_EDGE ( 'NONE', *, *, #17146, .T. ) ;
#28106=LINE ( 'NONE', #21033, #10026 ) ;
#28108=LINE ( 'NONE', #27953, #23106 ) ;
#28109=DIRECTION ( 'NONE',  ( -1.224606353819999829E-16, -1.000000000000000000, 0.000000000000000000 ) ) ;
#28131=DIRECTION ( 'NONE',  ( 0.000000000000000000, 0.000000000000000000, -1.000000000000000000 ) ) ;
#28137=PRODUCT_CONTEXT ( 'NONE', #18620, 'mechanical' ) ;
#28143=CARTESIAN_POINT ( 'NONE',  ( 24.49999999470000134, -3.000285566199999922E-15, 90.00000000069999828 ) ) ;
#28162=CARTESIAN_POINT ( 'NONE',  ( -23.35305511486607344, -13.14889042309849465, 3.928509483819665249 ) ) ;
#28164=B_SPLINE_CURVE_WITH_KNOTS ( 'NONE', 3,
 ( #20843, #30447, #13914, #16423, #1808, #11860, #4160, #2112, #11398, #13753 ),
 .UNSPECIFIED., .F., .F.,
 ( 4, 2, 2, 2, 4 ),
 ( 0.000000000000000000, 0.2500000000000000000, 0.5000000000000000000, 0.7500000000000000000, 1.000000000000000000 ),
 .UNSPECIFIED. ) ;
#28165=CARTESIAN_POINT ( 'NONE',  ( 27.50000000000000000, -3.367667472999999580E-15, 186.7190980919999959 ) ) ;
#28170=ORIENTED_EDGE ( 'NONE', *, *, #1741, .F. ) ;
#28183=CARTESIAN_POINT ( 'NONE',  ( -25.43319852990947183, -8.630493912089182373, 0.000000000000000000 ) ) ;
#28188=CARTESIAN_POINT ( 'NONE',  ( -2.107992564109736122, -27.41908764619381245, 210.0000000000000284 ) ) ;
#28190=CARTESIAN_POINT ( 'NONE',  ( 23.20948082139999968, -13.40000000000000036, 226.0999999999999943 ) ) ;
#28195=FACE_OUTER_BOUND ( 'NONE', #12107, .T. ) ;
#28205=ORIENTED_EDGE ( 'NONE', *, *, #19659, .T. ) ;
#28206=DIRECTION ( 'NONE',  ( 0.000000000000000000, 0.000000000000000000, -1.000000000000000000 ) ) ;
#28207=CARTESIAN_POINT ( 'NONE',  ( 25.43121960300669215, -8.635379644106567554, 186.7828584119999960 ) ) ;
#28212=VERTEX_POINT ( 'NONE', #22552 ) ;
#28218=AXIS2_PLACEMENT_3D ( 'NONE', #2506, #19648, #14318 ) ;
#28228=CARTESIAN_POINT ( 'NONE',  ( -11.08346179031915568, -28.41490585489481902, 136.3944487250000179 ) ) ;
#28233=CARTESIAN_POINT ( 'NONE',  ( -11.08346179031915568, -28.41490585489481902, 186.3944487249999895 ) ) ;
#28238=DIRECTION ( 'NONE',  ( 0.000000000000000000, 0.000000000000000000, -1.000000000000000000 ) ) ;
#28264=ORIENTED_EDGE ( 'NONE', *, *, #16214, .T. ) ;
#28265=CARTESIAN_POINT ( 'NONE',  ( -26.93395386830000149, 3.298349104069999855E-15, 192.2432411359999946 ) ) ;
#28267=CARTESIAN_POINT ( 'NONE',  ( 1.099927927706055852, -26.77741881808358215, 225.1458785545408716 ) ) ;
#28269=EDGE_CURVE ( 'NONE', #18020, #23553, #20322, .T. ) ;
#28280=CIRCLE ( 'NONE', #14721, 27.50000000000000000 ) ;
#28292=EDGE_CURVE ( 'NONE', #8812, #27653, #16305, .T. ) ;
#28296=CARTESIAN_POINT ( 'NONE',  ( 0.000000000000000000, 0.000000000000000000, 40.00000000000000000 ) ) ;
#28298=DIRECTION ( 'NONE',  ( 1.000000000000000000, 0.000000000000000000, 0.000000000000000000 ) ) ;
#28334=CARTESIAN_POINT ( 'NONE',  ( 10.35667741062603397, -26.55163333981976592, 40.00000000000000000 ) ) ;
#28338=CIRCLE ( 'NONE', #17281, 3.000000000000001332 ) ;
#28346=CARTESIAN_POINT ( 'NONE',  ( -8.090238276950914909, -26.28358643434116004, 207.3140698626388314 ) ) ;
#28347=CIRCLE ( 'NONE', #8222, 3.200000004570001888 ) ;
#28357=MECHANICAL_DESIGN_GEOMETRIC_PRESENTATION_REPRESENTATION('',(#15305),#19331);
#28362=DIRECTION ( 'NONE',  ( 0.000000000000000000, 0.000000000000000000, -1.000000000000000000 ) ) ;
#28365=CIRCLE ( 'NONE', #237, 4.000000000000000888 ) ;
#28368=ORIENTED_EDGE ( 'NONE', *, *, #3291, .T. ) ;
#28370=TOROIDAL_SURFACE ( 'NONE', #6263, 30.50000000000000000, 3.000000000000000000 ) ;
#28383=CIRCLE ( 'NONE', #27882, 27.50000000000000000 ) ;
#28386=VERTEX_POINT ( 'NONE', #23957 ) ;
#28389=CARTESIAN_POINT ( 'NONE',  ( 26.80000000000000071, 7.105427357599999217E-15, 0.000000000000000000 ) ) ;
#28392=ORIENTED_EDGE ( 'NONE', *, *, #15174, .T. ) ;
#28398=CARTESIAN_POINT ( 'NONE',  ( 22.86188831120908560, -13.98516151523984341, 4.123351189131411410 ) ) ;
#28402=CARTESIAN_POINT ( 'NONE',  ( -2.947640775130000104E-14, -27.50000000000000000, 223.8999999999999773 ) ) ;
#28409=DIRECTION ( 'NONE',  ( -1.224606353819999829E-16, -1.000000000000000000, 0.000000000000000000 ) ) ;
#28411=ORIENTED_EDGE ( 'NONE', *, *, #23886, .T. ) ;
#28419=LINE ( 'NONE', #6700, #22044 ) ;
#28422=ORIENTED_EDGE ( 'NONE', *, *, #2934, .T. ) ;
#28424=EDGE_LOOP ( 'NONE', ( #2941, #22071, #12423, #26772 ) ) ;
#28451=DIRECTION ( 'NONE',  ( 0.000000000000000000, 0.000000000000000000, 1.000000000000000000 ) ) ;
#28455=CARTESIAN_POINT ( 'NONE',  ( 7.105427357599999217E-15, 3.552713678799999608E-15, 193.6055512750000105 ) ) ;
#28467=CARTESIAN_POINT ( 'NONE',  ( 0.000000000000000000, 0.000000000000000000, 140.0000000000000000 ) ) ;
#28473=CARTESIAN_POINT ( 'NONE',  ( 0.000000000000000000, 0.000000000000000000, 140.0000000000000000 ) ) ;
#28478=VERTEX_POINT ( 'NONE', #3300 ) ;
#28482=ORIENTED_EDGE ( 'NONE', *, *, #28269, .T. ) ;
#28485=ORIENTED_EDGE ( 'NONE', *, *, #11756, .T. ) ;
#28501=EDGE_CURVE ( 'NONE', #3582, #9397, #26863, .T. ) ;
#28502=CARTESIAN_POINT ( 'NONE',  ( -23.28210887531993123, -13.27420452059575062, 223.8999999999999773 ) ) ;
#28504=DIRECTION ( 'NONE',  ( 0.000000000000000000, 0.000000000000000000, 1.000000000000000000 ) ) ;
#28507=CIRCLE ( 'NONE', #18961, 2.999999999999999112 ) ;
#28520=ORIENTED_EDGE ( 'NONE', *, *, #5979, .F. ) ;
#28521=ORIENTED_EDGE ( 'NONE', *, *, #24628, .T. ) ;
#28522=ORIENTED_EDGE ( 'NONE', *, *, #8074, .T. ) ;
#28530=TOROIDAL_SURFACE ( 'NONE', #24997, 30.50000000000000000, 3.000000000000000000 ) ;
#28532=AXIS2_PLACEMENT_3D ( 'NONE', #8262, #5756, #15663 ) ;
#28534=TOROIDAL_SURFACE ( 'NONE', #1403, 30.50000000000000000, 3.000000000000000000 ) ;
#28544=CARTESIAN_POINT ( 'NONE',  ( -9.738910687886976447, -24.96785170200593384, 43.21714158840000408 ) ) ;
#28547=CIRCLE ( 'NONE', #16971, 27.23548387100000312 ) ;
#28550=B_SPLINE_CURVE_WITH_KNOTS ( 'NONE', 5,
 ( #18664, #24168, #28265, #2463, #12202, #23716 ),
 .UNSPECIFIED., .F., .F.,
 ( 6, 6 ),
 ( -2.319815200069999861, 0.000000000000000000 ),
 .UNSPECIFIED. ) ;
#28558=CYLINDRICAL_SURFACE ( 'NONE', #6065, 26.80000000000002203 ) ;
#28567=ORIENTED_EDGE ( 'NONE', *, *, #4671, .T. ) ;
#28568=CARTESIAN_POINT ( 'NONE',  ( -8.903108651239966420, -22.82508830966961000, 140.0000000000000000 ) ) ;
#28570=VERTEX_POINT ( 'NONE', #13525 ) ;
#28575=CARTESIAN_POINT ( 'NONE',  ( 0.000000000000000000, 0.000000000000000000, 210.0000000000000284 ) ) ;
#28578=CARTESIAN_POINT ( 'NONE',  ( 27.63177371540000138, -3.383804565909999813E-15, 42.63947604839999883 ) ) ;
#28585=CARTESIAN_POINT ( 'NONE',  ( 0.5612683548718201409, -26.79446734662158747, 225.9574525908840883 ) ) ;
#28591=EDGE_CURVE ( 'NONE', #6179, #21098, #6061, .T. ) ;
#28598=DIRECTION ( 'NONE',  ( 1.000000000000000000, 0.000000000000000000, 0.000000000000000000 ) ) ;
#28599=EDGE_LOOP ( 'NONE', ( #17987, #7389, #12573, #14149 ) ) ;
#28601=ORIENTED_EDGE ( 'NONE', *, *, #27686, .F. ) ;
#28606=ORIENTED_EDGE ( 'NONE', *, *, #12119, .T. ) ;
#28625=DIRECTION ( 'NONE',  ( 0.000000000000000000, 0.000000000000000000, 1.000000000000000000 ) ) ;
#28628=CARTESIAN_POINT ( 'NONE',  ( -23.54244930407671532, -12.80639529791832842, 4.123351189496611724 ) ) ;
#28638=DIRECTION ( 'NONE',  ( 0.000000000000000000, 0.000000000000000000, 1.000000000000000000 ) ) ;
#28639=ORIENTED_EDGE ( 'NONE', *, *, #24049, .T. ) ;
#28648=DIRECTION ( 'NONE',  ( 1.000000000000000000, -1.224606353819998843E-16, 0.000000000000000000 ) ) ;
#28661=DIRECTION ( 'NONE',  ( 0.000000000000000000, 0.000000000000000000, -1.000000000000000000 ) ) ;
#28664=CARTESIAN_POINT ( 'NONE',  ( -24.50000001620000134, 3.000285568850000245E-15, 190.0000000039999861 ) ) ;
#28667=ORIENTED_EDGE ( 'NONE', *, *, #17728, .F. ) ;
#28668=AXIS2_PLACEMENT_3D ( 'NONE', #18538, #9242, #25195 ) ;
#28670=DIRECTION ( 'NONE',  ( 1.000000000000000000, 0.000000000000000000, 0.000000000000000000 ) ) ;
#28675=ORIENTED_EDGE ( 'NONE', *, *, #3704, .T. ) ;
#28678=CIRCLE ( 'NONE', #30176, 26.80000000000000071 ) ;
#28682=DIRECTION ( 'NONE',  ( 0.000000000000000000, 0.000000000000000000, -1.000000000000000000 ) ) ;
#28687=DIRECTION ( 'NONE',  ( 1.881554647690000340E-09, 1.000000000000000000, 0.000000000000000000 ) ) ;
#28690=ORIENTED_EDGE ( 'NONE', *, *, #11149, .T. ) ;
#28697=VERTEX_POINT ( 'NONE', #13611 ) ;
#28698=CARTESIAN_POINT ( 'NONE',  ( -27.92857142820000149, 5.329070518200000398E-15, 137.9396849850000137 ) ) ;
#28700=CARTESIAN_POINT ( 'NONE',  ( 26.80000000069999899, -3.281945028320000125E-15, 92.88981852279999885 ) ) ;
#28706=VERTEX_POINT ( 'NONE', #15971 ) ;
#28726=CARTESIAN_POINT ( 'NONE',  ( 18.95046173579999760, -18.95046173579999760, 143.2171415880000040 ) ) ;
#28732=VECTOR ( 'NONE', #13164, 1000.000000000000000 ) ;
#28736=CARTESIAN_POINT ( 'NONE',  ( 0.000000000000000000, 0.000000000000000000, 115.0000000000000000 ) ) ;
#28741=CARTESIAN_POINT ( 'NONE',  ( 26.80000000069999899, -3.281945028320000125E-15, 86.78285841090000474 ) ) ;
#28783=VERTEX_POINT ( 'NONE', #9041 ) ;
#28785=ORIENTED_EDGE ( 'NONE', *, *, #26568, .F. ) ;
#28789=DIRECTION ( 'NONE',  ( 1.000000000000000000, 0.000000000000000000, 0.000000000000000000 ) ) ;
#28809=CARTESIAN_POINT ( 'NONE',  ( -8.903108651239966420, -22.82508830966961000, 40.00000000000000000 ) ) ;
#28813=DIRECTION ( 'NONE',  ( 0.000000000000000000, 0.000000000000000000, -1.000000000000000000 ) ) ;
#28814=VERTEX_POINT ( 'NONE', #18637 ) ;
#28817=ORIENTED_EDGE ( 'NONE', *, *, #846, .T. ) ;
#28825=EDGE_CURVE ( 'NONE', #10713, #12574, #19772, .T. ) ;
#28826=AXIS2_PLACEMENT_3D ( 'NONE', #12070, #2172, #31115 ) ;
#28828=AXIS2_PLACEMENT_3D ( 'NONE', #281, #9861, #26692 ) ;
#28830=DIRECTION ( 'NONE',  ( 0.000000000000000000, 0.000000000000000000, 1.000000000000000000 ) ) ;
#28841=CARTESIAN_POINT ( 'NONE',  ( -27.54391552369999729, 3.373045395949999841E-15, 142.9562530130000084 ) ) ;
#28842=ORIENTED_EDGE ( 'NONE', *, *, #30649, .F. ) ;
#28845=CARTESIAN_POINT ( 'NONE',  ( 22.87891075595186763, -13.95728375069770877, 5.909812224949991588 ) ) ;
#28846=DIRECTION ( 'NONE',  ( 0.3633921898465276024, -0.9316362575375355393, 0.000000000000000000 ) ) ;
#28857=ADVANCED_FACE ( 'NONE', ( #21632 ), #26792, .T. ) ;
#28858=CIRCLE ( 'NONE', #12778, 27.92857142840000151 ) ;
#28859=VECTOR ( 'NONE', #11288, 1000.000000000000000 ) ;
#28868=( GEOMETRIC_REPRESENTATION_CONTEXT ( 3 ) GLOBAL_UNCERTAINTY_ASSIGNED_CONTEXT ( ( #5577 ) ) GLOBAL_UNIT_ASSIGNED_CONTEXT ( ( #22570, #17823, #22253 ) ) REPRESENTATION_CONTEXT ( 'NONE', 'WORKASPACE' ) );
#28878=CARTESIAN_POINT ( 'NONE',  ( -26.80000000000000071, 6.217248937899999413E-15, 136.7828584120000244 ) ) ;
#28882=AXIS2_PLACEMENT_3D ( 'NONE', #22385, #10884, #24897 ) ;
#28886=EDGE_LOOP ( 'NONE', ( #16168, #18838, #29247, #26369, #28411, #16939 ) ) ;
#28888=CARTESIAN_POINT ( 'NONE',  ( 23.62009186283282958, -12.66256056296848342, 224.2880739211889249 ) ) ;
#28889=CARTESIAN_POINT ( 'NONE',  ( 10.35667741062603397, -26.55163333981976592, 90.00000000000000000 ) ) ;
#28891=CARTESIAN_POINT ( 'NONE',  ( 0.000000000000000000, 0.000000000000000000, 90.00000000000000000 ) ) ;
#28895=CARTESIAN_POINT ( 'NONE',  ( -0.9876156946363959799, -26.78228253927133196, 225.4913731638064576 ) ) ;
#28899=ADVANCED_FACE ( 'NONE', ( #12793 ), #26499, .T. ) ;
#28914=DIRECTION ( 'NONE',  ( -0.3633921898465292122, -0.9316362575375349842, 0.000000000000000000 ) ) ;
#28925=ORIENTED_EDGE ( 'NONE', *, *, #18281, .T. ) ;
#28933=ADVANCED_FACE ( 'NONE', ( #14862 ), #24914, .F. ) ;
#28937=CARTESIAN_POINT ( 'NONE',  ( 1.018916989216064772, -26.78112380533112358, 224.5794179396494883 ) ) ;
#28943=B_SPLINE_CURVE_WITH_KNOTS ( 'NONE', 3,
 ( #13238, #10584, #17801, #3032, #12625, #8053, #22854, #15148, #3184, #694, #5850, #12787 ),
 .UNSPECIFIED., .F., .F.,
 ( 4, 2, 2, 2, 2, 4 ),
 ( 0.000000000000000000, 0.2499999999999988343, 0.3749999999999989453, 0.4999999999999991118, 0.7499999999999995559, 1.000000000000000000 ),
 .UNSPECIFIED. ) ;
#28953=VERTEX_POINT ( 'NONE', #29629 ) ;
#28954=CARTESIAN_POINT ( 'NONE',  ( -24.49999999470000134, 3.000285566209999917E-15, 90.00000000069999828 ) ) ;
#28961=CARTESIAN_POINT ( 'NONE',  ( -27.50000000000000000, 3.367667473009999970E-15, 43.28090191839999790 ) ) ;
#28972=B_SPLINE_CURVE_WITH_KNOTS ( 'NONE', 5,
 ( #10611, #22425, #17379, #27288, #25088, #7626 ),
 .UNSPECIFIED., .F., .F.,
 ( 6, 6 ),
 ( 0.000000000000000000, 2.300779637260000232 ),
 .UNSPECIFIED. ) ;
#28977=ORIENTED_EDGE ( 'NONE', *, *, #6124, .F. ) ;
#28991=ORIENTED_EDGE ( 'NONE', *, *, #9065, .F. ) ;
#29003=CARTESIAN_POINT ( 'NONE',  ( -27.92857142909999979, 3.420150602519999655E-15, 142.0603150149999863 ) ) ;
#29018=AXIS2_PLACEMENT_3D ( 'NONE', #11506, #13551, #13870 ) ;
#29026=CARTESIAN_POINT ( 'NONE',  ( 8.903108651239925564, -22.82508830966962421, 90.00000000000000000 ) ) ;
#29031=EDGE_CURVE ( 'NONE', #13864, #7590, #22794, .T. ) ;
#29033=TOROIDAL_SURFACE ( 'NONE', #17486, 24.50000000000000000, 3.200000000000000178 ) ;
#29047=CARTESIAN_POINT ( 'NONE',  ( 0.5621952752015302313, -27.49459032396439540, 4.043049797261333289 ) ) ;
#29052=CARTESIAN_POINT ( 'NONE',  ( -24.34663841809999951, -12.78636765230000094, 5.000000000000000000 ) ) ;
#29067=ORIENTED_EDGE ( 'NONE', *, *, #9079, .F. ) ;
#29070=CARTESIAN_POINT ( 'NONE',  ( 9.993285220779439371, -25.61999708228226069, 86.39444872449999480 ) ) ;
#29081=CARTESIAN_POINT ( 'NONE',  ( 0.9950318228358414618, -27.48257863589062922, 225.4905541412982757 ) ) ;
#29084=DIRECTION ( 'NONE',  ( 0.9316362575375356503, 0.3633921898465274913, 0.000000000000000000 ) ) ;
#29099=AXIS2_PLACEMENT_3D ( 'NONE', #9653, #14544, #26343 ) ;
#29118=CARTESIAN_POINT ( 'NONE',  ( 27.92857142909999979, -3.420150602509999660E-15, 87.93968498519998889 ) ) ;
#29121=CARTESIAN_POINT ( 'NONE',  ( 2.107992564109750333, -27.41908764619381245, 20.00000000000000355 ) ) ;
#29126=VERTEX_POINT ( 'NONE', #660 ) ;
#29127=DIRECTION ( 'NONE',  ( -1.000000000000000000, 5.665498452320000818E-16, 0.000000000000000000 ) ) ;
#29132=FACE_OUTER_BOUND ( 'NONE', #18965, .T. ) ;
#29139=FACE_OUTER_BOUND ( 'NONE', #26008, .T. ) ;
#29148=EDGE_LOOP ( 'NONE', ( #11741, #12313, #21875, #1048 ) ) ;
#29156=CARTESIAN_POINT ( 'NONE',  ( 22.68367506382111287, -14.27296989803571314, 5.420582065402280492 ) ) ;
#29176=CARTESIAN_POINT ( 'NONE',  ( -24.13062658843018227, -13.18986347163402506, 4.086914725630220069 ) ) ;
#29177=CARTESIAN_POINT ( 'NONE',  ( 0.5569265643388185971, -27.49469370723012673, 224.0404533956380249 ) ) ;
#29198=CARTESIAN_POINT ( 'NONE',  ( -23.95771898009571999, -13.50170546721040310, 6.071909320494010665 ) ) ;
#29203=DIRECTION ( 'NONE',  ( 1.000000000000000000, 0.000000000000000000, 0.000000000000000000 ) ) ;
#29230=CARTESIAN_POINT ( 'NONE',  ( 0.09666810063946208731, -27.50000000000001066, 226.1000000000000227 ) ) ;
#29232=DIRECTION ( 'NONE',  ( 0.000000000000000000, 0.000000000000000000, 1.000000000000000000 ) ) ;
#29247=ORIENTED_EDGE ( 'NONE', *, *, #21269, .F. ) ;
#29256=FACE_OUTER_BOUND ( 'NONE', #21649, .T. ) ;
#29261=CARTESIAN_POINT ( 'NONE',  ( 0.000000000000000000, 0.000000000000000000, 115.0000000000000000 ) ) ;
#29267=DIRECTION ( 'NONE',  ( 0.000000000000000000, 0.000000000000000000, -1.000000000000000000 ) ) ;
#29277=EDGE_CURVE ( 'NONE', #22078, #1493, #10246, .T. ) ;
#29279=EDGE_CURVE ( 'NONE', #4649, #19471, #5669, .T. ) ;
#29284=DIRECTION ( 'NONE',  ( -1.000000000000000000, 5.665498452320000818E-16, 0.000000000000000000 ) ) ;
#29289=ORIENTED_EDGE ( 'NONE', *, *, #6981, .F. ) ;
#29297=DIRECTION ( 'NONE',  ( 0.000000000000000000, 0.000000000000000000, -1.000000000000000000 ) ) ;
#29298=DIRECTION ( 'NONE',  ( 1.000000000000000000, 0.000000000000000000, 0.000000000000000000 ) ) ;
#29301=CARTESIAN_POINT ( 'NONE',  ( 26.84464183080000055, -3.287411895189999871E-15, 42.56249624490000372 ) ) ;
#29303=CARTESIAN_POINT ( 'NONE',  ( -23.25788685383075105, -13.43083806724683882, 193.2171415880000040 ) ) ;
#29310=CARTESIAN_POINT ( 'NONE',  ( 24.50000001620000134, -3.000285568839999855E-15, 140.0000000040000145 ) ) ;
#29316=ADVANCED_FACE ( 'NONE', ( #10869 ), #29817, .T. ) ;
#29322=AXIS2_PLACEMENT_3D ( 'NONE', #6447, #13848, #14006 ) ;
#29333=LINE ( 'NONE', #7777, #18041 ) ;
#29342=DIRECTION ( 'NONE',  ( 1.000000000000000000, -1.224606353819998843E-16, 0.000000000000000000 ) ) ;
#29344=TOROIDAL_SURFACE ( 'NONE', #2233, 24.50000000000000000, 3.200000000000000178 ) ;
#29350=CARTESIAN_POINT ( 'NONE',  ( -4.421808970600616284, -26.43392618132182292, 209.5992702222104640 ) ) ;
#29355=FACE_OUTER_BOUND ( 'NONE', #30547, .T. ) ;
#29356=CARTESIAN_POINT ( 'NONE',  ( -9.484767271962882162, -25.06561782275614547, 25.91365951406786294 ) ) ;
#29365=ORIENTED_EDGE ( 'NONE', *, *, #22789, .F. ) ;
#29370=ORIENTED_EDGE ( 'NONE', *, *, #16284, .T. ) ;
#29374=CARTESIAN_POINT ( 'NONE',  ( -26.79999999999999361, -1.754055898254264445, 143.2171415879999756 ) ) ;
#29399=VERTEX_POINT ( 'NONE', #25965 ) ;
#29401=CIRCLE ( 'NONE', #6298, 26.79999999889999884 ) ;
#29406=VERTEX_POINT ( 'NONE', #1739 ) ;
#29416=CARTESIAN_POINT ( 'NONE',  ( -9.897162125286939727, -25.37356426548038613, 188.3395398250000028 ) ) ;
#29421=ADVANCED_FACE ( 'NONE', ( #18405 ), #13531, .F. ) ;
#29428=CARTESIAN_POINT ( 'NONE',  ( -27.50000000000000000, 3.367667473009999970E-15, 0.000000000000000000 ) ) ;
#29439=ORIENTED_EDGE ( 'NONE', *, *, #1742, .F. ) ;
#29448=EDGE_CURVE ( 'NONE', #18243, #24363, #29680, .T. ) ;
#29449=ORIENTED_EDGE ( 'NONE', *, *, #29708, .F. ) ;
#29462=CYLINDRICAL_SURFACE ( 'NONE', #22390, 1.100000000000000089 ) ;
#29467=CARTESIAN_POINT ( 'NONE',  ( -23.47117976025595354, -14.33053685711701419, 224.1195089972090102 ) ) ;
#29472=ORIENTED_EDGE ( 'NONE', *, *, #30062, .T. ) ;
#29475=B_SPLINE_CURVE_WITH_KNOTS ( 'NONE', 5,
 ( #9418, #19495, #21397, #9732, #19025, #2202 ),
 .UNSPECIFIED., .F., .F.,
 ( 6, 6 ),
 ( -2.300779637610000261, 0.000000000000000000 ),
 .UNSPECIFIED. ) ;
#29494=EDGE_CURVE ( 'NONE', #25858, #1290, #708, .T. ) ;
#29505=CARTESIAN_POINT ( 'NONE',  ( -6.706468900734749106, -25.94814536837671426, 208.3914661911716735 ) ) ;
#29514=CARTESIAN_POINT ( 'NONE',  ( -23.82266443414333423, -12.31939917416737629, 93.21714158843887787 ) ) ;
#29516=ORIENTED_EDGE ( 'NONE', *, *, #17758, .F. ) ;
#29518=DIRECTION ( 'NONE',  ( 0.7071067811865475727, -0.7071067811865475727, 0.000000000000000000 ) ) ;
#29521=ORIENTED_EDGE ( 'NONE', *, *, #3411, .F. ) ;
#29528=CARTESIAN_POINT ( 'NONE',  ( -23.20948082139999968, -13.40000000000000036, 226.0999999999999943 ) ) ;
#29533=B_SPLINE_CURVE_WITH_KNOTS ( 'NONE', 5,
 ( #22820, #5976, #18080, #813, #20298, #12911 ),
 .UNSPECIFIED., .F., .F.,
 ( 6, 6 ),
 ( 0.000000000000000000, 2.300779653469999797 ),
 .UNSPECIFIED. ) ;
#29538=ORIENTED_EDGE ( 'NONE', *, *, #22913, .T. ) ;
#29549=CARTESIAN_POINT ( 'NONE',  ( 9.254368700311683682, -25.15168151593200818, 204.8447925225967481 ) ) ;
#29551=CARTESIAN_POINT ( 'NONE',  ( -26.80000000069999899, 3.281945028329999726E-15, 43.21714158909999526 ) ) ;
#29554=CARTESIAN_POINT ( 'NONE',  ( 23.92402432494557729, -13.56054119037707117, 226.0877068033694002 ) ) ;
#29558=ORIENTED_EDGE ( 'NONE', *, *, #10254, .T. ) ;
#29580=AXIS2_PLACEMENT_3D ( 'NONE', #10895, #22237, #20331 ) ;
#29581=EDGE_CURVE ( 'NONE', #17360, #6881, #9725, .T. ) ;
#29591=ORIENTED_EDGE ( 'NONE', *, *, #11703, .T. ) ;
#29593=FACE_OUTER_BOUND ( 'NONE', #17792, .T. ) ;
#29594=FACE_OUTER_BOUND ( 'NONE', #25824, .T. ) ;
#29608=AXIS2_PLACEMENT_3D ( 'NONE', #11969, #11821, #16533 ) ;
#29615=EDGE_CURVE ( 'NONE', #27542, #13694, #21388, .T. ) ;
#29617=EDGE_CURVE ( 'NONE', #6309, #21418, #9718, .T. ) ;
#29620=CARTESIAN_POINT ( 'NONE',  ( -24.08872333959828893, -11.87645233066224826, 193.2171415879999756 ) ) ;
#29625=( GEOMETRIC_REPRESENTATION_CONTEXT ( 3 ) GLOBAL_UNCERTAINTY_ASSIGNED_CONTEXT ( ( #16304 ) ) GLOBAL_UNIT_ASSIGNED_CONTEXT ( ( #1680, #3880, #20717 ) ) REPRESENTATION_CONTEXT ( 'NONE', 'WORKASPACE' ) );
#29627=CIRCLE ( 'NONE', #22091, 26.80000000000000071 ) ;
#29629=CARTESIAN_POINT ( 'NONE',  ( -27.69999999930000101, 3.392159599999999562E-15, 190.0000000000000000 ) ) ;
#29638=EDGE_CURVE ( 'NONE', #24321, #20581, #30348, .T. ) ;
#29649=CARTESIAN_POINT ( 'NONE',  ( -27.50000000000000000, 3.367667473009999970E-15, 0.000000000000000000 ) ) ;
#29652=LINE ( 'NONE', #22113, #6034 ) ;
#29657=CARTESIAN_POINT ( 'NONE',  ( -3.552713678799999608E-15, 0.000000000000000000, 43.21714158840000408 ) ) ;
#29660=CARTESIAN_POINT ( 'NONE',  ( -22.73383167079628819, -14.19258501544933004, 4.402070809670797225 ) ) ;
#29663=CARTESIAN_POINT ( 'NONE',  ( -23.26185891380717763, -14.66761890373121524, 4.713248588340865020 ) ) ;
#29664=AXIS2_PLACEMENT_3D ( 'NONE', #23277, #1721, #20917 ) ;
#29667=CARTESIAN_POINT ( 'NONE',  ( 27.50000000000000000, -3.367667472999999580E-15, 143.2809019210000088 ) ) ;
#29671=CARTESIAN_POINT ( 'NONE',  ( -5.852082250035282485, -26.15431190117149995, 21.03698545514888707 ) ) ;
#29680=B_SPLINE_CURVE_WITH_KNOTS ( 'NONE', 3,
 ( #11795, #20930, #21401, #16201, #30991, #30533, #9423, #28628, #25498, #28162, #25814, #4253 ),
 .UNSPECIFIED., .F., .F.,
 ( 4, 2, 2, 2, 2, 4 ),
 ( 0.000000000000000000, 0.2499999999999983347, 0.3749999999999973355, 0.4999999999999963363, 0.7499999999999981126, 1.000000000000000000 ),
 .UNSPECIFIED. ) ;
#29682=VERTEX_POINT ( 'NONE', #25141 ) ;
#29683=ORIENTED_EDGE ( 'NONE', *, *, #5213, .F. ) ;
#29700=DIRECTION ( 'NONE',  ( 0.000000000000000000, 0.000000000000000000, 1.000000000000000000 ) ) ;
#29705=CARTESIAN_POINT ( 'NONE',  ( 3.931979172340990036, -26.51120696000497645, 209.7426969702732720 ) ) ;
#29707=CARTESIAN_POINT ( 'NONE',  ( -22.81399828927099094, -14.09994392937124985, 43.21714158846111786 ) ) ;
#29708=EDGE_CURVE ( 'NONE', #3758, #28478, #2596, .T. ) ;
#29723=CARTESIAN_POINT ( 'NONE',  ( 9.897162125400447152, -25.37356426577149549, 88.33953982530000815 ) ) ;
#29725=DIRECTION ( 'NONE',  ( -1.000000000000000000, 1.224606353819999829E-16, 0.000000000000000000 ) ) ;
#29729=LINE ( 'NONE', #1096, #15004 ) ;
#29730=CARTESIAN_POINT ( 'NONE',  ( 9.993285220779513978, -25.61999708228223227, 143.6055512739999926 ) ) ;
#29734=CARTESIAN_POINT ( 'NONE',  ( 0.000000000000000000, 0.000000000000000000, 115.0000000000000000 ) ) ;
#29740=CIRCLE ( 'NONE', #30236, 26.80000000000000071 ) ;
#29744=ORIENTED_EDGE ( 'NONE', *, *, #6705, .F. ) ;
#29747=ORIENTED_EDGE ( 'NONE', *, *, #29825, .T. ) ;
#29751=CARTESIAN_POINT ( 'NONE',  ( -0.8784922619252688580, -26.78562592415266153, 4.333924731881555026 ) ) ;
#29758=ORIENTED_EDGE ( 'NONE', *, *, #3517, .T. ) ;
#29767=CARTESIAN_POINT ( 'NONE',  ( -4.130757957910000097E-10, -1.288485762530000039E-09, 230.0000000000000000 ) ) ;
#29772=LINE ( 'NONE', #3336, #731 ) ;
#29787=ORIENTED_EDGE ( 'NONE', *, *, #22457, .F. ) ;
#29802=CARTESIAN_POINT ( 'NONE',  ( 0.2892544189978767388, -26.79878419700509085, 6.071490516278870153 ) ) ;
#29817=TOROIDAL_SURFACE ( 'NONE', #7206, 24.50000000000000000, 4.000000000000000000 ) ;
#29819=CARTESIAN_POINT ( 'NONE',  ( -24.76914019444433279, -10.23375669952358358, 93.21714158839957065 ) ) ;
#29823=DIRECTION ( 'NONE',  ( -0.7071067811865475727, 0.7071067811865475727, 0.000000000000000000 ) ) ;
#29825=EDGE_CURVE ( 'NONE', #9526, #25596, #19882, .T. ) ;
#29834=CIRCLE ( 'NONE', #20290, 3.200000000000002398 ) ;
#29836=CIRCLE ( 'NONE', #24840, 28.50000000000000000 ) ;
#29839=AXIS2_PLACEMENT_3D ( 'NONE', #5118, #12362, #7633 ) ;
#29846=CARTESIAN_POINT ( 'NONE',  ( 27.50000000000000000, -3.367667472999999580E-15, 136.7190980919999959 ) ) ;
#29853=EDGE_CURVE ( 'NONE', #27919, #2249, #4366, .T. ) ;
#29857=CARTESIAN_POINT ( 'NONE',  ( -25.04491701902129819, -9.543388590360489587, 43.21714158838634745 ) ) ;
#29860=CARTESIAN_POINT ( 'NONE',  ( 9.689804814931740395, -24.98716964724288658, 26.94038990441057280 ) ) ;
#29861=ORIENTED_EDGE ( 'NONE', *, *, #1511, .T. ) ;
#29865=FACE_BOUND ( 'NONE', #1673, .T. ) ;
#29892=DIRECTION ( 'NONE',  ( -0.7071067811865475727, -0.7071067811865475727, 0.000000000000000000 ) ) ;
#29897=CARTESIAN_POINT ( 'NONE',  ( 22.64684861877907451, -14.33122899589083943, 225.2180667916778702 ) ) ;
#29899=DIRECTION ( 'NONE',  ( 0.000000000000000000, 0.000000000000000000, -1.000000000000000000 ) ) ;
#29907=CARTESIAN_POINT ( 'NONE',  ( -22.88229166409188409, -13.95171381497113039, 224.0862411982057267 ) ) ;
#29909=EDGE_LOOP ( 'NONE', ( #5596, #13067, #11957, #17183 ) ) ;
#29910=CARTESIAN_POINT ( 'NONE',  ( -9.993285220779423383, -25.61999708228226069, 27.46711697431777921 ) ) ;
#29911=ORIENTED_EDGE ( 'NONE', *, *, #13862, .F. ) ;
#29914=ORIENTED_EDGE ( 'NONE', *, *, #27794, .T. ) ;
#29932=CARTESIAN_POINT ( 'NONE',  ( -23.67167941898225791, -13.99714052002833320, 223.9280906791120458 ) ) ;
#29933=DIRECTION ( 'NONE',  ( 0.3633921898465292122, 0.9316362575375348731, -6.938893903907226800E-15 ) ) ;
#29935=CARTESIAN_POINT ( 'NONE',  ( 23.81569860410000317, -13.75000000000000000, 223.8999999999999773 ) ) ;
#29941=ORIENTED_EDGE ( 'NONE', *, *, #8095, .F. ) ;
#29953=EDGE_CURVE ( 'NONE', #21389, #21418, #21322, .T. ) ;
#29959=ORIENTED_EDGE ( 'NONE', *, *, #22848, .T. ) ;
#29965=DIRECTION ( 'NONE',  ( 0.9316362575375356503, 0.3633921898465274913, 0.000000000000000000 ) ) ;
#29968=DIRECTION ( 'NONE',  ( 0.000000000000000000, 0.000000000000000000, 1.000000000000000000 ) ) ;
#29977=CARTESIAN_POINT ( 'NONE',  ( -3.552713678799999608E-15, -3.552713678799999608E-15, 91.66046017469999185 ) ) ;
#29982=ORIENTED_EDGE ( 'NONE', *, *, #24595, .T. ) ;
#29983=EDGE_CURVE ( 'NONE', #19781, #25596, #14254, .T. ) ;
#29998=CIRCLE ( 'NONE', #14943, 27.69999999999999929 ) ;
#29999=EDGE_CURVE ( 'NONE', #15620, #25870, #30004, .T. ) ;
#30004=B_SPLINE_CURVE_WITH_KNOTS ( 'NONE', 3,
 ( #21513, #9551, #27458, #30427, #22286, #10631, #3233, #17852, #19926, #20225, #13577, #17693, #12522, #29819, #16092, #27311, #7949, #5594, #29514, #5901, #591, #12676, #10173, #24646, #892, #5750 ),
 .UNSPECIFIED., .F., .F.,
 ( 4, 2, 2, 2, 1, 1, 1, 1, 1, 1, 2, 2, 2, 2, 2, 4 ),
 ( 0.000000000000000000, 0.2499999999999633626, 0.3749999999999450440, 0.4374999999999361067, 0.4687499999999313882, 0.4843749999999291123, 0.4921874999999278910, 0.4960937499999271139, 0.4980468749999268363, 0.4990234374999269473, 0.4995117187499270583, 0.4999999999999272804, 0.6249999999999453770, 0.7499999999999634737, 0.8749999999999817923, 1.000000000000000000 ),
 .UNSPECIFIED. ) ;
#30008=EDGE_CURVE ( 'NONE', #16461, #20682, #2985, .T. ) ;
#30012=CARTESIAN_POINT ( 'NONE',  ( -24.31247271682645206, -11.33627354958356825, 43.21714158842222986 ) ) ;
#30014=CARTESIAN_POINT ( 'NONE',  ( 23.86403265435992083, -13.66628296921426156, 226.0999999999988859 ) ) ;
#30018=EDGE_CURVE ( 'NONE', #18284, #17478, #4498, .T. ) ;
#30038=CARTESIAN_POINT ( 'NONE',  ( 10.14902473071355793, -26.01926976408358527, 42.06031501460000044 ) ) ;
#30040=CIRCLE ( 'NONE', #31067, 3.000000000000001332 ) ;
#30045=DIRECTION ( 'NONE',  ( 1.000000000000000000, 0.000000000000000000, 0.000000000000000000 ) ) ;
#30057=FACE_OUTER_BOUND ( 'NONE', #11440, .T. ) ;
#30059=CARTESIAN_POINT ( 'NONE',  ( 14.39562240800000126, -9.581487064249998298, 5.000000000000000000 ) ) ;
#30062=EDGE_CURVE ( 'NONE', #6137, #25637, #5226, .T. ) ;
#30064=CARTESIAN_POINT ( 'NONE',  ( -1.071233646927975736, -26.77863814329466052, 4.711903514136000837 ) ) ;
#30065=ORIENTED_EDGE ( 'NONE', *, *, #30062, .F. ) ;
#30066=ORIENTED_EDGE ( 'NONE', *, *, #6301, .F. ) ;
#30069=ORIENTED_EDGE ( 'NONE', *, *, #9821, .F. ) ;
#30074=AXIS2_PLACEMENT_3D ( 'NONE', #18801, #28409, #7580 ) ;
#30079=AXIS2_PLACEMENT_3D ( 'NONE', #13194, #13519, #20599 ) ;
#30083=ORIENTED_EDGE ( 'NONE', *, *, #23107, .F. ) ;
#30086=DIRECTION ( 'NONE',  ( -1.000000000000000000, -5.289357741729999318E-17, 0.000000000000000000 ) ) ;
#30092=AXIS2_PLACEMENT_3D ( 'NONE', #29657, #20371, #18154 ) ;
#30096=ORIENTED_EDGE ( 'NONE', *, *, #15572, .F. ) ;
#30104=CARTESIAN_POINT ( 'NONE',  ( 24.08872333959831380, -11.87645233066226069, 186.7828584119999960 ) ) ;
#30105=ORIENTED_EDGE ( 'NONE', *, *, #14186, .F. ) ;
#30107=ORIENTED_EDGE ( 'NONE', *, *, #29853, .F. ) ;
#30110=EDGE_CURVE ( 'NONE', #18767, #25637, #29836, .T. ) ;
#30116=DIRECTION ( 'NONE',  ( 0.000000000000000000, 0.000000000000000000, 1.000000000000000000 ) ) ;
#30117=CARTESIAN_POINT ( 'NONE',  ( -0.9891023348422632866, -26.78175549063930205, 224.5133938523520385 ) ) ;
#30122=AXIS2_PLACEMENT_3D ( 'NONE', #8350, #3482, #13393 ) ;
#30126=ORIENTED_EDGE ( 'NONE', *, *, #886, .F. ) ;
#30128=CARTESIAN_POINT ( 'NONE',  ( -22.74641636049597793, -14.17229404738486132, 4.366512952753266674 ) ) ;
#30143=DIRECTION ( 'NONE',  ( 0.000000000000000000, 0.000000000000000000, 1.000000000000000000 ) ) ;
#30152=DIRECTION ( 'NONE',  ( 0.000000000000000000, 0.000000000000000000, -1.000000000000000000 ) ) ;
#30176=AXIS2_PLACEMENT_3D ( 'NONE', #15911, #11504, #21107 ) ;
#30185=ORIENTED_EDGE ( 'NONE', *, *, #19785, .T. ) ;
#30186=ORIENTED_EDGE ( 'NONE', *, *, #27698, .T. ) ;
#30212=DIRECTION ( 'NONE',  ( -1.881554647690000340E-09, 1.000000000000000000, 0.000000000000000000 ) ) ;
#30217=CARTESIAN_POINT ( 'NONE',  ( 0.2196031082797668954, -26.79904496338328812, 3.912378621952441016 ) ) ;
#30218=ORIENTED_EDGE ( 'NONE', *, *, #11703, .F. ) ;
#30221=ORIENTED_EDGE ( 'NONE', *, *, #12352, .T. ) ;
#30225=EDGE_CURVE ( 'NONE', #11948, #15558, #16243, .T. ) ;
#30233=CARTESIAN_POINT ( 'NONE',  ( -26.80000000000000071, 1.776356839399999804E-15, -2.842170943039999687E-14 ) ) ;
#30235=ORIENTED_EDGE ( 'NONE', *, *, #19030, .F. ) ;
#30236=AXIS2_PLACEMENT_3D ( 'NONE', #115, #271, #21664 ) ;
#30239=DIRECTION ( 'NONE',  ( 0.7071067811865475727, 0.7071067811865475727, 0.000000000000000000 ) ) ;
#30247=DIRECTION ( 'NONE',  ( 0.3633921898465291567, 0.9316362575375349842, -5.551115123125783333E-14 ) ) ;
#30252=EDGE_LOOP ( 'NONE', ( #30995, #513, #11035, #11338, #25070 ) ) ;
#30260=AXIS2_PLACEMENT_3D ( 'NONE', #12079, #21686, #9401 ) ;
#30261=CARTESIAN_POINT ( 'NONE',  ( -3.552713678799999608E-15, 0.000000000000000000, 93.60555127549999099 ) ) ;
#30276=CARTESIAN_POINT ( 'NONE',  ( -23.45268582408035485, -12.96920632950135754, 5.993195173463121250 ) ) ;
#30278=FACE_OUTER_BOUND ( 'NONE', #30666, .T. ) ;
#30280=CARTESIAN_POINT ( 'NONE',  ( 0.000000000000000000, 0.000000000000000000, -2.842170943039999687E-14 ) ) ;
#30283=AXIS2_PLACEMENT_3D ( 'NONE', #28233, #14235, #23995 ) ;
#30286=CARTESIAN_POINT ( 'NONE',  ( 0.000000000000000000, 0.000000000000000000, 115.0000000000000000 ) ) ;
#30290=ADVANCED_FACE ( 'NONE', ( #29593 ), #29344, .F. ) ;
#30307=ORIENTED_EDGE ( 'NONE', *, *, #19236, .T. ) ;
#30310=ORIENTED_EDGE ( 'NONE', *, *, #16635, .T. ) ;
#30324=AXIS2_PLACEMENT_3D ( 'NONE', #6636, #6331, #14043 ) ;
#30325=CARTESIAN_POINT ( 'NONE',  ( 24.49999999589999788, -3.000285566359999846E-15, 190.0000000000000000 ) ) ;
#30326=AXIS2_PLACEMENT_3D ( 'NONE', #31070, #9511, #16437 ) ;
#30331=CARTESIAN_POINT ( 'NONE',  ( -10.82908725742657730, -27.76276047461854191, 86.78285841159998881 ) ) ;
#30340=EDGE_LOOP ( 'NONE', ( #12450, #11269, #9598, #5416 ) ) ;
#30343=ORIENTED_EDGE ( 'NONE', *, *, #19157, .F. ) ;
#30348=CIRCLE ( 'NONE', #16767, 27.69999999999999929 ) ;
#30367=DIRECTION ( 'NONE',  ( 0.000000000000000000, 0.000000000000000000, 1.000000000000000000 ) ) ;
#30376=CIRCLE ( 'NONE', #9773, 4.000000004070001225 ) ;
#30377=CARTESIAN_POINT ( 'NONE',  ( 23.16113320640637241, -13.48374052559371350, 226.0999999999989143 ) ) ;
#30385=CARTESIAN_POINT ( 'NONE',  ( 1.100000000000000755, -26.77741585740001184, 4.902938919652013894 ) ) ;
#30389=EDGE_LOOP ( 'NONE', ( #2274, #8420, #19475, #6849 ) ) ;
#30396=VERTEX_POINT ( 'NONE', #14671 ) ;
#30397=TOROIDAL_SURFACE ( 'NONE', #14806, 24.50000000000000000, 4.000000000000000000 ) ;
#30401=FACE_OUTER_BOUND ( 'NONE', #14139, .T. ) ;
#30405=CARTESIAN_POINT ( 'NONE',  ( -18.95046173579999760, -18.95046173579999760, -2.842170943039999687E-14 ) ) ;
#30410=CIRCLE ( 'NONE', #14822, 26.80000000000000071 ) ;
#30415=CARTESIAN_POINT ( 'NONE',  ( 26.80000000000000071, 7.105427357599999217E-15, 0.000000000000000000 ) ) ;
#30422=FACE_OUTER_BOUND ( 'NONE', #14981, .T. ) ;
#30424=CIRCLE ( 'NONE', #16762, 27.92857142840000151 ) ;
#30426=EDGE_CURVE ( 'NONE', #28570, #16475, #20293, .T. ) ;
#30427=CARTESIAN_POINT ( 'NONE',  ( -26.11394584979204225, -6.088596733047862308, 93.21714158835003161 ) ) ;
#30429=ORIENTED_EDGE ( 'NONE', *, *, #4678, .F. ) ;
#30445=EDGE_LOOP ( 'NONE', ( #30096, #9243, #27395, #18647 ) ) ;
#30447=CARTESIAN_POINT ( 'NONE',  ( -22.63996212553987064, -14.34127312896723971, 225.1459679062982673 ) ) ;
#30456=CARTESIAN_POINT ( 'NONE',  ( 22.63992238019999803, -14.34133587289999845, 5.000000000000000000 ) ) ;
#30469=CARTESIAN_POINT ( 'NONE',  ( 27.76135143639999825, -3.399672735949999729E-15, 37.66141409829999986 ) ) ;
#30473=DIRECTION ( 'NONE',  ( 0.9316362575375349842, -0.3633921898465292122, 0.000000000000000000 ) ) ;
#30479=VERTEX_POINT ( 'NONE', #16900 ) ;
#30483=CARTESIAN_POINT ( 'NONE',  ( 27.54391552379999908, -3.373045395939999845E-15, 42.95625301639999805 ) ) ;
#30499=CARTESIAN_POINT ( 'NONE',  ( -23.70578532278555528, -13.93854223031271999, 6.087706803517302312 ) ) ;
#30507=ORIENTED_EDGE ( 'NONE', *, *, #2509, .T. ) ;
#30510=DIRECTION ( 'NONE',  ( -1.000000000000000000, 0.000000000000000000, 0.000000000000000000 ) ) ;
#30512=ADVANCED_FACE ( 'NONE', ( #26505 ), #19295, .F. ) ;
#30519=CARTESIAN_POINT ( 'NONE',  ( -18.95046173589999938, -18.95046173589999938, 230.0000000000000000 ) ) ;
#30533=CARTESIAN_POINT ( 'NONE',  ( -23.63627835177424075, -12.63201688151322699, 4.333923913749079482 ) ) ;
#30536=AXIS2_PLACEMENT_3D ( 'NONE', #12541, #22149, #27329 ) ;
#30537=CARTESIAN_POINT ( 'NONE',  ( 24.50000001620000134, -3.000285568839999855E-15, 189.9999999960000139 ) ) ;
#30544=CARTESIAN_POINT ( 'NONE',  ( 8.903108651239925564, -22.82508830966962421, 40.00000000000000000 ) ) ;
#30547=EDGE_LOOP ( 'NONE', ( #30066, #3320, #14524, #11844 ) ) ;
#30561=AXIS2_PLACEMENT_3D ( 'NONE', #27399, #24731, #13072 ) ;
#30566=CARTESIAN_POINT ( 'NONE',  ( 23.35113490838396189, -13.15228900088872521, 226.0721256962708878 ) ) ;
#30571=DIRECTION ( 'NONE',  ( 0.000000000000000000, 0.000000000000000000, 1.000000000000000000 ) ) ;
#30572=CARTESIAN_POINT ( 'NONE',  ( 0.000000000000000000, 0.000000000000000000, 0.000000000000000000 ) ) ;
#30575=DIRECTION ( 'NONE',  ( 0.000000000000000000, 0.000000000000000000, 1.000000000000000000 ) ) ;
#30589=AXIS2_PLACEMENT_3D ( 'NONE', #23604, #26419, #7059 ) ;
#30607=ORIENTED_EDGE ( 'NONE', *, *, #18793, .T. ) ;
#30613=CARTESIAN_POINT ( 'NONE',  ( 22.92405521622628939, -13.88330634250967144, 4.042547418791329505 ) ) ;
#30615=ADVANCED_FACE ( 'NONE', ( #16247 ), #9010, .T. ) ;
#30625=ORIENTED_EDGE ( 'NONE', *, *, #6230, .T. ) ;
#30626=DIRECTION ( 'NONE',  ( 0.000000000000000000, 0.000000000000000000, -1.000000000000000000 ) ) ;
#30635=AXIS2_PLACEMENT_3D ( 'NONE', #17495, #682, #5231 ) ;
#30649=EDGE_CURVE ( 'NONE', #4540, #24004, #23472, .T. ) ;
#30658=CARTESIAN_POINT ( 'NONE',  ( -9.993285220779425160, -25.61999708228226069, 27.99999999999999645 ) ) ;
#30664=ORIENTED_EDGE ( 'NONE', *, *, #25827, .F. ) ;
#30666=EDGE_LOOP ( 'NONE', ( #16112, #14350, #23617, #5218, #25274, #8372 ) ) ;
#30668=DIRECTION ( 'NONE',  ( 0.7071067811865475727, -0.7071067811865475727, 0.000000000000000000 ) ) ;
#30673=CARTESIAN_POINT ( 'NONE',  ( 27.92857142860000152, 3.552713678799999608E-15, 92.06031501460000754 ) ) ;
#30698=ORIENTED_EDGE ( 'NONE', *, *, #4464, .T. ) ;
#30711=ADVANCED_FACE ( 'NONE', ( #1316 ), #12283, .F. ) ;
#30714=CARTESIAN_POINT ( 'NONE',  ( 27.14999999970000033, -1.044534738649999915E-13, 0.000000000000000000 ) ) ;
#30715=CARTESIAN_POINT ( 'NONE',  ( -23.73988791507445484, -12.43614577693665879, 224.8540320935318846 ) ) ;
#30718=CARTESIAN_POINT ( 'NONE',  ( -10.14902473054660348, -26.01926976365539090, 187.9396849849999853 ) ) ;
#30720=B_SPLINE_CURVE_WITH_KNOTS ( 'NONE', 3,
 ( #25104, #1189, #20077, #8250, #24947, #22742, #25429, #25262, #3694, #3379 ),
 .UNSPECIFIED., .F., .F.,
 ( 4, 2, 2, 2, 4 ),
 ( 0.000000000000000000, 0.2500000000000000000, 0.5000000000000000000, 0.7500000000000000000, 1.000000000000000000 ),
 .UNSPECIFIED. ) ;
#30727=CARTESIAN_POINT ( 'NONE',  ( -8.903108651239966420, -22.82508830966961000, 190.0000000000000000 ) ) ;
#30734=ORIENTED_EDGE ( 'NONE', *, *, #27545, .F. ) ;
#30742=CARTESIAN_POINT ( 'NONE',  ( -0.2892544267695482674, -26.79878419693495317, 223.9285094851671261 ) ) ;
#30750=CARTESIAN_POINT ( 'NONE',  ( 27.23548387100000312, -3.552713678799999608E-15, 38.33953982530000104 ) ) ;
#30756=CARTESIAN_POINT ( 'NONE',  ( 9.594426947539483663, -25.77213547066686772, 25.40809952595784793 ) ) ;
#30757=ORIENTED_EDGE ( 'NONE', *, *, #5098, .F. ) ;
#30758=CARTESIAN_POINT ( 'NONE',  ( 22.69912944684746137, -14.24746549195691436, 4.513393846468806814 ) ) ;
#30760=DIRECTION ( 'NONE',  ( 1.000000000000000000, 0.000000000000000000, 0.000000000000000000 ) ) ;
#30762=EDGE_CURVE ( 'NONE', #24086, #10417, #11843, .T. ) ;
#30765=AXIS2_PLACEMENT_3D ( 'NONE', #19764, #22436, #10011 ) ;
#30771=EDGE_LOOP ( 'NONE', ( #12565, #15125, #28520, #10100, #18639, #25612 ) ) ;
#30772=LINE ( 'NONE', #21331, #26026 ) ;
#30777=B_SPLINE_CURVE_WITH_KNOTS ( 'NONE', 3,
 ( #18567, #1117, #3789, #13379, #1433, #15900, #25034, #29907, #11028, #20617, #8647, #25506 ),
 .UNSPECIFIED., .F., .F.,
 ( 4, 2, 2, 2, 2, 4 ),
 ( 0.000000000000000000, 0.2500000000000128786, 0.3750000000000193179, 0.5000000000000257572, 0.7500000000000128786, 1.000000000000000000 ),
 .UNSPECIFIED. ) ;
#30789=VERTEX_POINT ( 'NONE', #2405 ) ;
#30790=LINE ( 'NONE', #14422, #13475 ) ;
#30793=DIRECTION ( 'NONE',  ( 1.000000000000000000, 0.000000000000000000, 0.000000000000000000 ) ) ;
#30811=VERTEX_POINT ( 'NONE', #19232 ) ;
#30814=ORIENTED_EDGE ( 'NONE', *, *, #15559, .T. ) ;
#30839=VECTOR ( 'NONE', #28131, 1000.000000000000000 ) ;
#30843=AXIS2_PLACEMENT_3D ( 'NONE', #22880, #15626, #20983 ) ;
#30848=EDGE_LOOP ( 'NONE', ( #9613, #28925, #17706, #18470 ) ) ;
#30854=ADVANCED_FACE ( 'NONE', ( #3159 ), #12760, .F. ) ;
#30859=CARTESIAN_POINT ( 'NONE',  ( -10.82908725742657730, -27.76276047461854901, 36.78285841159999592 ) ) ;
#30865=DIRECTION ( 'NONE',  ( 1.000000000000000000, 0.000000000000000000, 0.000000000000000000 ) ) ;
#30866=CIRCLE ( 'NONE', #2230, 3.200000000000000178 ) ;
#30875=CARTESIAN_POINT ( 'NONE',  ( 0.000000000000000000, 0.000000000000000000, 43.60555127639999995 ) ) ;
#30876=DIRECTION ( 'NONE',  ( -0.000000000000000000, -0.000000000000000000, -1.000000000000000000 ) ) ;
#30888=CARTESIAN_POINT ( 'NONE',  ( -3.552713678799999608E-15, 0.000000000000000000, 143.2171415880000040 ) ) ;
#30889=DIRECTION ( 'NONE',  ( -0.3090169943750401549, -0.9510565162951233331, 0.000000000000000000 ) ) ;
#30890=CIRCLE ( 'NONE', #9260, 27.92857142860000152 ) ;
#30894=AXIS2_PLACEMENT_3D ( 'NONE', #15309, #5701, #24911 ) ;
#30896=CIRCLE ( 'NONE', #4689, 27.50000000000000000 ) ;
#30897=ORIENTED_EDGE ( 'NONE', *, *, #9235, .T. ) ;
#30903=DIRECTION ( 'NONE',  ( 0.000000000000000000, 0.000000000000000000, 1.000000000000000000 ) ) ;
#30905=VECTOR ( 'NONE', #27631, 1000.000000000000000 ) ;
#30915=CIRCLE ( 'NONE', #26399, 27.23548387080000310 ) ;
#30926=FACE_BOUND ( 'NONE', #10408, .T. ) ;
#30930=EDGE_CURVE ( 'NONE', #17294, #13677, #15734, .T. ) ;
#30945=ADVANCED_FACE ( 'NONE', ( #3465 ), #27804, .T. ) ;
#30948=CARTESIAN_POINT ( 'NONE',  ( -9.738910687886855655, -24.96785170200598714, 86.78285841159998881 ) ) ;
#30969=ORIENTED_EDGE ( 'NONE', *, *, #25565, .F. ) ;
#30974=ADVANCED_FACE ( 'NONE', ( #29132 ), #691, .T. ) ;
#30991=CARTESIAN_POINT ( 'NONE',  ( -23.67274795584174285, -12.56353887392313062, 4.451031837395022173 ) ) ;
#30994=DIRECTION ( 'NONE',  ( 1.000000000000000000, -1.224606353820000075E-16, 0.000000000000000000 ) ) ;
#30995=ORIENTED_EDGE ( 'NONE', *, *, #17385, .T. ) ;
#30997=CARTESIAN_POINT ( 'NONE',  ( -7.105427357599999217E-15, 0.000000000000000000, 86.78285841159998881 ) ) ;
#31000=CARTESIAN_POINT ( 'NONE',  ( 0.000000000000000000, 0.000000000000000000, 40.00000000000000000 ) ) ;
#31004=AXIS2_PLACEMENT_3D ( 'NONE', #9839, #14569, #568 ) ;
#31009=CARTESIAN_POINT ( 'NONE',  ( -2.664535259099999568E-14, -26.80000000000000071, 223.8999999999999773 ) ) ;
#31017=ORIENTED_EDGE ( 'NONE', *, *, #7371, .F. ) ;
#31021=DIRECTION ( 'NONE',  ( 0.5000000000001894040, 0.8660254037843291286, 0.000000000000000000 ) ) ;
#31025=CARTESIAN_POINT ( 'NONE',  ( -23.81569860410000317, -13.75000000000000000, 226.0999999999999943 ) ) ;
#31027=VECTOR ( 'NONE', #7850, 1000.000000000000000 ) ;
#31029=LINE ( 'NONE', #21125, #7171 ) ;
#31034=ORIENTED_EDGE ( 'NONE', *, *, #21179, .T. ) ;
#31035=EDGE_CURVE ( 'NONE', #20682, #5307, #18244, .T. ) ;
#31042=VERTEX_POINT ( 'NONE', #1279 ) ;
#31050=ORIENTED_EDGE ( 'NONE', *, *, #1416, .F. ) ;
#31052=TOROIDAL_SURFACE ( 'NONE', #30561, 24.50000000000000000, 4.000000000000000000 ) ;
#31062=CARTESIAN_POINT ( 'NONE',  ( 0.6483608293613253304, -27.49254329982320399, 5.909562041028879165 ) ) ;
#31066=CARTESIAN_POINT ( 'NONE',  ( 23.16094352345281138, -13.48406906521379334, 6.099999999996507327 ) ) ;
#31067=AXIS2_PLACEMENT_3D ( 'NONE', #15551, #3916, #18060 ) ;
#31070=CARTESIAN_POINT ( 'NONE',  ( 0.000000000000000000, 0.000000000000000000, 190.0000000000000000 ) ) ;
#31075=CIRCLE ( 'NONE', #17494, 3.000000000000001332 ) ;
#31077=DIRECTION ( 'NONE',  ( -1.000000000000000000, 1.224606353819999829E-16, 0.000000000000000000 ) ) ;
#31078=AXIS2_PLACEMENT_3D ( 'NONE', #9690, #9069, #9215 ) ;
#31084=DIRECTION ( 'NONE',  ( 0.000000000000000000, 0.000000000000000000, 1.000000000000000000 ) ) ;
#31090=CARTESIAN_POINT ( 'NONE',  ( -18.95046173579999760, -18.95046173579999760, 143.2171415880000040 ) ) ;
#31099=DIRECTION ( 'NONE',  ( -1.000000000000000000, 5.665498452320000818E-16, 0.000000000000000000 ) ) ;
#31107=FACE_OUTER_BOUND ( 'NONE', #9199, .T. ) ;
#31115=DIRECTION ( 'NONE',  ( -0.8090169943751909232, 0.5877852522921378498, 0.000000000000000000 ) ) ;
ENDSEC;
END-ISO-10303-21;
